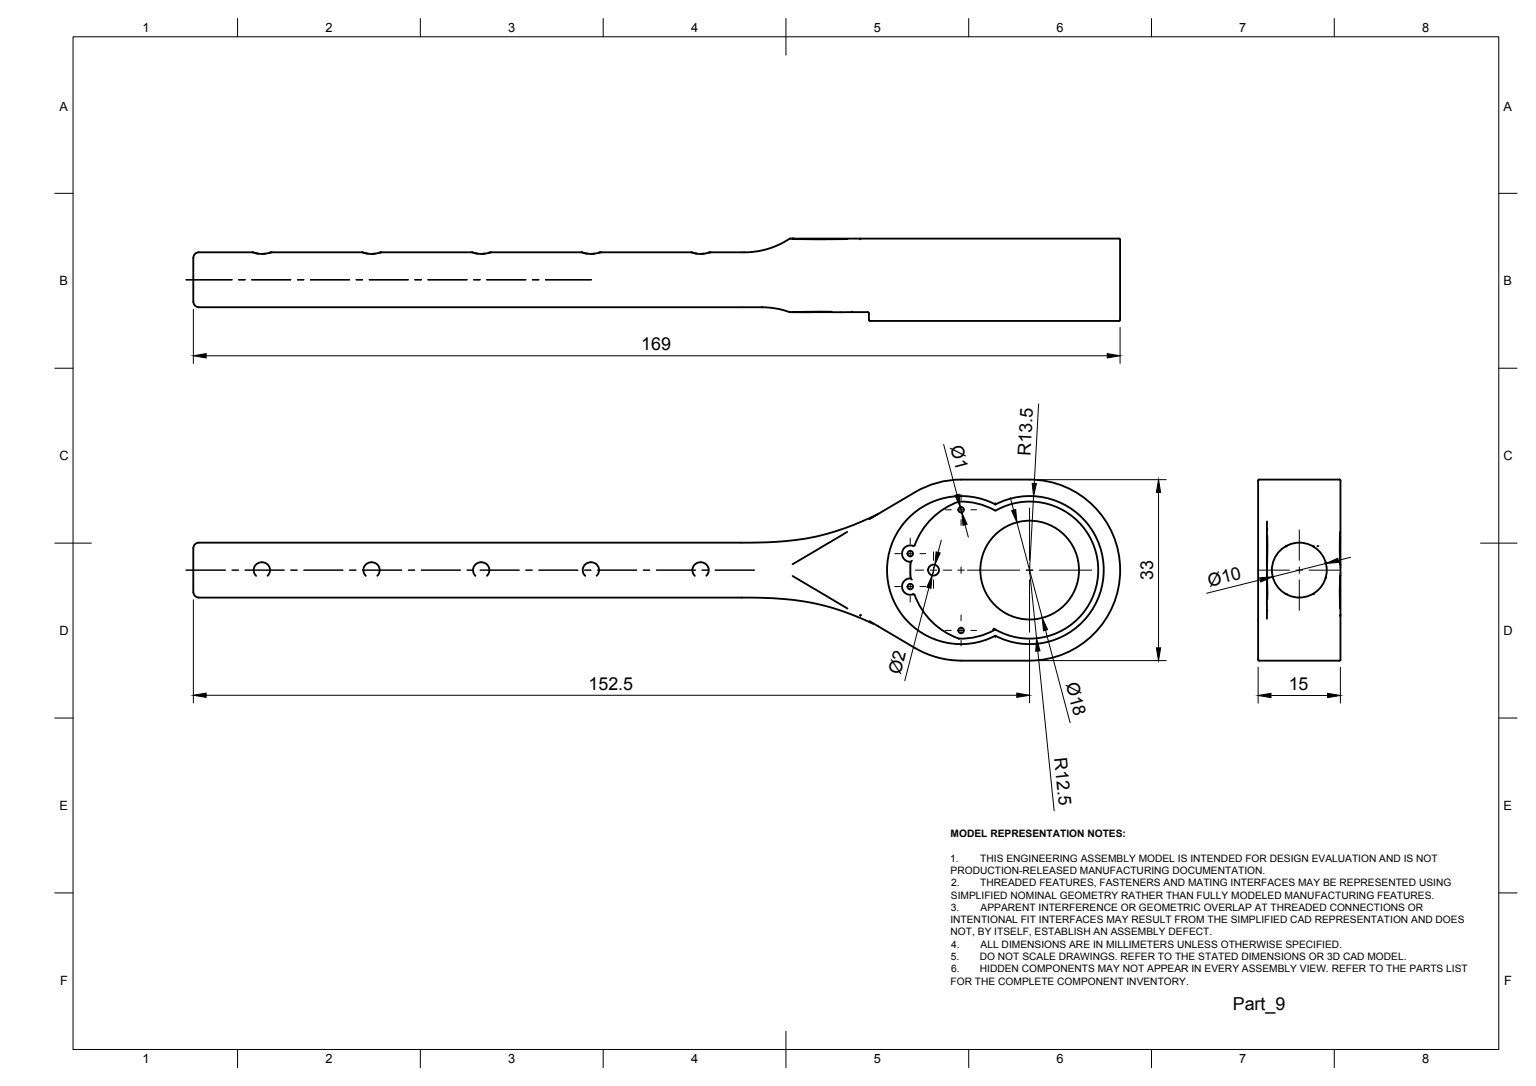
ISO-10303-21;
HEADER;
/* Generated by software containing ST-Developer
 * from STEP Tools, Inc. (www.steptools.com) 
 */

FILE_DESCRIPTION(
/* description */ ('STEP AP242 Edition 2'),
/* implementation_level */ '2;1');

FILE_NAME(
/* name */ 'Part_9.step',
/* time_stamp */ '2026-10-06T10:11:12-07:00',
/* author */ (''),
/* organization */ (''),
/* preprocessor_version */ 'ST-DEVELOPER v20.2',
/* originating_system */ 'Autodesk Translation Framework v15.15.0.0',
/* authorisation */ '');

FILE_SCHEMA (('AUTOMOTIVE_DESIGN { 1 0 10303 214 3 1 1 }'));
ENDSEC;

DATA;
#10=MECHANICAL_DESIGN_GEOMETRIC_PRESENTATION_REPRESENTATION('',(#1799),#54580);
#124=ELLIPSE('',#19386,0.00047049920898836,0.0004);
#125=ELLIPSE('',#19388,0.00047049920898836,0.0004);
#126=ELLIPSE('',#19445,0.000286242347628646,0.000206247332886668);
#127=ELLIPSE('',#19470,0.000318385781181688,0.0002);
#128=ELLIPSE('',#19492,0.000318385781181688,0.0002);
#129=ELLIPSE('',#19548,0.00200013961276074,0.00200000211919392);
#130=ELLIPSE('',#19569,0.00200131676890062,0.00200065811979615);
#160=SPHERICAL_SURFACE('',#19391,0.0015);
#161=SPHERICAL_SURFACE('',#19392,0.0015);
#162=SPHERICAL_SURFACE('',#19393,0.0015);
#163=SPHERICAL_SURFACE('',#19394,0.0015);
#164=SPHERICAL_SURFACE('',#19395,0.0015);
#165=SPHERICAL_SURFACE('',#19475,0.0002);
#166=SPHERICAL_SURFACE('',#19500,0.0002);
#167=SPHERICAL_SURFACE('',#19532,0.0002);
#168=SPHERICAL_SURFACE('',#19537,0.0002);
#169=SPHERICAL_SURFACE('',#19539,0.0002);
#283=TOROIDAL_SURFACE('',#19417,0.0723798046062635,0.0693846505577955);
#284=TOROIDAL_SURFACE('',#19418,0.0725493479148083,0.0695588361081736);
#285=TOROIDAL_SURFACE('',#19419,0.0729629625245639,0.0699799856940105);
#286=TOROIDAL_SURFACE('',#19420,0.0719744531392773,0.0689794249020661);
#287=TOROIDAL_SURFACE('',#19421,0.0127,0.0002);
#288=TOROIDAL_SURFACE('',#19424,0.0004,0.0002);
#289=TOROIDAL_SURFACE('',#19429,0.0134323601801219,0.0002);
#290=TOROIDAL_SURFACE('',#19430,0.0130323601801219,0.0002);
#291=TOROIDAL_SURFACE('',#19435,0.0004,0.0002);
#292=TOROIDAL_SURFACE('',#19437,0.0013,0.0002);
#293=TOROIDAL_SURFACE('',#19438,0.0130323601801219,0.0002);
#294=TOROIDAL_SURFACE('',#19439,0.0013,0.0002);
#295=TOROIDAL_SURFACE('',#19441,0.0004,0.0002);
#296=TOROIDAL_SURFACE('',#19444,0.0130323601801219,0.0002);
#297=TOROIDAL_SURFACE('',#19449,0.0134323601801219,0.0002);
#298=TOROIDAL_SURFACE('',#19451,0.0004,0.0002);
#299=TOROIDAL_SURFACE('',#19453,0.0127,0.0002);
#300=TOROIDAL_SURFACE('',#19456,0.0163,0.0002);
#301=TOROIDAL_SURFACE('',#19461,1.2311209928723,1.23094461923187);
#302=TOROIDAL_SURFACE('',#19471,0.00114036081014246,0.000200479570708582);
#303=TOROIDAL_SURFACE('',#19473,0.0163,0.0002);
#304=TOROIDAL_SURFACE('',#19479,1.19654575499128,1.19636811754444);
#305=TOROIDAL_SURFACE('',#19485,0.0023,0.0002);
#306=TOROIDAL_SURFACE('',#19487,0.0163,0.0002);
#307=TOROIDAL_SURFACE('',#19489,0.0027,0.0002);
#308=TOROIDAL_SURFACE('',#19503,0.0123,0.0002);
#309=TOROIDAL_SURFACE('',#19506,0.0092,0.0002);
#310=TOROIDAL_SURFACE('',#19512,0.0163,0.0002);
#311=TOROIDAL_SURFACE('',#19514,0.00109148741098655,0.000200226016163471);
#312=TOROIDAL_SURFACE('',#19519,0.0163,0.0002);
#313=TOROIDAL_SURFACE('',#19525,0.0163,0.0002);
#314=TOROIDAL_SURFACE('',#19526,0.0137,0.0002);
#315=TOROIDAL_SURFACE('',#19527,0.0137,0.0002);
#316=TOROIDAL_SURFACE('',#19528,0.0092,0.0002);
#317=TOROIDAL_SURFACE('',#19530,0.0012,0.0002);
#318=TOROIDAL_SURFACE('',#19534,0.0127,0.0002);
#319=TOROIDAL_SURFACE('',#19543,0.0123,0.0002);
#320=TOROIDAL_SURFACE('',#19546,0.0127,0.0002);
#321=TOROIDAL_SURFACE('',#19547,0.0021940391762114,0.00199286501744214);
#322=TOROIDAL_SURFACE('',#19575,0.004,0.001);
#337=B_SPLINE_SURFACE_WITH_KNOTS('',3,3,((#50042,#50043,#50044,#50045),
(#50046,#50047,#50048,#50049),(#50050,#50051,#50052,#50053),(#50054,#50055,
#50056,#50057),(#50058,#50059,#50060,#50061),(#50062,#50063,#50064,#50065),
(#50066,#50067,#50068,#50069)),.UNSPECIFIED.,.F.,.F.,.F.,(4,1,1,1,4),(4,
4),(0.581678330580955,0.66570223965942,0.749726148737884,0.833750057816349,
0.917773966894813),(0.,0.272096154167828),.UNSPECIFIED.);
#338=B_SPLINE_SURFACE_WITH_KNOTS('',3,3,((#50328,#50329,#50330,#50331),
(#50332,#50333,#50334,#50335),(#50336,#50337,#50338,#50339),(#50340,#50341,
#50342,#50343),(#50344,#50345,#50346,#50347),(#50348,#50349,#50350,#50351),
(#50352,#50353,#50354,#50355)),.UNSPECIFIED.,.F.,.F.,.F.,(4,1,1,1,4),(4,
4),(0.082398587787618,0.16607539724211,0.249752206696602,0.333429016151093,
0.417105825605585),(0.,0.340678729399104),.UNSPECIFIED.);
#339=B_SPLINE_SURFACE_WITH_KNOTS('',3,3,((#50620,#50621,#50622,#50623),
(#50624,#50625,#50626,#50627),(#50628,#50629,#50630,#50631),(#50632,#50633,
#50634,#50635),(#50636,#50637,#50638,#50639),(#50640,#50641,#50642,#50643),
(#50644,#50645,#50646,#50647),(#50648,#50649,#50650,#50651),(#50652,#50653,
#50654,#50655),(#50656,#50657,#50658,#50659)),.UNSPECIFIED.,.F.,.F.,.F.,
(4,3,1,1,1,4),(4,4),(0.88386669972742,0.917773966894813,0.93833047517111,
0.958886983447406,0.979443491723703,1.),(0.,1.),.UNSPECIFIED.);
#340=B_SPLINE_SURFACE_WITH_KNOTS('',3,3,((#50859,#50860,#50861,#50862),
(#50863,#50864,#50865,#50866),(#50867,#50868,#50869,#50870),(#50871,#50872,
#50873,#50874),(#50875,#50876,#50877,#50878),(#50879,#50880,#50881,#50882),
(#50883,#50884,#50885,#50886),(#50887,#50888,#50889,#50890),(#50891,#50892,
#50893,#50894),(#50895,#50896,#50897,#50898),(#50899,#50900,#50901,#50902),
(#50903,#50904,#50905,#50906),(#50907,#50908,#50909,#50910),(#50911,#50912,
#50913,#50914),(#50915,#50916,#50917,#50918),(#50919,#50920,#50921,#50922),
(#50923,#50924,#50925,#50926),(#50927,#50928,#50929,#50930)),
 .UNSPECIFIED.,.F.,.F.,.F.,(4,3,1,1,1,2,1,1,1,3,4),(4,4),(0.414454525410024,
0.417105825605585,0.437698866011632,0.45829190641768,0.478884946823728,
0.499477987229775,0.52002807306757,0.540578158905365,0.56112824474316,0.581678330580955,
0.616449456714453),(0.,1.),.UNSPECIFIED.);
#341=B_SPLINE_SURFACE_WITH_KNOTS('',3,3,((#51085,#51086,#51087,#51088),
(#51089,#51090,#51091,#51092),(#51093,#51094,#51095,#51096),(#51097,#51098,
#51099,#51100),(#51101,#51102,#51103,#51104),(#51105,#51106,#51107,#51108),
(#51109,#51110,#51111,#51112),(#51113,#51114,#51115,#51116),(#51117,#51118,
#51119,#51120),(#51121,#51122,#51123,#51124)),.UNSPECIFIED.,.F.,.F.,.F.,
(4,1,1,1,3,4),(4,4),(0.,0.0205996469469045,0.041199293893809,0.0617989408407135,
0.082398587787618,0.082892979314345),(0.,1.),.UNSPECIFIED.);
#342=B_SPLINE_SURFACE_WITH_KNOTS('',3,3,((#53343,#53344,#53345,#53346),
(#53347,#53348,#53349,#53350),(#53351,#53352,#53353,#53354),(#53355,#53356,
#53357,#53358),(#53359,#53360,#53361,#53362),(#53363,#53364,#53365,#53366),
(#53367,#53368,#53369,#53370),(#53371,#53372,#53373,#53374),(#53375,#53376,
#53377,#53378),(#53379,#53380,#53381,#53382),(#53383,#53384,#53385,#53386)),
 .UNSPECIFIED.,.F.,.F.,.F.,(4,1,1,1,1,1,1,1,4),(4,4),(-0.00100716856165045,
0.00254911418953192,0.00509822837906388,0.00764734256859584,0.0101964567581278,
0.0127455709476598,0.0152946851371917,0.0178437993267237,0.0213314374719094),
(0.,1.00749523383058),.UNSPECIFIED.);
#1362=B_SPLINE_CURVE_WITH_KNOTS('',3,(#49171,#49172,#49173,#49174,#49175,
#49176,#49177,#49178,#49179,#49180,#49181),.UNSPECIFIED.,.F.,.F.,(4,1,1,
1,1,1,1,1,4),(2.16840434497101E-19,0.00133638350122092,0.00267276700244183,
0.00400915050366275,0.00534553400488367,0.00668191750610458,0.0080183010073255,
0.00935468450854642,0.0106661079505718),.UNSPECIFIED.);
#1363=B_SPLINE_CURVE_WITH_KNOTS('',3,(#49187,#49188,#49189,#49190),
 .UNSPECIFIED.,.F.,.F.,(4,4),(0.0082109079468729,0.00936873648796082),
 .UNSPECIFIED.);
#1364=B_SPLINE_CURVE_WITH_KNOTS('',3,(#49192,#49193,#49194,#49195,#49196),
 .UNSPECIFIED.,.F.,.F.,(4,1,4),(0.00704598836791066,0.00819764442696572,
0.0082109079468729),.UNSPECIFIED.);
#1365=B_SPLINE_CURVE_WITH_KNOTS('',3,(#49198,#49199,#49200,#49201,#49202),
 .UNSPECIFIED.,.F.,.F.,(4,1,4),(0.00585546030497552,0.00702655236597062,
0.00704598836791066),.UNSPECIFIED.);
#1366=B_SPLINE_CURVE_WITH_KNOTS('',3,(#49204,#49205,#49206,#49207,#49208),
 .UNSPECIFIED.,.F.,.F.,(4,1,4),(0.00352617550117164,0.00468436824398041,
0.00585546030497552),.UNSPECIFIED.);
#1367=B_SPLINE_CURVE_WITH_KNOTS('',3,(#49210,#49211,#49212,#49213,#49214),
 .UNSPECIFIED.,.F.,.F.,(4,1,4),(0.00236041305988056,0.00351327618298531,
0.00352617550117164),.UNSPECIFIED.);
#1368=B_SPLINE_CURVE_WITH_KNOTS('',3,(#49216,#49217,#49218,#49219,#49220),
 .UNSPECIFIED.,.F.,.F.,(4,1,4),(0.0011710920609951,0.00234218412199021,
0.00236041305988056),.UNSPECIFIED.);
#1369=B_SPLINE_CURVE_WITH_KNOTS('',3,(#49221,#49222,#49223,#49224),
 .UNSPECIFIED.,.F.,.F.,(4,4),(2.22095063237474E-5,0.0011710920609951),
 .UNSPECIFIED.);
#1370=B_SPLINE_CURVE_WITH_KNOTS('',3,(#49264,#49265,#49266,#49267,#49268,
#49269,#49270,#49271,#49272,#49273,#49274),.UNSPECIFIED.,.F.,.F.,(4,1,1,
1,1,1,1,1,4),(2.16840434497101E-19,0.00133638350122092,0.00267276700244184,
0.00400915050366276,0.00534553400488369,0.00668191750610461,0.00801830100732553,
0.00935468450854645,0.0106661079505719),.UNSPECIFIED.);
#1371=B_SPLINE_CURVE_WITH_KNOTS('',3,(#49280,#49281,#49282,#49283),
 .UNSPECIFIED.,.F.,.F.,(4,4),(0.00821090794687196,0.00936873648796082),
 .UNSPECIFIED.);
#1372=B_SPLINE_CURVE_WITH_KNOTS('',3,(#49285,#49286,#49287,#49288,#49289),
 .UNSPECIFIED.,.F.,.F.,(4,1,4),(0.00704598836790975,0.00819764442696572,
0.00821090794687196),.UNSPECIFIED.);
#1373=B_SPLINE_CURVE_WITH_KNOTS('',3,(#49291,#49292,#49293,#49294,#49295),
 .UNSPECIFIED.,.F.,.F.,(4,1,4),(0.00585546030497551,0.00702655236597062,
0.00704598836790975),.UNSPECIFIED.);
#1374=B_SPLINE_CURVE_WITH_KNOTS('',3,(#49297,#49298,#49299,#49300,#49301),
 .UNSPECIFIED.,.F.,.F.,(4,1,4),(0.00352617550117226,0.00468436824398041,
0.00585546030497551),.UNSPECIFIED.);
#1375=B_SPLINE_CURVE_WITH_KNOTS('',3,(#49303,#49304,#49305,#49306,#49307),
 .UNSPECIFIED.,.F.,.F.,(4,1,4),(0.00236041305988015,0.00351327618298531,
0.00352617550117226),.UNSPECIFIED.);
#1376=B_SPLINE_CURVE_WITH_KNOTS('',3,(#49309,#49310,#49311,#49312,#49313),
 .UNSPECIFIED.,.F.,.F.,(4,1,4),(0.0011710920609951,0.00234218412199021,
0.00236041305988015),.UNSPECIFIED.);
#1377=B_SPLINE_CURVE_WITH_KNOTS('',3,(#49314,#49315,#49316,#49317),
 .UNSPECIFIED.,.F.,.F.,(4,4),(2.22095063236846E-5,0.0011710920609951),
 .UNSPECIFIED.);
#1378=B_SPLINE_CURVE_WITH_KNOTS('',3,(#49357,#49358,#49359,#49360,#49361,
#49362,#49363,#49364,#49365,#49366,#49367),.UNSPECIFIED.,.F.,.F.,(4,1,1,
1,1,1,1,1,4),(2.16840434497101E-19,0.00133638350122092,0.00267276700244184,
0.00400915050366277,0.00534553400488369,0.00668191750610461,0.00801830100732553,
0.00935468450854646,0.0106661079505718),.UNSPECIFIED.);
#1379=B_SPLINE_CURVE_WITH_KNOTS('',3,(#49373,#49374,#49375,#49376),
 .UNSPECIFIED.,.F.,.F.,(4,4),(0.00821090794687294,0.00936873648796081),
 .UNSPECIFIED.);
#1380=B_SPLINE_CURVE_WITH_KNOTS('',3,(#49378,#49379,#49380,#49381,#49382),
 .UNSPECIFIED.,.F.,.F.,(4,1,4),(0.00704598836791145,0.00819764442696571,
0.00821090794687294),.UNSPECIFIED.);
#1381=B_SPLINE_CURVE_WITH_KNOTS('',3,(#49384,#49385,#49386,#49387,#49388),
 .UNSPECIFIED.,.F.,.F.,(4,1,4),(0.00585546030497551,0.00702655236597061,
0.00704598836791145),.UNSPECIFIED.);
#1382=B_SPLINE_CURVE_WITH_KNOTS('',3,(#49390,#49391,#49392,#49393,#49394),
 .UNSPECIFIED.,.F.,.F.,(4,1,4),(0.00352617550117169,0.00468436824398041,
0.00585546030497551),.UNSPECIFIED.);
#1383=B_SPLINE_CURVE_WITH_KNOTS('',3,(#49396,#49397,#49398,#49399,#49400),
 .UNSPECIFIED.,.F.,.F.,(4,1,4),(0.00236041305987884,0.00351327618298531,
0.00352617550117169),.UNSPECIFIED.);
#1384=B_SPLINE_CURVE_WITH_KNOTS('',3,(#49402,#49403,#49404,#49405,#49406),
 .UNSPECIFIED.,.F.,.F.,(4,1,4),(0.0011710920609951,0.0023421841219902,0.00236041305987884),
 .UNSPECIFIED.);
#1385=B_SPLINE_CURVE_WITH_KNOTS('',3,(#49407,#49408,#49409,#49410),
 .UNSPECIFIED.,.F.,.F.,(4,4),(2.2209506323702E-5,0.0011710920609951),
 .UNSPECIFIED.);
#1386=B_SPLINE_CURVE_WITH_KNOTS('',3,(#49450,#49451,#49452,#49453,#49454,
#49455,#49456,#49457,#49458,#49459,#49460),.UNSPECIFIED.,.F.,.F.,(4,1,1,
1,1,1,1,1,4),(2.16840434497101E-19,0.00133638350122092,0.00267276700244185,
0.00400915050366277,0.0053455340048837,0.00668191750610462,0.00801830100732555,
0.00935468450854647,0.0106661079505723),.UNSPECIFIED.);
#1387=B_SPLINE_CURVE_WITH_KNOTS('',3,(#49466,#49467,#49468,#49469),
 .UNSPECIFIED.,.F.,.F.,(4,4),(0.00821090794688191,0.00936873648796083),
 .UNSPECIFIED.);
#1388=B_SPLINE_CURVE_WITH_KNOTS('',3,(#49471,#49472,#49473,#49474,#49475),
 .UNSPECIFIED.,.F.,.F.,(4,1,4),(0.00704598836790659,0.00819764442696573,
0.00821090794688191),.UNSPECIFIED.);
#1389=B_SPLINE_CURVE_WITH_KNOTS('',3,(#49477,#49478,#49479,#49480,#49481),
 .UNSPECIFIED.,.F.,.F.,(4,1,4),(0.00585546030497552,0.00702655236597062,
0.00704598836790659),.UNSPECIFIED.);
#1390=B_SPLINE_CURVE_WITH_KNOTS('',3,(#49483,#49484,#49485,#49486,#49487),
 .UNSPECIFIED.,.F.,.F.,(4,1,4),(0.00352617550117701,0.00468436824398042,
0.00585546030497552),.UNSPECIFIED.);
#1391=B_SPLINE_CURVE_WITH_KNOTS('',3,(#49489,#49490,#49491,#49492,#49493),
 .UNSPECIFIED.,.F.,.F.,(4,1,4),(0.00236041305988171,0.00351327618298531,
0.00352617550117701),.UNSPECIFIED.);
#1392=B_SPLINE_CURVE_WITH_KNOTS('',3,(#49495,#49496,#49497,#49498,#49499),
 .UNSPECIFIED.,.F.,.F.,(4,1,4),(0.0011710920609951,0.00234218412199021,
0.00236041305988171),.UNSPECIFIED.);
#1393=B_SPLINE_CURVE_WITH_KNOTS('',3,(#49500,#49501,#49502,#49503),
 .UNSPECIFIED.,.F.,.F.,(4,4),(2.22095063237639E-5,0.0011710920609951),
 .UNSPECIFIED.);
#1394=B_SPLINE_CURVE_WITH_KNOTS('',3,(#49543,#49544,#49545,#49546,#49547,
#49548,#49549,#49550,#49551,#49552,#49553),.UNSPECIFIED.,.F.,.F.,(4,1,1,
1,1,1,1,1,4),(2.16840434497101E-19,0.00133638350122091,0.00267276700244182,
0.00400915050366274,0.00534553400488365,0.00668191750610456,0.00801830100732547,
0.00935468450854638,0.0106661079505722),.UNSPECIFIED.);
#1395=B_SPLINE_CURVE_WITH_KNOTS('',3,(#49559,#49560,#49561,#49562),
 .UNSPECIFIED.,.F.,.F.,(4,4),(0.00821090794688314,0.00936873648796083),
 .UNSPECIFIED.);
#1396=B_SPLINE_CURVE_WITH_KNOTS('',3,(#49564,#49565,#49566,#49567,#49568),
 .UNSPECIFIED.,.F.,.F.,(4,1,4),(0.00704598836790498,0.00819764442696573,
0.00821090794688314),.UNSPECIFIED.);
#1397=B_SPLINE_CURVE_WITH_KNOTS('',3,(#49570,#49571,#49572,#49573,#49574),
 .UNSPECIFIED.,.F.,.F.,(4,1,4),(0.00585546030497552,0.00702655236597062,
0.00704598836790498),.UNSPECIFIED.);
#1398=B_SPLINE_CURVE_WITH_KNOTS('',3,(#49576,#49577,#49578,#49579,#49580),
 .UNSPECIFIED.,.F.,.F.,(4,1,4),(0.0035261755011782,0.00468436824398041,
0.00585546030497552),.UNSPECIFIED.);
#1399=B_SPLINE_CURVE_WITH_KNOTS('',3,(#49582,#49583,#49584,#49585,#49586),
 .UNSPECIFIED.,.F.,.F.,(4,1,4),(0.00236041305988064,0.00351327618298531,
0.0035261755011782),.UNSPECIFIED.);
#1400=B_SPLINE_CURVE_WITH_KNOTS('',3,(#49588,#49589,#49590,#49591,#49592),
 .UNSPECIFIED.,.F.,.F.,(4,1,4),(0.0011710920609951,0.00234218412199021,
0.00236041305988064),.UNSPECIFIED.);
#1401=B_SPLINE_CURVE_WITH_KNOTS('',3,(#49593,#49594,#49595,#49596),
 .UNSPECIFIED.,.F.,.F.,(4,4),(2.2209506323727E-5,0.0011710920609951),
 .UNSPECIFIED.);
#1402=B_SPLINE_CURVE_WITH_KNOTS('',3,(#49600,#49601,#49602,#49603),
 .UNSPECIFIED.,.F.,.F.,(4,4),(0.,0.000682262674512534),.UNSPECIFIED.);
#1403=B_SPLINE_CURVE_WITH_KNOTS('',3,(#49668,#49669,#49670,#49671,#49672,
#49673),.UNSPECIFIED.,.F.,.F.,(4,2,4),(-0.101895978906481,-0.0984710269726971,
-0.0896897186466305),.UNSPECIFIED.);
#1404=B_SPLINE_CURVE_WITH_KNOTS('',3,(#49680,#49681,#49682,#49683,#49684,
#49685,#49686,#49687,#49688,#49689),.UNSPECIFIED.,.F.,.F.,(4,2,2,2,4),(0.00701311257563557,
0.010982820742087,0.0253526872842843,0.0698643291505208,0.0772205186033042),
 .UNSPECIFIED.);
#1405=B_SPLINE_CURVE_WITH_KNOTS('',3,(#49702,#49703,#49704,#49705,#49706,
#49707,#49708,#49709,#49710,#49711,#49712,#49713,#49714),.UNSPECIFIED.,
 .F.,.F.,(4,3,3,3,4),(0.0824582419012307,0.166224116038678,0.249986773069777,
0.333749430179514,0.417515304238324),.UNSPECIFIED.);
#1406=B_SPLINE_CURVE_WITH_KNOTS('',3,(#49720,#49721,#49722,#49723,#49724,
#49725,#49726,#49727,#49728,#49729,#49730,#49731,#49732),.UNSPECIFIED.,
 .F.,.F.,(4,3,3,3,4),(0.582140268332509,0.666078166051184,0.750012831472539,
0.833947496910044,0.91788539461257),.UNSPECIFIED.);
#1407=B_SPLINE_CURVE_WITH_KNOTS('',3,(#49741,#49742,#49743,#49744),
 .UNSPECIFIED.,.F.,.F.,(4,4),(0.0106661079505722,0.0106910680097673),
 .UNSPECIFIED.);
#1408=B_SPLINE_CURVE_WITH_KNOTS('',3,(#49745,#49746,#49747,#49748),
 .UNSPECIFIED.,.F.,.F.,(4,4),(0.0106661079505723,0.0106910680097674),
 .UNSPECIFIED.);
#1409=B_SPLINE_CURVE_WITH_KNOTS('',3,(#49749,#49750,#49751,#49752),
 .UNSPECIFIED.,.F.,.F.,(4,4),(0.0106661079505718,0.0106910680097674),
 .UNSPECIFIED.);
#1410=B_SPLINE_CURVE_WITH_KNOTS('',3,(#49753,#49754,#49755,#49756),
 .UNSPECIFIED.,.F.,.F.,(4,4),(0.0106661079505719,0.0106910680097674),
 .UNSPECIFIED.);
#1411=B_SPLINE_CURVE_WITH_KNOTS('',3,(#49757,#49758,#49759,#49760),
 .UNSPECIFIED.,.F.,.F.,(4,4),(0.0106661079505718,0.0106910680097673),
 .UNSPECIFIED.);
#1412=B_SPLINE_CURVE_WITH_KNOTS('',3,(#49824,#49825,#49826,#49827,#49828,
#49829,#49830),.UNSPECIFIED.,.F.,.F.,(4,3,4),(2.16840434497101E-19,0.00581319522920539,
0.0116263904584108),.UNSPECIFIED.);
#1413=B_SPLINE_CURVE_WITH_KNOTS('',3,(#49832,#49833,#49834,#49835),
 .UNSPECIFIED.,.F.,.F.,(4,4),(2.79715755706988E-17,0.00267897349074099),
 .UNSPECIFIED.);
#1414=B_SPLINE_CURVE_WITH_KNOTS('',3,(#49851,#49852,#49853,#49854),
 .UNSPECIFIED.,.F.,.F.,(4,4),(3.43963882861591E-14,0.0026798705859963),
 .UNSPECIFIED.);
#1415=B_SPLINE_CURVE_WITH_KNOTS('',3,(#49856,#49857,#49858,#49859,#49860,
#49861,#49862),.UNSPECIFIED.,.F.,.F.,(4,3,4),(0.0153783179950603,0.0211672261179413,
0.0269561342408223),.UNSPECIFIED.);
#1416=B_SPLINE_CURVE_WITH_KNOTS('',3,(#49863,#49864,#49865,#49866,#49867,
#49868,#49869,#49870,#49871,#49872,#49873,#49874,#49875),.UNSPECIFIED.,
 .F.,.F.,(4,3,3,3,4),(1.62471150819444E-9,0.371962494639839,0.5,0.868119627457051,
0.999999997610495),.UNSPECIFIED.);
#1417=B_SPLINE_CURVE_WITH_KNOTS('',3,(#49934,#49935,#49936,#49937,#49938,
#49939,#49940,#49941,#49942,#49943,#49944,#49945,#49946,#49947,#49948,#49949),
 .UNSPECIFIED.,.F.,.F.,(4,3,3,3,3,4),(1.63653485417008E-17,0.000871734875690096,
0.00174346975138018,0.00261520462707026,0.0030510720649153,0.00348693950276033),
 .UNSPECIFIED.);
#1418=B_SPLINE_CURVE_WITH_KNOTS('',3,(#49951,#49952,#49953,#49954,#49955,
#49956,#49957,#49958,#49959,#49960,#49961,#49962,#49963,#49964,#49965,#49966),
 .UNSPECIFIED.,.F.,.F.,(4,3,3,3,3,4),(0.,0.25,0.375,0.5,0.75,1.),
 .UNSPECIFIED.);
#1419=B_SPLINE_CURVE_WITH_KNOTS('',3,(#49970,#49971,#49972,#49973,#49974,
#49975,#49976,#49977,#49978,#49979,#49980,#49981,#49982),.UNSPECIFIED.,
 .F.,.F.,(4,3,3,3,4),(3.26962013452912E-17,0.000593256852872857,0.00118651370574568,
0.00177977055861851,0.00237302741149133),.UNSPECIFIED.);
#1420=B_SPLINE_CURVE_WITH_KNOTS('',3,(#49993,#49994,#49995,#49996,#49997,
#49998,#49999,#50000,#50001,#50002,#50003,#50004,#50005),.UNSPECIFIED.,
 .F.,.F.,(4,3,3,3,4),(1.56949960400744E-16,0.000586676321783765,0.00117335264356737,
0.00176002896535098,0.00234670528713459),.UNSPECIFIED.);
#1421=B_SPLINE_CURVE_WITH_KNOTS('',3,(#50009,#50010,#50011,#50012),
 .UNSPECIFIED.,.F.,.F.,(4,4),(0.,1.),.UNSPECIFIED.);
#1422=B_SPLINE_CURVE_WITH_KNOTS('',3,(#50014,#50015,#50016,#50017),
 .UNSPECIFIED.,.F.,.F.,(4,4),(0.,1.),.UNSPECIFIED.);
#1423=B_SPLINE_CURVE_WITH_KNOTS('',3,(#50019,#50020,#50021,#50022,#50023,
#50024,#50025,#50026,#50027,#50028,#50029,#50030,#50031,#50032,#50033,#50034),
 .UNSPECIFIED.,.F.,.F.,(4,3,3,3,3,4),(1.23884035470014E-17,0.000436227682635904,
0.000872455365271796,0.00174491073054358,0.00261736609581536,0.00348982146108715),
 .UNSPECIFIED.);
#1424=B_SPLINE_CURVE_WITH_KNOTS('',3,(#50071,#50072,#50073,#50074,#50075,
#50076,#50077,#50078,#50079,#50080),.UNSPECIFIED.,.F.,.F.,(4,3,3,4),(0.,
0.250198742533901,0.484142189377901,0.72625720196945),.UNSPECIFIED.);
#1425=B_SPLINE_CURVE_WITH_KNOTS('',3,(#50082,#50083,#50084,#50085,#50086,
#50087,#50088,#50089,#50090,#50091,#50092,#50093,#50094,#50095,#50096,#50097,
#50098,#50099,#50100,#50101,#50102,#50103,#50104,#50105,#50106,#50107,#50108,
#50109,#50110,#50111,#50112,#50113,#50114,#50115,#50116,#50117,#50118,#50119,
#50120,#50121,#50122,#50123,#50124,#50125,#50126,#50127,#50128,#50129,#50130,
#50131,#50132,#50133,#50134,#50135,#50136),.UNSPECIFIED.,.F.,.F.,(4,3,3,
3,3,3,3,3,3,3,3,3,3,3,3,3,3,3,4),(2.6220077343514E-7,0.0203152518413343,
0.134046967430369,0.239869415550571,0.25,0.339303542480863,0.375,0.5,0.523390970218302,
0.625,0.6875,0.69519800169401,0.71875,0.75,0.78125,0.8125,0.875,0.884458267348107,
1.),.UNSPECIFIED.);
#1426=B_SPLINE_CURVE_WITH_KNOTS('',3,(#50138,#50139,#50140,#50141,#50142,
#50143,#50144,#50145,#50146,#50147,#50148,#50149,#50150,#50151,#50152,#50153,
#50154,#50155,#50156,#50157,#50158,#50159,#50160,#50161,#50162,#50163,#50164,
#50165,#50166,#50167,#50168,#50169,#50170,#50171,#50172,#50173,#50174,#50175,
#50176,#50177,#50178,#50179,#50180,#50181,#50182,#50183,#50184,#50185,#50186,
#50187,#50188,#50189,#50190,#50191,#50192,#50193,#50194,#50195,#50196,#50197,
#50198,#50199,#50200,#50201,#50202,#50203,#50204),.UNSPECIFIED.,.F.,.F.,
(4,3,3,3,3,3,3,3,3,3,3,3,3,3,3,3,3,3,3,3,3,3,4),(0.,0.0625,0.125,0.182156208275604,
0.1875,0.25,0.31138954419103,0.3125,0.375,0.41421262630946,0.4375,0.5,0.5625,
0.586017101931546,0.625,0.6875,0.688684714649581,0.75,0.8125,0.81792114283053,
0.875,0.9375,1.),.UNSPECIFIED.);
#1427=B_SPLINE_CURVE_WITH_KNOTS('',3,(#50206,#50207,#50208,#50209,#50210,
#50211,#50212,#50213,#50214,#50215,#50216,#50217,#50218,#50219,#50220,#50221,
#50222,#50223,#50224,#50225,#50226,#50227,#50228,#50229,#50230,#50231,#50232,
#50233,#50234,#50235,#50236,#50237,#50238,#50239,#50240,#50241,#50242,#50243,
#50244,#50245,#50246,#50247,#50248,#50249,#50250,#50251,#50252,#50253,#50254,
#50255,#50256,#50257),.UNSPECIFIED.,.F.,.F.,(4,3,3,3,3,3,3,3,3,3,3,3,3,
3,3,3,3,4),(0.,0.113955744298881,0.125,0.1875,0.21875,0.25,0.28125,0.30198702723121,
0.3125,0.375,0.471780754133228,0.5,0.625,0.654220290439613,0.75,0.856955738520236,
0.969024551611296,0.999999731075503),.UNSPECIFIED.);
#1428=B_SPLINE_CURVE_WITH_KNOTS('',3,(#50258,#50259,#50260,#50261,#50262,
#50263,#50264,#50265,#50266,#50267,#50268,#50269,#50270,#50271,#50272,#50273,
#50274,#50275,#50276,#50277,#50278,#50279,#50280,#50281,#50282,#50283,#50284,
#50285,#50286,#50287,#50288,#50289,#50290,#50291,#50292,#50293,#50294,#50295,
#50296,#50297,#50298,#50299,#50300,#50301,#50302,#50303,#50304,#50305,#50306,
#50307,#50308,#50309,#50310,#50311,#50312,#50313,#50314,#50315,#50316,#50317,
#50318,#50319,#50320,#50321,#50322,#50323,#50324,#50325,#50326,#50327),
 .UNSPECIFIED.,.F.,.F.,(4,3,3,3,3,3,3,3,3,3,3,3,3,3,3,3,3,3,3,3,3,3,3,4),
(0.,0.0625,0.09375,0.109375,0.1171875,0.125,0.140625,0.15625,0.1875,0.25,
0.3125,0.375,0.4375,0.5,0.5625,0.625,0.65625,0.6875,0.703125,0.71875,0.75,
0.8125,0.875,1.),.UNSPECIFIED.);
#1429=B_SPLINE_CURVE_WITH_KNOTS('',3,(#50358,#50359,#50360,#50361,#50362,
#50363,#50364,#50365,#50366,#50367,#50368,#50369,#50370,#50371,#50372,#50373,
#50374,#50375,#50376,#50377,#50378,#50379,#50380,#50381,#50382,#50383,#50384,
#50385,#50386,#50387,#50388,#50389,#50390,#50391,#50392,#50393,#50394,#50395,
#50396,#50397,#50398,#50399,#50400,#50401,#50402,#50403,#50404,#50405,#50406,
#50407,#50408,#50409,#50410,#50411,#50412,#50413,#50414,#50415,#50416,#50417,
#50418),.UNSPECIFIED.,.F.,.F.,(4,3,3,3,3,3,3,3,3,3,3,3,3,3,3,3,3,3,3,3,
4),(0.,0.125,0.18211780806116,0.21875,0.232943528841739,0.25,0.28125,0.3125,
0.32477251801541,0.375,0.4375,0.451086136346817,0.5,0.5625,0.589820371942222,
0.625,0.740436596594459,0.75,0.823581534574207,0.912738301505326,0.999999265653549),
 .UNSPECIFIED.);
#1430=B_SPLINE_CURVE_WITH_KNOTS('',3,(#50419,#50420,#50421,#50422,#50423,
#50424,#50425,#50426,#50427,#50428,#50429,#50430,#50431,#50432,#50433,#50434,
#50435,#50436,#50437,#50438,#50439,#50440,#50441,#50442,#50443,#50444,#50445,
#50446,#50447,#50448,#50449,#50450,#50451,#50452,#50453,#50454,#50455,#50456,
#50457,#50458,#50459,#50460,#50461,#50462,#50463,#50464,#50465,#50466,#50467,
#50468,#50469,#50470),.UNSPECIFIED.,.F.,.F.,(4,3,3,3,3,3,3,3,3,3,3,3,3,
3,3,3,3,4),(1.08343486081908E-7,0.125,0.1875,0.25,0.375,0.4375,0.46875,
0.5,0.53125,0.5625,0.625,0.6875,0.75,0.8125,0.875,0.90625,0.9375,1.),
 .UNSPECIFIED.);
#1431=B_SPLINE_CURVE_WITH_KNOTS('',3,(#50472,#50473,#50474,#50475,#50476,
#50477,#50478,#50479,#50480,#50481,#50482,#50483,#50484,#50485,#50486,#50487,
#50488,#50489,#50490,#50491,#50492,#50493,#50494,#50495,#50496,#50497,#50498,
#50499,#50500,#50501,#50502,#50503,#50504,#50505,#50506,#50507,#50508),
 .UNSPECIFIED.,.F.,.F.,(4,3,3,3,3,3,3,3,3,3,3,3,4),(0.,0.0625,0.125,0.1875,
0.25,0.375,0.5,0.625,0.75,0.78125,0.8125,0.875,0.999999860772477),
 .UNSPECIFIED.);
#1432=B_SPLINE_CURVE_WITH_KNOTS('',3,(#50510,#50511,#50512,#50513,#50514,
#50515,#50516,#50517,#50518,#50519,#50520,#50521,#50522,#50523,#50524,#50525,
#50526,#50527,#50528,#50529,#50530,#50531,#50532,#50533,#50534,#50535,#50536,
#50537,#50538,#50539,#50540,#50541,#50542,#50543,#50544,#50545,#50546,#50547,
#50548,#50549,#50550,#50551,#50552,#50553,#50554,#50555,#50556,#50557,#50558,
#50559,#50560,#50561,#50562,#50563,#50564,#50565,#50566,#50567,#50568,#50569,
#50570),.UNSPECIFIED.,.F.,.F.,(4,3,3,3,3,3,3,3,3,3,3,3,3,3,3,3,3,3,3,3,
4),(7.54076708606675E-7,0.0890838043400427,0.177519647918873,0.25,0.260152278755688,
0.375,0.410146430846909,0.4375,0.5,0.548806008922445,0.5625,0.625,0.675295564779425,
0.6875,0.71875,0.75,0.768236511403328,0.78125,0.829706236970379,0.875,1.),
 .UNSPECIFIED.);
#1433=B_SPLINE_CURVE_WITH_KNOTS('',3,(#50571,#50572,#50573,#50574,#50575,
#50576,#50577,#50578,#50579,#50580,#50581,#50582,#50583,#50584,#50585,#50586,
#50587,#50588,#50589,#50590,#50591,#50592,#50593,#50594,#50595,#50596,#50597,
#50598,#50599,#50600,#50601,#50602,#50603,#50604,#50605,#50606,#50607,#50608,
#50609,#50610,#50611,#50612,#50613,#50614,#50615,#50616,#50617,#50618,#50619),
 .UNSPECIFIED.,.F.,.F.,(4,3,3,3,3,3,3,3,3,3,3,3,3,3,3,3,4),(0.,0.125,0.1875,
0.25,0.299171599130771,0.3125,0.375,0.405133032227414,0.5,0.597278855307766,
0.625,0.6875,0.702732497560042,0.75,0.8125,0.875,1.),.UNSPECIFIED.);
#1434=B_SPLINE_CURVE_WITH_KNOTS('',3,(#50662,#50663,#50664,#50665),
 .UNSPECIFIED.,.F.,.F.,(4,4),(4.48352082164622E-10,0.999999999778094),
 .UNSPECIFIED.);
#1435=B_SPLINE_CURVE_WITH_KNOTS('',3,(#50669,#50670,#50671,#50672,#50673,
#50674,#50675,#50676,#50677,#50678,#50679,#50680,#50681,#50682,#50683,#50684,
#50685,#50686,#50687,#50688,#50689,#50690,#50691,#50692,#50693,#50694,#50695,
#50696,#50697,#50698,#50699,#50700,#50701,#50702,#50703,#50704,#50705,#50706,
#50707,#50708,#50709,#50710,#50711,#50712,#50713,#50714,#50715,#50716,#50717,
#50718,#50719,#50720,#50721,#50722,#50723,#50724,#50725,#50726,#50727,#50728,
#50729,#50730,#50731,#50732,#50733,#50734,#50735,#50736,#50737,#50738,#50739,
#50740,#50741,#50742,#50743,#50744,#50745,#50746,#50747,#50748,#50749,#50750,
#50751,#50752,#50753,#50754,#50755,#50756,#50757,#50758,#50759,#50760,#50761,
#50762,#50763,#50764,#50765,#50766,#50767,#50768,#50769,#50770,#50771,#50772,
#50773,#50774,#50775,#50776,#50777,#50778,#50779,#50780,#50781,#50782,#50783,
#50784,#50785,#50786,#50787,#50788,#50789,#50790,#50791,#50792,#50793,#50794,
#50795),.UNSPECIFIED.,.F.,.F.,(4,3,3,3,3,3,3,3,3,3,3,3,3,3,3,3,3,3,3,3,
3,3,3,3,3,3,3,3,3,3,3,3,3,3,3,3,3,3,3,3,3,3,4),(0.,0.0458053754614711,0.0750691510926553,
0.10248161995056,0.135574456705558,0.183221501845885,0.215541126384413,
0.235200596896411,0.25121949529829,0.270280464799092,0.297803561834966,
0.3125,0.34375,0.375,0.389701511535224,0.40625,0.445507570744879,0.477590011279423,
0.506318202949039,0.54013120645178,0.5625,0.585957017411357,0.625,0.6875,
0.703125,0.71875,0.75,0.780133441203814,0.78125,0.796875,0.813355261544154,
0.831836748639714,0.84375,0.873025477612267,0.875,0.890625,0.912254662027643,
0.926757684009806,0.940434508371303,0.953125,0.964809427833706,0.96875,
0.999999999954988),.UNSPECIFIED.);
#1436=B_SPLINE_CURVE_WITH_KNOTS('',3,(#50797,#50798,#50799,#50800,#50801,
#50802,#50803,#50804,#50805,#50806,#50807,#50808),.UNSPECIFIED.,.F.,.F.,
(4,1,1,1,1,1,1,1,1,4),(0.,0.125,0.25,0.375,0.5,0.5625,0.625,0.75,0.875,
1.),.UNSPECIFIED.);
#1437=B_SPLINE_CURVE_WITH_KNOTS('',3,(#50809,#50810,#50811,#50812,#50813,
#50814,#50815,#50816,#50817,#50818,#50819,#50820,#50821,#50822,#50823,#50824,
#50825,#50826,#50827,#50828,#50829,#50830,#50831,#50832,#50833,#50834,#50835,
#50836,#50837,#50838,#50839,#50840,#50841,#50842,#50843,#50844,#50845,#50846,
#50847,#50848,#50849,#50850,#50851,#50852,#50853,#50854),.UNSPECIFIED.,
 .F.,.F.,(4,3,3,3,3,3,3,3,3,3,3,3,3,3,3,4),(0.,0.0625,0.125,0.15625,0.1875,
0.25,0.375,0.4375,0.5,0.5625,0.625,0.6875,0.75,0.875,0.977913764805899,
1.),.UNSPECIFIED.);
#1438=B_SPLINE_CURVE_WITH_KNOTS('',3,(#50855,#50856,#50857,#50858),
 .UNSPECIFIED.,.F.,.F.,(4,4),(0.,0.997240928837636),.UNSPECIFIED.);
#1439=B_SPLINE_CURVE_WITH_KNOTS('',3,(#50935,#50936,#50937,#50938,#50939,
#50940,#50941,#50942,#50943,#50944,#50945,#50946,#50947,#50948,#50949,#50950,
#50951,#50952,#50953,#50954,#50955,#50956,#50957,#50958,#50959),
 .UNSPECIFIED.,.F.,.F.,(4,3,3,3,3,3,3,3,4),(2.03487242492536E-9,0.0258251891945382,
0.164170751422891,0.302802438327866,0.441718638276399,0.580627042706572,
0.719815414030138,0.859281996108356,1.),.UNSPECIFIED.);
#1440=B_SPLINE_CURVE_WITH_KNOTS('',3,(#50961,#50962,#50963,#50964,#50965,
#50966,#50967,#50968,#50969),.UNSPECIFIED.,.F.,.F.,(4,1,1,1,1,1,4),(7.70326878569046E-5,
0.00437432926208278,0.008671626066204,0.0108202744682646,0.0129689228703252,
0.0151175712723858,0.0172662196744464),.UNSPECIFIED.);
#1441=B_SPLINE_CURVE_WITH_KNOTS('',3,(#50970,#50971,#50972,#50973,#50974,
#50975,#50976,#50977,#50978,#50979,#50980,#50981,#50982,#50983,#50984,#50985,
#50986,#50987,#50988,#50989,#50990,#50991,#50992,#50993,#50994,#50995,#50996,
#50997,#50998,#50999,#51000,#51001,#51002,#51003,#51004,#51005,#51006,#51007,
#51008,#51009,#51010,#51011,#51012,#51013,#51014,#51015,#51016,#51017,#51018,
#51019,#51020,#51021,#51022,#51023,#51024,#51025,#51026,#51027,#51028,#51029,
#51030,#51031,#51032,#51033,#51034,#51035,#51036),.UNSPECIFIED.,.F.,.F.,
(4,3,3,3,3,3,3,3,3,3,3,3,3,3,3,3,3,3,3,3,3,3,4),(1.42349606405191E-7,0.125,
0.1875,0.25,0.3125,0.375,0.4375,0.46875,0.484375,0.5,0.515625,0.53125,0.5625,
0.625,0.6875,0.75,0.8125,0.832640388956925,0.84375,0.875,0.90625,0.9375,
1.),.UNSPECIFIED.);
#1442=B_SPLINE_CURVE_WITH_KNOTS('',3,(#51038,#51039,#51040,#51041,#51042,
#51043,#51044,#51045,#51046,#51047,#51048,#51049,#51050,#51051,#51052,#51053,
#51054,#51055,#51056,#51057,#51058,#51059,#51060,#51061,#51062),
 .UNSPECIFIED.,.F.,.F.,(4,3,3,3,3,3,3,3,4),(0.,0.0171992441380122,0.25,
0.5,0.625,0.75,0.8125,0.875,1.),.UNSPECIFIED.);
#1443=B_SPLINE_CURVE_WITH_KNOTS('',3,(#51064,#51065,#51066,#51067,#51068,
#51069,#51070,#51071,#51072,#51073,#51074,#51075,#51076),.UNSPECIFIED.,
 .F.,.F.,(4,3,3,3,4),(0.,0.500000000000001,0.548723791104437,0.75,1.),
 .UNSPECIFIED.);
#1444=B_SPLINE_CURVE_WITH_KNOTS('',3,(#51077,#51078,#51079,#51080,#51081,
#51082,#51083,#51084),.UNSPECIFIED.,.F.,.F.,(4,1,1,1,1,4),(-5.99999999944752E-8,
0.00312786895657466,0.00469183343486199,0.00625579791314932,0.00938372686972398,
0.0125116558262986),.UNSPECIFIED.);
#1445=B_SPLINE_CURVE_WITH_KNOTS('',3,(#51127,#51128,#51129,#51130,#51131,
#51132,#51133,#51134,#51135,#51136,#51137,#51138,#51139,#51140,#51141,#51142,
#51143,#51144,#51145,#51146,#51147,#51148,#51149,#51150,#51151,#51152,#51153,
#51154,#51155,#51156,#51157,#51158,#51159,#51160,#51161,#51162,#51163,#51164,
#51165,#51166,#51167,#51168,#51169,#51170,#51171,#51172,#51173,#51174,#51175,
#51176,#51177,#51178,#51179,#51180,#51181,#51182,#51183,#51184,#51185,#51186,
#51187,#51188,#51189,#51190,#51191,#51192,#51193,#51194,#51195,#51196,#51197,
#51198,#51199,#51200,#51201,#51202,#51203,#51204,#51205,#51206,#51207,#51208,
#51209,#51210,#51211,#51212,#51213,#51214,#51215,#51216,#51217,#51218,#51219,
#51220,#51221,#51222,#51223,#51224,#51225,#51226,#51227,#51228,#51229,#51230,
#51231,#51232,#51233,#51234,#51235,#51236,#51237,#51238,#51239,#51240,#51241,
#51242,#51243,#51244,#51245,#51246,#51247,#51248,#51249,#51250,#51251,#51252,
#51253,#51254,#51255,#51256,#51257,#51258,#51259,#51260,#51261,#51262,#51263,
#51264,#51265,#51266,#51267,#51268,#51269,#51270,#51271,#51272,#51273,#51274),
 .UNSPECIFIED.,.F.,.F.,(4,3,3,3,3,3,3,3,3,3,3,3,3,3,3,3,3,3,3,3,3,3,3,3,
3,3,3,3,3,3,3,3,3,3,3,3,3,3,3,3,3,3,3,3,3,3,3,3,3,4),(0.,0.0625,0.09375,
0.124731584851994,0.125,0.15625,0.185898086488356,0.1875,0.21875,0.246713282675617,
0.25,0.28125,0.308162129481387,0.328945253391501,0.346341543597235,0.359375,
0.370641832386322,0.375,0.3828125,0.390625,0.3984375,0.40625,0.4140625,
0.421875,0.430538691367311,0.4375,0.46875,0.492575847998397,0.5,0.53125,
0.5625,0.59375,0.609375,0.618852153197554,0.625,0.644295096358991,0.671432424588419,
0.706945894626813,0.730283133511903,0.734375,0.74707850512236,0.75,0.765625,
0.78125,0.84375,0.875,0.876135893436369,0.9375,0.939588219697389,1.),
 .UNSPECIFIED.);
#1446=B_SPLINE_CURVE_WITH_KNOTS('',3,(#51275,#51276,#51277,#51278,#51279,
#51280,#51281,#51282,#51283,#51284,#51285,#51286,#51287),.UNSPECIFIED.,
 .F.,.F.,(4,3,3,3,4),(2.79419382013459E-10,0.290816211170589,0.60141503799362,
0.93668173505155,0.999999998265381),.UNSPECIFIED.);
#1447=B_SPLINE_CURVE_WITH_KNOTS('',3,(#51288,#51289,#51290,#51291,#51292,
#51293,#51294,#51295,#51296,#51297,#51298,#51299,#51300,#51301,#51302,#51303,
#51304,#51305,#51306,#51307,#51308,#51309,#51310,#51311,#51312,#51313,#51314,
#51315,#51316,#51317,#51318,#51319,#51320,#51321,#51322,#51323,#51324,#51325,
#51326,#51327,#51328,#51329,#51330,#51331,#51332,#51333,#51334,#51335,#51336,
#51337,#51338,#51339,#51340,#51341,#51342,#51343,#51344,#51345,#51346,#51347,
#51348),.UNSPECIFIED.,.F.,.F.,(4,3,3,3,3,3,3,3,3,3,3,3,3,3,3,3,3,3,3,3,
4),(0.,0.0625,0.078125,0.09375,0.125,0.15625,0.160643478189123,0.1875,0.25,
0.3125,0.375,0.4375,0.5,0.53125,0.546875,0.5625,0.59375,0.625,0.6875,0.75,
0.999999873926191),.UNSPECIFIED.);
#1448=B_SPLINE_CURVE_WITH_KNOTS('',3,(#51353,#51354,#51355,#51356),
 .UNSPECIFIED.,.F.,.F.,(4,4),(0.,2.22095063237474E-5),.UNSPECIFIED.);
#1449=B_SPLINE_CURVE_WITH_KNOTS('',3,(#51358,#51359,#51360,#51361),
 .UNSPECIFIED.,.F.,.F.,(4,4),(0.,2.22095063236846E-5),.UNSPECIFIED.);
#1450=B_SPLINE_CURVE_WITH_KNOTS('',3,(#51363,#51364,#51365,#51366),
 .UNSPECIFIED.,.F.,.F.,(4,4),(0.,2.2209506323702E-5),.UNSPECIFIED.);
#1451=B_SPLINE_CURVE_WITH_KNOTS('',3,(#51368,#51369,#51370,#51371),
 .UNSPECIFIED.,.F.,.F.,(4,4),(0.,2.22095063237639E-5),.UNSPECIFIED.);
#1452=B_SPLINE_CURVE_WITH_KNOTS('',3,(#51373,#51374,#51375,#51376),
 .UNSPECIFIED.,.F.,.F.,(4,4),(0.,2.2209506323727E-5),.UNSPECIFIED.);
#1453=B_SPLINE_CURVE_WITH_KNOTS('',3,(#51397,#51398,#51399,#51400,#51401,
#51402,#51403),.UNSPECIFIED.,.F.,.F.,(4,3,4),(0.,0.125,0.25),
 .UNSPECIFIED.);
#1454=B_SPLINE_CURVE_WITH_KNOTS('',3,(#51405,#51406,#51407,#51408,#51409,
#51410,#51411,#51412,#51413,#51414,#51415,#51416,#51417,#51418,#51419,#51420,
#51421,#51422,#51423,#51424,#51425,#51426,#51427,#51428,#51429,#51430,#51431,
#51432,#51433,#51434,#51435,#51436,#51437,#51438,#51439,#51440,#51441,#51442,
#51443,#51444,#51445,#51446,#51447,#51448,#51449,#51450),.UNSPECIFIED.,
 .F.,.F.,(4,3,3,3,3,3,3,3,3,3,3,3,3,3,3,4),(0.25,0.3125,0.375,0.4375,0.46875,
0.4765625,0.484375,0.5,0.515625,0.53125,0.5625,0.625,0.6875,0.75,0.875,
1.),.UNSPECIFIED.);
#1455=B_SPLINE_CURVE_WITH_KNOTS('',3,(#51452,#51453,#51454,#51455,#51456,
#51457,#51458,#51459,#51460,#51461,#51462,#51463,#51464),.UNSPECIFIED.,
 .F.,.F.,(4,3,3,3,4),(3.36788025480501E-14,0.351091870377537,0.5,0.845889958604177,
0.999999999999961),.UNSPECIFIED.);
#1456=B_SPLINE_CURVE_WITH_KNOTS('',3,(#51466,#51467,#51468,#51469,#51470,
#51471,#51472,#51473,#51474,#51475,#51476,#51477,#51478,#51479,#51480,#51481,
#51482,#51483,#51484,#51485,#51486,#51487,#51488,#51489,#51490,#51491,#51492,
#51493,#51494,#51495,#51496,#51497,#51498,#51499,#51500,#51501,#51502,#51503,
#51504,#51505,#51506,#51507,#51508,#51509,#51510,#51511,#51512,#51513,#51514),
 .UNSPECIFIED.,.F.,.F.,(4,3,3,3,3,3,3,3,3,3,3,3,3,3,3,3,4),(1.91266793240995E-6,
0.125,0.25,0.3125,0.375,0.4375,0.46875,0.484375,0.5,0.515625,0.53125,0.53515625,
0.53857421875,0.5625,0.625,0.6875,0.75),.UNSPECIFIED.);
#1457=B_SPLINE_CURVE_WITH_KNOTS('',3,(#51516,#51517,#51518,#51519,#51520,
#51521,#51522),.UNSPECIFIED.,.F.,.F.,(4,3,4),(0.75,0.875,1.),
 .UNSPECIFIED.);
#1458=B_SPLINE_CURVE_WITH_KNOTS('',3,(#51524,#51525,#51526,#51527),
 .UNSPECIFIED.,.F.,.F.,(4,4),(7.33287537516016E-16,0.00234848012465154),
 .UNSPECIFIED.);
#1459=B_SPLINE_CURVE_WITH_KNOTS('',3,(#51538,#51539,#51540,#51541),
 .UNSPECIFIED.,.F.,.F.,(4,4),(1.73200015566965E-14,0.00232242609217698),
 .UNSPECIFIED.);
#1460=B_SPLINE_CURVE_WITH_KNOTS('',3,(#51725,#51726,#51727,#51728,#51729,
#51730,#51731,#51732,#51733,#51734,#51735,#51736,#51737,#51738,#51739,#51740,
#51741,#51742,#51743,#51744,#51745,#51746,#51747,#51748,#51749,#51750,#51751,
#51752,#51753,#51754,#51755,#51756,#51757,#51758,#51759,#51760,#51761,#51762,
#51763,#51764,#51765,#51766,#51767,#51768,#51769,#51770,#51771,#51772,#51773,
#51774,#51775,#51776,#51777,#51778,#51779,#51780,#51781,#51782,#51783,#51784,
#51785,#51786,#51787,#51788,#51789,#51790,#51791,#51792,#51793,#51794),
 .UNSPECIFIED.,.F.,.F.,(4,3,3,3,3,3,3,3,3,3,3,3,3,3,3,3,3,3,3,3,3,3,3,4),
(3.70547010534069E-18,0.000685488878875431,0.00136362733180547,0.00203809428842422,
0.00233379670455984,0.00271195014349479,0.00304962754454054,0.00338935778381529,
0.0037325111035576,0.00408059769401021,0.00425701959752223,0.00443534472717101,
0.00461584026680862,0.0047069932936327,0.00479880275422561,0.00489131137324147,
0.0049845646172225,0.00502420741213766,0.00507856216536076,0.0051258809722966,
0.00517358713695751,0.00519763445194167,0.00521516460782795,0.00522531763086377),
 .UNSPECIFIED.);
#1461=B_SPLINE_CURVE_WITH_KNOTS('',3,(#51796,#51797,#51798,#51799,#51800,
#51801,#51802,#51803,#51804,#51805,#51806,#51807,#51808,#51809,#51810,#51811,
#51812,#51813,#51814,#51815,#51816,#51817,#51818,#51819,#51820,#51821,#51822,
#51823,#51824,#51825,#51826,#51827,#51828,#51829,#51830,#51831,#51832,#51833,
#51834,#51835,#51836,#51837,#51838,#51839,#51840,#51841,#51842,#51843,#51844,
#51845,#51846,#51847,#51848,#51849,#51850,#51851,#51852,#51853,#51854,#51855,
#51856,#51857,#51858,#51859,#51860,#51861,#51862,#51863,#51864,#51865,#51866,
#51867,#51868,#51869,#51870,#51871,#51872,#51873,#51874,#51875,#51876,#51877),
 .UNSPECIFIED.,.F.,.F.,(4,3,3,3,3,3,3,3,3,3,3,3,3,3,3,3,3,3,3,3,3,3,3,3,
3,3,3,4),(0.00522531763086377,0.00522824582386111,0.00524825807115921,0.00527773686304108,
0.005310921500641,0.00534817438862756,0.00538918146335247,0.00543238248536955,
0.00547514739040225,0.0055150805388988,0.00557528016196572,0.00564345584262177,
0.00570170125821141,0.00578803619489881,0.00581440066319727,0.00592499322569639,
0.00614208305587578,0.00635423289316619,0.00656198496558043,0.00676580497685607,
0.00696609711170371,0.00735747320605897,0.00773849369111559,0.00811107456944985,
0.00883702717746603,0.00954554528659402,0.010244744341838,0.0115760723897976),
 .UNSPECIFIED.);
#1462=B_SPLINE_CURVE_WITH_KNOTS('',3,(#51878,#51879,#51880,#51881,#51882,
#51883,#51884,#51885,#51886,#51887,#51888,#51889,#51890,#51891,#51892,#51893,
#51894,#51895,#51896,#51897,#51898,#51899,#51900,#51901,#51902,#51903,#51904,
#51905,#51906,#51907,#51908,#51909,#51910,#51911,#51912,#51913,#51914,#51915,
#51916,#51917,#51918,#51919,#51920,#51921,#51922,#51923),.UNSPECIFIED.,
 .F.,.F.,(4,3,3,3,3,3,3,3,3,3,3,3,3,3,3,4),(0.000332625453320718,0.00115607112755972,
0.00186065645282291,0.00239123963891823,0.00362640815027674,0.0045803311999874,
0.00527329949875475,0.00568502233587425,0.00692019084723276,0.00693751245226992,
0.00856708219571078,0.00911007271031551,0.0102139735441888,0.0106256963813083,
0.0112717507118465,0.0135077562411448),.UNSPECIFIED.);
#1463=B_SPLINE_CURVE_WITH_KNOTS('',3,(#51959,#51960,#51961,#51962,#51963,
#51964,#51965,#51966,#51967,#51968,#51969,#51970,#51971,#51972,#51973,#51974,
#51975,#51976,#51977,#51978,#51979,#51980,#51981,#51982,#51983,#51984,#51985,
#51986,#51987,#51988,#51989,#51990,#51991,#51992,#51993,#51994,#51995,#51996,
#51997,#51998,#51999,#52000,#52001),.UNSPECIFIED.,.F.,.F.,(4,3,3,3,3,3,
3,3,3,3,3,3,3,3,4),(0.,0.0803788659656621,0.125,0.199206661927729,0.25,
0.345037361920189,0.375,0.5,0.625,0.654605288102519,0.75,0.800518552305932,
0.875,0.91969786384336,1.),.UNSPECIFIED.);
#1464=B_SPLINE_CURVE_WITH_KNOTS('',3,(#52156,#52157,#52158,#52159,#52160,
#52161,#52162),.UNSPECIFIED.,.F.,.F.,(4,1,1,1,4),(0.,0.00328982736702057,
0.00657965473404115,0.00986948210106172,0.0131593094680823),
 .UNSPECIFIED.);
#1465=B_SPLINE_CURVE_WITH_KNOTS('',3,(#52164,#52165,#52166,#52167,#52168,
#52169,#52170,#52171,#52172,#52173,#52174,#52175,#52176,#52177,#52178,#52179,
#52180,#52181,#52182,#52183,#52184,#52185,#52186,#52187,#52188,#52189,#52190,
#52191,#52192,#52193,#52194,#52195,#52196,#52197,#52198,#52199,#52200,#52201,
#52202,#52203,#52204,#52205,#52206,#52207,#52208,#52209,#52210,#52211,#52212,
#52213,#52214,#52215,#52216,#52217,#52218,#52219,#52220,#52221,#52222,#52223,
#52224,#52225,#52226,#52227,#52228,#52229,#52230,#52231,#52232,#52233,#52234,
#52235,#52236,#52237,#52238,#52239,#52240,#52241,#52242,#52243,#52244,#52245,
#52246,#52247,#52248,#52249,#52250,#52251,#52252,#52253,#52254,#52255,#52256,
#52257,#52258,#52259,#52260,#52261,#52262,#52263),.UNSPECIFIED.,.F.,.F.,
(4,3,3,3,3,3,3,3,3,3,3,3,3,3,3,3,3,3,3,3,3,3,3,3,3,3,3,3,3,3,3,3,3,4),(1.79045146764256E-15,
0.00133239898080196,0.00203135800119964,0.0027393221849017,0.00346457247643882,
0.00383680540508471,0.00421752044955265,0.00460867485617364,0.00480890442754651,
0.00501270574910554,0.00522049417185399,0.00543274922784831,0.00554072296176422,
0.00565003054244384,0.00576075791804394,0.00581233006619133,0.00587405491108055,
0.00593349990772224,0.00599474288809984,0.00605737935932001,0.00612089251884205,
0.00618468694311985,0.00621649466230807,0.00624814061748105,0.00631066365578348,
0.00632608721374795,0.00634141346716181,0.00635663602067303,0.00637174896766624,
0.00640162488731466,0.00643100383429519,0.00648815925212972,0.00654306111029986,
0.00659565065852666),.UNSPECIFIED.);
#1466=B_SPLINE_CURVE_WITH_KNOTS('',3,(#52264,#52265,#52266,#52267,#52268,
#52269,#52270,#52271,#52272,#52273,#52274,#52275,#52276,#52277,#52278,#52279,
#52280,#52281,#52282,#52283,#52284,#52285,#52286,#52287,#52288,#52289,#52290,
#52291,#52292,#52293,#52294,#52295,#52296,#52297,#52298,#52299,#52300,#52301,
#52302,#52303,#52304,#52305,#52306,#52307,#52308,#52309),.UNSPECIFIED.,
 .F.,.F.,(4,3,3,3,3,3,3,3,3,3,3,3,3,3,3,4),(0.00659565065852666,0.00669380080030737,
0.00678763860389039,0.00688067717343409,0.0069731418250513,0.00715645851125297,
0.00733779444607574,0.007517337530045,0.00787172263135117,0.00822084899494823,
0.00856579604438765,0.0089075288715255,0.00958482516796702,0.0102592404404008,
0.0109370028829842,0.0116246601323809),.UNSPECIFIED.);
#1467=B_SPLINE_CURVE_WITH_KNOTS('',3,(#52458,#52459,#52460,#52461,#52462,
#52463,#52464,#52465),.UNSPECIFIED.,.F.,.F.,(4,1,1,1,1,4),(1.77756260508886E-17,
0.00247652675053282,0.00371479012579921,0.00495305350106561,0.00742958025159841,
0.00990610420568183),.UNSPECIFIED.);
#1468=B_SPLINE_CURVE_WITH_KNOTS('',3,(#52467,#52468,#52469,#52470,#52471,
#52472,#52473),.UNSPECIFIED.,.F.,.F.,(4,3,4),(0.890529645287399,0.941951608103805,
1.),.UNSPECIFIED.);
#1469=B_SPLINE_CURVE_WITH_KNOTS('',3,(#52475,#52476,#52477,#52478,#52479,
#52480,#52481,#52482,#52483,#52484,#52485,#52486,#52487,#52488,#52489,#52490,
#52491,#52492,#52493,#52494,#52495,#52496,#52497,#52498,#52499,#52500,#52501,
#52502,#52503,#52504,#52505,#52506,#52507,#52508,#52509,#52510,#52511,#52512,
#52513,#52514,#52515,#52516,#52517,#52518,#52519,#52520,#52521,#52522,#52523,
#52524,#52525,#52526,#52527,#52528,#52529,#52530,#52531,#52532,#52533,#52534,
#52535,#52536,#52537,#52538,#52539,#52540,#52541,#52542,#52543,#52544,#52545,
#52546,#52547,#52548,#52549,#52550,#52551,#52552,#52553,#52554,#52555,#52556,
#52557,#52558,#52559,#52560,#52561,#52562,#52563,#52564,#52565,#52566,#52567,
#52568,#52569,#52570,#52571,#52572,#52573,#52574,#52575,#52576,#52577,#52578,
#52579,#52580,#52581,#52582,#52583,#52584,#52585,#52586,#52587,#52588,#52589,
#52590,#52591,#52592,#52593,#52594,#52595,#52596,#52597,#52598,#52599,#52600,
#52601),.UNSPECIFIED.,.F.,.F.,(4,3,3,3,3,3,3,3,3,3,3,3,3,3,3,3,3,3,3,3,
3,3,3,3,3,3,3,3,3,3,3,3,3,3,3,3,3,3,3,3,3,3,4),(0.4375,0.447953139951671,
0.46875,0.484375,0.5,0.50261698921794,0.515625,0.522734388082496,0.53125,
0.533337365500028,0.543622114252509,0.553625463971614,0.5625,0.568643278230123,
0.574064030279117,0.579758768591498,0.585692930148249,0.588732265688585,
0.590265995396032,0.591807342322294,0.593354897555682,0.594907192948267,
0.598019914889625,0.601133101571348,0.604234327992868,0.610353982579369,
0.616296060704126,0.622000466234711,0.625,0.63268403637845,0.642706690214556,
0.65223168774306,0.670184521519534,0.6875,0.71875,0.746273631098841,0.75,
0.779126048854605,0.78125,0.8125,0.875,0.877403592710768,0.890529645287399),
 .UNSPECIFIED.);
#1470=B_SPLINE_CURVE_WITH_KNOTS('',3,(#52603,#52604,#52605,#52606,#52607,
#52608,#52609,#52610,#52611,#52612,#52613,#52614,#52615,#52616,#52617,#52618,
#52619,#52620,#52621,#52622,#52623,#52624,#52625,#52626,#52627,#52628,#52629,
#52630,#52631,#52632,#52633,#52634,#52635,#52636,#52637,#52638,#52639,#52640,
#52641,#52642,#52643,#52644,#52645,#52646,#52647,#52648),.UNSPECIFIED.,
 .F.,.F.,(4,3,3,3,3,3,3,3,3,3,3,3,3,3,3,4),(0.,0.0680280639044606,0.104883098894702,
0.125,0.144558395882076,0.188305153814917,0.238207334935121,0.25,0.266693333173773,
0.298717535411549,0.3125,0.335981288472857,0.375,0.381870329444042,0.410570188685067,
0.4375),.UNSPECIFIED.);
#1471=B_SPLINE_CURVE_WITH_KNOTS('',3,(#52678,#52679,#52680,#52681,#52682,
#52683,#52684,#52685,#52686,#52687,#52688,#52689,#52690),.UNSPECIFIED.,
 .F.,.F.,(4,3,3,3,4),(0.,0.385769213597709,0.5,0.8882470488323,0.99999999999998),
 .UNSPECIFIED.);
#1472=B_SPLINE_CURVE_WITH_KNOTS('',3,(#52858,#52859,#52860,#52861,#52862,
#52863,#52864,#52865,#52866,#52867,#52868,#52869,#52870,#52871,#52872,#52873,
#52874,#52875,#52876,#52877,#52878,#52879),.UNSPECIFIED.,.F.,.F.,(4,3,3,
3,3,3,3,4),(0.75,0.762630349837623,0.812707493406033,0.856396526178607,
0.875,0.895847435088822,0.932392098898145,1.),.UNSPECIFIED.);
#1473=B_SPLINE_CURVE_WITH_KNOTS('',3,(#52881,#52882,#52883,#52884,#52885,
#52886,#52887,#52888,#52889,#52890,#52891,#52892,#52893,#52894,#52895,#52896,
#52897,#52898,#52899,#52900,#52901,#52902,#52903,#52904,#52905,#52906,#52907,
#52908,#52909,#52910,#52911,#52912,#52913,#52914,#52915,#52916,#52917,#52918,
#52919,#52920,#52921,#52922,#52923,#52924,#52925,#52926,#52927,#52928,#52929,
#52930,#52931,#52932,#52933,#52934,#52935,#52936,#52937,#52938,#52939,#52940,
#52941,#52942,#52943,#52944,#52945,#52946,#52947,#52948,#52949,#52950,#52951,
#52952,#52953,#52954,#52955,#52956,#52957,#52958,#52959,#52960,#52961,#52962,
#52963,#52964,#52965,#52966,#52967,#52968,#52969,#52970,#52971,#52972,#52973,
#52974,#52975,#52976,#52977,#52978,#52979,#52980,#52981,#52982,#52983,#52984,
#52985,#52986,#52987,#52988,#52989,#52990,#52991,#52992,#52993,#52994,#52995,
#52996,#52997,#52998,#52999,#53000,#53001,#53002,#53003,#53004,#53005,#53006,
#53007,#53008,#53009,#53010,#53011,#53012,#53013,#53014,#53015,#53016,#53017,
#53018,#53019,#53020,#53021,#53022,#53023,#53024,#53025,#53026,#53027,#53028,
#53029,#53030,#53031,#53032,#53033,#53034,#53035,#53036,#53037,#53038,#53039,
#53040,#53041,#53042,#53043,#53044,#53045,#53046,#53047,#53048,#53049,#53050,
#53051,#53052,#53053,#53054,#53055,#53056,#53057,#53058,#53059,#53060,#53061,
#53062,#53063,#53064,#53065,#53066,#53067,#53068,#53069,#53070),
 .UNSPECIFIED.,.F.,.F.,(4,3,3,3,3,3,3,3,3,3,3,3,3,3,3,3,3,3,3,3,3,3,3,3,
3,3,3,3,3,3,3,3,3,3,3,3,3,3,3,3,3,3,3,3,3,3,3,3,3,3,3,3,3,3,3,3,3,3,3,3,
3,3,3,4),(0.183933550895872,0.1875,0.21875,0.25,0.25098239560007,0.279533235815916,
0.28125,0.295006732441368,0.31232060369789,0.331303612740551,0.34139109420047,
0.34375,0.351986115795895,0.359375,0.364637802978179,0.375,0.376321507864968,
0.38451085849127,0.388462648085802,0.390625,0.392740169656706,0.397601835508714,
0.400288993494641,0.403160543694781,0.406217079719029,0.40958258006508,
0.411447390674892,0.413444325260174,0.415574852471787,0.417830243347339,
0.418954779483583,0.419628043089068,0.42005515725583,0.421336499756114,
0.42371844902768,0.42676266038335,0.428586931024468,0.430291954434473,0.433433718802995,
0.436311041923835,0.438987607354032,0.443872262911617,0.452821357758043,
0.46160958182739,0.46875,0.478223111052318,0.484375,0.4921875,0.493727913835873,
0.5,0.5078125,0.515625,0.53125,0.542156621633365,0.5625,0.584268222136265,
0.59375,0.615486063512961,0.625,0.66344091850867,0.6875,0.701499573604137,
0.733921780432045,0.75),.UNSPECIFIED.);
#1474=B_SPLINE_CURVE_WITH_KNOTS('',3,(#53072,#53073,#53074,#53075,#53076,
#53077,#53078,#53079,#53080,#53081,#53082,#53083,#53084),.UNSPECIFIED.,
 .F.,.F.,(4,3,3,3,4),(0.,0.0559678243043705,0.11909959188631,0.125,0.183933550895872),
 .UNSPECIFIED.);
#1475=B_SPLINE_CURVE_WITH_KNOTS('',3,(#53085,#53086,#53087,#53088,#53089,
#53090,#53091,#53092,#53093,#53094,#53095,#53096,#53097,#53098,#53099,#53100,
#53101,#53102,#53103,#53104,#53105,#53106,#53107,#53108,#53109,#53110,#53111,
#53112,#53113,#53114,#53115,#53116,#53117,#53118,#53119,#53120,#53121,#53122,
#53123,#53124,#53125,#53126,#53127,#53128,#53129,#53130,#53131,#53132,#53133),
 .UNSPECIFIED.,.F.,.F.,(4,3,3,3,3,3,3,3,3,3,3,3,3,3,3,3,4),(0.000238545193572011,
0.000851590334526773,0.00177115804595892,0.00202346165952711,0.00223094190167499,
0.00269072575739106,0.00319418747363505,0.00391681603930059,0.00425872230842761,
0.00514290632121012,0.00616921820595708,0.00636899660311964,0.00652225788835833,
0.00712664416160244,0.00759508688502917,0.00809898762340667,0.0100472674488482),
 .UNSPECIFIED.);
#1476=B_SPLINE_CURVE_WITH_KNOTS('',3,(#53177,#53178,#53179,#53180,#53181,
#53182,#53183),.UNSPECIFIED.,.F.,.F.,(4,3,4),(1.64794717479639E-14,0.000692615597163757,
0.0022638573967611),.UNSPECIFIED.);
#1477=B_SPLINE_CURVE_WITH_KNOTS('',3,(#53185,#53186,#53187,#53188,#53189,
#53190,#53191,#53192,#53193,#53194),.UNSPECIFIED.,.F.,.F.,(4,1,1,1,1,1,
1,4),(0.,0.000164336190648263,0.000328672381296526,0.000657344762593053,
0.000986017143889579,0.00131468952518611,0.00197203428777916,0.00262937905037221),
 .UNSPECIFIED.);
#1478=B_SPLINE_CURVE_WITH_KNOTS('',3,(#53195,#53196,#53197,#53198,#53199,
#53200,#53201,#53202,#53203,#53204,#53205,#53206,#53207,#53208,#53209,#53210,
#53211,#53212,#53213,#53214,#53215,#53216,#53217,#53218,#53219,#53220,#53221,
#53222),.UNSPECIFIED.,.F.,.F.,(4,3,3,3,3,3,3,3,3,4),(1.58990032769613E-17,
0.000791485231628063,0.000826267123390952,0.00158297046325611,0.00197871307907013,
0.00199274490496515,0.00237445569488416,0.00277019831069818,0.00296806961860519,
0.0031659409265122),.UNSPECIFIED.);
#1479=B_SPLINE_CURVE_WITH_KNOTS('',3,(#53223,#53224,#53225,#53226,#53227,
#53228,#53229),.UNSPECIFIED.,.F.,.F.,(4,3,4),(0.,0.864714126347195,0.999999253323372),
 .UNSPECIFIED.);
#1480=B_SPLINE_CURVE_WITH_KNOTS('',3,(#53280,#53281,#53282,#53283,#53284,
#53285,#53286,#53287,#53288,#53289,#53290,#53291,#53292,#53293,#53294,#53295,
#53296,#53297,#53298),.UNSPECIFIED.,.F.,.F.,(4,3,3,3,3,3,4),(3.84625751079355E-15,
0.000265106688219907,0.000530213376435968,0.000795320064652029,0.00106042675286809,
0.00159064012930021,0.00212085350573233),.UNSPECIFIED.);
#1481=B_SPLINE_CURVE_WITH_KNOTS('',3,(#53300,#53301,#53302,#53303,#53304,
#53305,#53306,#53307,#53308,#53309,#53310,#53311,#53312,#53313,#53314,#53315,
#53316,#53317,#53318,#53319,#53320,#53321,#53322,#53323,#53324,#53325,#53326,
#53327,#53328,#53329,#53330,#53331,#53332,#53333),.UNSPECIFIED.,.F.,.F.,
(4,3,3,3,3,3,3,3,3,3,3,4),(3.93312924486614E-18,0.000498106772859835,0.000538560220293626,
0.000996213545719667,0.00106388037241615,0.00124526693214958,0.0014943203185795,
0.00156579269657072,0.00174337370500941,0.00180010855767657,0.00186790039822437,
0.00199242709143933),.UNSPECIFIED.);
#1482=B_SPLINE_CURVE_WITH_KNOTS('',3,(#53334,#53335,#53336,#53337),
 .UNSPECIFIED.,.F.,.F.,(4,4),(-0.000356991008063635,0.00227547242484036),
 .UNSPECIFIED.);
#1483=B_SPLINE_CURVE_WITH_KNOTS('',3,(#53338,#53339,#53340,#53341),
 .UNSPECIFIED.,.F.,.F.,(4,4),(6.75947242081653E-8,1.),.UNSPECIFIED.);
#1484=B_SPLINE_CURVE_WITH_KNOTS('',3,(#53388,#53389,#53390,#53391),
 .UNSPECIFIED.,.F.,.F.,(4,4),(5.26912590866588E-9,0.00263380354365925),
 .UNSPECIFIED.);
#1485=B_SPLINE_CURVE_WITH_KNOTS('',3,(#53393,#53394,#53395,#53396,#53397,
#53398,#53399,#53400,#53401,#53402,#53403,#53404,#53405,#53406,#53407,#53408,
#53409,#53410,#53411,#53412,#53413,#53414,#53415,#53416,#53417,#53418,#53419,
#53420,#53421,#53422,#53423,#53424,#53425,#53426),.UNSPECIFIED.,.F.,.F.,
(4,3,3,3,3,3,3,3,3,3,3,4),(0.,0.000124653703275801,0.000184227434801142,
0.000249307406551601,0.00041766537279728,0.000498614813103202,0.000747922219654804,
0.000922322810580849,0.000997229626206405,0.00145222768964327,0.00149584443930961,
0.00199445925241281),.UNSPECIFIED.);
#1486=B_SPLINE_CURVE_WITH_KNOTS('',3,(#53427,#53428,#53429,#53430,#53431,
#53432,#53433,#53434,#53435,#53436,#53437,#53438,#53439,#53440,#53441,#53442,
#53443,#53444,#53445),.UNSPECIFIED.,.F.,.F.,(4,3,3,3,3,3,4),(3.90312782094781E-18,
0.000530467727866949,0.00106093545573389,0.00132616931966737,0.00159140318360084,
0.00185663704753431,0.00212187091146779),.UNSPECIFIED.);
#1487=B_SPLINE_CURVE_WITH_KNOTS('',3,(#53446,#53447,#53448,#53449),
 .UNSPECIFIED.,.F.,.F.,(4,4),(0.,1.),.UNSPECIFIED.);
#1488=B_SPLINE_CURVE_WITH_KNOTS('',3,(#53452,#53453,#53454,#53455,#53456,
#53457,#53458),.UNSPECIFIED.,.F.,.F.,(4,3,4),(7.59701845949959E-7,0.86537068925697,
1.),.UNSPECIFIED.);
#1489=B_SPLINE_CURVE_WITH_KNOTS('',3,(#53505,#53506,#53507,#53508,#53509,
#53510,#53511,#53512,#53513,#53514,#53515,#53516,#53517,#53518,#53519,#53520,
#53521,#53522,#53523,#53524,#53525,#53526,#53527,#53528,#53529,#53530,#53531,
#53532),.UNSPECIFIED.,.F.,.F.,(4,3,3,3,3,3,3,3,3,4),(5.70737205233477E-16,
0.000202064457052415,0.000404128914104259,0.000808257828207947,0.00119619719877999,
0.00121238674231163,0.00161651565641532,0.00237726972942536,0.0024247734846227,
0.00323303131283008),.UNSPECIFIED.);
#1490=B_SPLINE_CURVE_WITH_KNOTS('',3,(#53534,#53535,#53536,#53537,#53538,
#53539,#53540,#53541,#53542,#53543,#53544,#53545,#53546,#53547,#53548,#53549,
#53550,#53551,#53552,#53553,#53554,#53555,#53556,#53557,#53558,#53559,#53560,
#53561,#53562,#53563,#53564,#53565,#53566,#53567),.UNSPECIFIED.,.F.,.F.,
(4,3,3,3,3,3,3,3,3,3,3,4),(7.94950163848063E-18,0.000640690988150711,0.000699211931287781,
0.00128138197630141,0.00137633837260762,0.00160172747037677,0.00192207296445212,
0.00201766788276466,0.00224241845852747,0.00231776125826869,0.00240259120556514,
0.00256276376725831),.UNSPECIFIED.);
#1491=B_SPLINE_CURVE_WITH_KNOTS('',3,(#53568,#53569,#53570,#53571,#53572,
#53573,#53574),.UNSPECIFIED.,.F.,.F.,(4,3,4),(-0.000461466528563571,0.00111744893139882,
0.00182907629052203),.UNSPECIFIED.);
#1492=B_SPLINE_CURVE_WITH_KNOTS('',3,(#53584,#53585,#53586,#53587,#53588,
#53589,#53590,#53591,#53592,#53593,#53594,#53595),.UNSPECIFIED.,.F.,.F.,
(4,2,2,2,2,4),(-0.0429082490477899,-0.0358623622035485,-0.0270225822664231,
-0.0151674140885932,0.,0.000281753242151189),.UNSPECIFIED.);
#1493=B_SPLINE_CURVE_WITH_KNOTS('',3,(#53604,#53605,#53606,#53607,#53608,
#53609,#53610,#53611,#53612,#53613,#53614,#53615,#53616,#53617),
 .UNSPECIFIED.,.F.,.F.,(4,2,2,2,2,2,4),(-0.0423657771798303,-0.0371697057665082,
-0.0311389710525321,-0.022717188634609,-0.0120263902095206,-3.97598620693884E-15,
0.00034806785588522),.UNSPECIFIED.);
#1494=B_SPLINE_CURVE_WITH_KNOTS('',3,(#53619,#53620,#53621,#53622,#53623,
#53624,#53625,#53626,#53627,#53628,#53629,#53630,#53631,#53632),
 .UNSPECIFIED.,.F.,.F.,(4,2,2,2,2,2,4),(-0.0423574776745687,-0.0371604407800644,
-0.0311227690155774,-0.022675758099277,-0.0120468921834928,-2.5882074261574E-15,
0.000356146845347506),.UNSPECIFIED.);
#1495=B_SPLINE_CURVE_WITH_KNOTS('',3,(#53641,#53642,#53643,#53644,#53645,
#53646,#53647,#53648,#53649,#53650,#53651,#53652),.UNSPECIFIED.,.F.,.F.,
(4,2,2,2,2,4),(0.0382003500357908,0.043948148696183,0.0511593452998606,
0.060830394704669,0.0732034634623376,0.0734333083269417),.UNSPECIFIED.);
#1496=B_SPLINE_CURVE_WITH_KNOTS('',3,(#53673,#53674,#53675,#53676,#53677,
#53678,#53679),.UNSPECIFIED.,.F.,.F.,(4,3,4),(0.,0.726667315922346,1.),
 .UNSPECIFIED.);
#1497=B_SPLINE_CURVE_WITH_KNOTS('',3,(#53686,#53687,#53688,#53689,#53690,
#53691,#53692),.UNSPECIFIED.,.F.,.F.,(4,3,4),(1.07390946806767E-6,0.86016968037695,
0.999942871118562),.UNSPECIFIED.);
#1498=B_SPLINE_CURVE_WITH_KNOTS('',3,(#53693,#53694,#53695,#53696,#53697,
#53698,#53699,#53700,#53701,#53702,#53703,#53704,#53705,#53706,#53707,#53708,
#53709,#53710,#53711,#53712,#53713,#53714,#53715,#53716,#53717,#53718,#53719,
#53720,#53721,#53722,#53723),.UNSPECIFIED.,.F.,.F.,(4,3,3,3,3,3,3,3,3,3,
4),(1.34228257431211E-16,3.87540787402395E-5,7.75081574803447E-5,0.000155016314960555,
0.000310032629920976,0.000465048944881397,0.000620065259841818,0.00093009788976266,
0.0012401305196835,0.00186019577952519,0.00248026103936687),
 .UNSPECIFIED.);
#1499=B_SPLINE_CURVE_WITH_KNOTS('',3,(#53778,#53779,#53780,#53781,#53782,
#53783,#53784),.UNSPECIFIED.,.F.,.F.,(4,3,4),(0.,0.816373731602943,1.),
 .UNSPECIFIED.);
#1500=B_SPLINE_CURVE_WITH_KNOTS('',3,(#53793,#53794,#53795,#53796,#53797,
#53798,#53799,#53800,#53801,#53802,#53803,#53804,#53805,#53806,#53807,#53808,
#53809,#53810,#53811,#53812,#53813,#53814,#53815,#53816,#53817,#53818,#53819,
#53820,#53821,#53822,#53823),.UNSPECIFIED.,.F.,.F.,(4,3,3,3,3,3,3,3,3,3,
4),(4.26082128994329E-16,0.000617840564227267,0.00123568112845411,0.00154460141056753,
0.00185352169268095,0.00200798183373766,0.00216244197479437,0.00231690211585108,
0.00239413218637943,0.00243274722164361,0.00247136225690779),
 .UNSPECIFIED.);
#1501=B_SPLINE_CURVE_WITH_KNOTS('',3,(#53824,#53825,#53826,#53827,#53828,
#53829,#53830),.UNSPECIFIED.,.F.,.F.,(4,3,4),(3.15157433218311E-5,0.776531405694898,
0.999998921742255),.UNSPECIFIED.);
#1502=B_SPLINE_CURVE_WITH_KNOTS('',3,(#53872,#53873,#53874,#53875,#53876,
#53877,#53878),.UNSPECIFIED.,.F.,.F.,(4,3,4),(0.,0.5,1.),.UNSPECIFIED.);
#1503=B_SPLINE_CURVE_WITH_KNOTS('',3,(#53882,#53883,#53884,#53885,#53886,
#53887,#53888,#53889,#53890,#53891,#53892,#53893,#53894,#53895,#53896,#53897,
#53898,#53899,#53900,#53901,#53902,#53903,#53904,#53905,#53906,#53907,#53908,
#53909,#53910,#53911,#53912,#53913,#53914,#53915,#53916,#53917,#53918,#53919,
#53920,#53921),.UNSPECIFIED.,.F.,.F.,(4,3,3,3,3,3,3,3,3,3,3,3,3,4),(3.87981183129397E-18,
0.000476315485915268,0.00053559406864673,0.000952630971830532,0.0010598222626488,
0.00119078871478816,0.0014289464577458,0.00154802532922461,0.00155886726192386,
0.00166710420070343,0.00177886290992897,0.00184572250792165,0.00188774403954471,
0.00190526194366106),.UNSPECIFIED.);
#1504=B_SPLINE_CURVE_WITH_KNOTS('',3,(#53922,#53923,#53924,#53925,#53926,
#53927,#53928),.UNSPECIFIED.,.F.,.F.,(4,3,4),(9.15977827778901E-6,0.5,0.999998963616504),
 .UNSPECIFIED.);
#1505=B_SPLINE_CURVE_WITH_KNOTS('',3,(#53982,#53983,#53984,#53985,#53986,
#53987,#53988),.UNSPECIFIED.,.F.,.F.,(4,3,4),(0.,0.661687537605397,0.999999849194684),
 .UNSPECIFIED.);
#1506=B_SPLINE_CURVE_WITH_KNOTS('',3,(#53993,#53994,#53995,#53996,#53997,
#53998,#53999),.UNSPECIFIED.,.F.,.F.,(4,3,4),(1.05656453661477E-6,0.769344479228148,
0.999985988157446),.UNSPECIFIED.);
#1507=B_SPLINE_CURVE_WITH_KNOTS('',3,(#54000,#54001,#54002,#54003,#54004,
#54005,#54006,#54007,#54008,#54009,#54010,#54011,#54012,#54013,#54014,#54015,
#54016,#54017,#54018,#54019,#54020,#54021,#54022,#54023,#54024,#54025,#54026,
#54027,#54028,#54029,#54030),.UNSPECIFIED.,.F.,.F.,(4,3,3,3,3,3,3,3,3,3,
4),(7.59605884606955E-17,3.00957540793479E-5,6.01915081586198E-5,0.000120383016317164,
0.000240766032634251,0.000361149048951339,0.000481532065268427,0.000722298097902602,
0.000963064130536778,0.00144459619580513,0.00192612826107348),
 .UNSPECIFIED.);
#1508=B_SPLINE_CURVE_WITH_KNOTS('',3,(#54034,#54035,#54036,#54037,#54038,
#54039,#54040,#54041,#54042,#54043,#54044,#54045,#54046,#54047,#54048,#54049),
 .UNSPECIFIED.,.F.,.F.,(4,2,2,2,2,2,2,4),(-0.0333293903198794,-0.0329576040327539,
-0.0259519923232747,-0.0185023367726281,-0.0101196043509111,-0.00508448543974312,
-4.19109191795997E-15,0.00022476035086433),.UNSPECIFIED.);
#1509=B_SPLINE_CURVE_WITH_KNOTS('',3,(#54050,#54051,#54052,#54053,#54054,
#54055,#54056,#54057,#54058,#54059,#54060,#54061),.UNSPECIFIED.,.F.,.F.,
(4,2,2,2,2,4),(0.0333293903199977,0.0401691226088174,0.0479843704625406,
0.0568871869476023,0.0666660435803344,0.066890541210896),.UNSPECIFIED.);
#1510=B_SPLINE_CURVE_WITH_KNOTS('',3,(#54079,#54080,#54081,#54082,#54083,
#54084,#54085,#54086,#54087,#54088,#54089,#54090,#54091,#54092,#54093,#54094,
#54095,#54096,#54097,#54098,#54099,#54100,#54101,#54102,#54103,#54104,#54105,
#54106,#54107,#54108,#54109),.UNSPECIFIED.,.F.,.F.,(4,3,3,3,3,3,3,3,3,3,
4),(0.,1.25074494335884E-5,5.94103848095448E-5,0.000200119190937414,0.000212626640371002,
0.000224352374214991,0.00031229537804491,0.000356266879959869,0.000378252630917348,
0.000389245506396088,0.000400238381874828),.UNSPECIFIED.);
#1511=B_SPLINE_CURVE_WITH_KNOTS('',3,(#54111,#54112,#54113,#54114,#54115,
#54116,#54117,#54118,#54119,#54120),.UNSPECIFIED.,.F.,.F.,(4,2,2,2,4),(0.0495097784252302,
0.0511592393817984,0.0608272218939915,0.0732022980075359,0.0734320722136546),
 .UNSPECIFIED.);
#1520=(
BOUNDED_CURVE()
B_SPLINE_CURVE(2,(#49167,#49168,#49169),.UNSPECIFIED.,.F.,.F.)
B_SPLINE_CURVE_WITH_KNOTS((3,3),(-0.999979498354126,-3.91220184957483E-5),
 .UNSPECIFIED.)
CURVE()
GEOMETRIC_REPRESENTATION_ITEM()
RATIONAL_B_SPLINE_CURVE((0.999987153020195,0.686696441488091,0.999975485362207))
REPRESENTATION_ITEM('')
);
#1521=(
BOUNDED_CURVE()
B_SPLINE_CURVE(2,(#49183,#49184,#49185),.UNSPECIFIED.,.F.,.F.)
B_SPLINE_CURVE_WITH_KNOTS((3,3),(-1.00003164257888,4.00451552356698E-5),
 .UNSPECIFIED.)
CURVE()
GEOMETRIC_REPRESENTATION_ITEM()
RATIONAL_B_SPLINE_CURVE((1.00001982986642,0.686645949278685,1.00002509582908))
REPRESENTATION_ITEM('')
);
#1522=(
BOUNDED_CURVE()
B_SPLINE_CURVE(2,(#49260,#49261,#49262),.UNSPECIFIED.,.F.,.F.)
B_SPLINE_CURVE_WITH_KNOTS((3,3),(-0.999979498354114,-3.91220185005021E-5),
 .UNSPECIFIED.)
CURVE()
GEOMETRIC_REPRESENTATION_ITEM()
RATIONAL_B_SPLINE_CURVE((0.999987153020188,0.686696441488096,0.999975485362204))
REPRESENTATION_ITEM('')
);
#1523=(
BOUNDED_CURVE()
B_SPLINE_CURVE(2,(#49276,#49277,#49278),.UNSPECIFIED.,.F.,.F.)
B_SPLINE_CURVE_WITH_KNOTS((3,3),(-1.00003164257888,4.00451552399089E-5),
 .UNSPECIFIED.)
CURVE()
GEOMETRIC_REPRESENTATION_ITEM()
RATIONAL_B_SPLINE_CURVE((1.00001982986642,0.686645949278685,1.00002509582908))
REPRESENTATION_ITEM('')
);
#1524=(
BOUNDED_CURVE()
B_SPLINE_CURVE(2,(#49353,#49354,#49355),.UNSPECIFIED.,.F.,.F.)
B_SPLINE_CURVE_WITH_KNOTS((3,3),(-0.999979498354106,-3.9122018497479E-5),
 .UNSPECIFIED.)
CURVE()
GEOMETRIC_REPRESENTATION_ITEM()
RATIONAL_B_SPLINE_CURVE((0.999987153020183,0.686696441488098,0.999975485362207))
REPRESENTATION_ITEM('')
);
#1525=(
BOUNDED_CURVE()
B_SPLINE_CURVE(2,(#49369,#49370,#49371),.UNSPECIFIED.,.F.,.F.)
B_SPLINE_CURVE_WITH_KNOTS((3,3),(-1.00003164257888,4.00451552363315E-5),
 .UNSPECIFIED.)
CURVE()
GEOMETRIC_REPRESENTATION_ITEM()
RATIONAL_B_SPLINE_CURVE((1.00001982986642,0.686645949278687,1.00002509582908))
REPRESENTATION_ITEM('')
);
#1526=(
BOUNDED_CURVE()
B_SPLINE_CURVE(2,(#49446,#49447,#49448),.UNSPECIFIED.,.F.,.F.)
B_SPLINE_CURVE_WITH_KNOTS((3,3),(-0.999979498354116,-3.91220185320975E-5),
 .UNSPECIFIED.)
CURVE()
GEOMETRIC_REPRESENTATION_ITEM()
RATIONAL_B_SPLINE_CURVE((0.999987153020189,0.686696441488106,0.999975485362184))
REPRESENTATION_ITEM('')
);
#1527=(
BOUNDED_CURVE()
B_SPLINE_CURVE(2,(#49462,#49463,#49464),.UNSPECIFIED.,.F.,.F.)
B_SPLINE_CURVE_WITH_KNOTS((3,3),(-1.00003164257888,4.0045155211594E-5),
 .UNSPECIFIED.)
CURVE()
GEOMETRIC_REPRESENTATION_ITEM()
RATIONAL_B_SPLINE_CURVE((1.00001982986642,0.686645949278692,1.00002509582907))
REPRESENTATION_ITEM('')
);
#1528=(
BOUNDED_CURVE()
B_SPLINE_CURVE(2,(#49539,#49540,#49541),.UNSPECIFIED.,.F.,.F.)
B_SPLINE_CURVE_WITH_KNOTS((3,3),(-0.999979498354118,-3.91220184959991E-5),
 .UNSPECIFIED.)
CURVE()
GEOMETRIC_REPRESENTATION_ITEM()
RATIONAL_B_SPLINE_CURVE((0.99998715302019,0.686696441488094,0.999975485362207))
REPRESENTATION_ITEM('')
);
#1529=(
BOUNDED_CURVE()
B_SPLINE_CURVE(2,(#49555,#49556,#49557),.UNSPECIFIED.,.F.,.F.)
B_SPLINE_CURVE_WITH_KNOTS((3,3),(-1.00003164257889,4.00451552394756E-5),
 .UNSPECIFIED.)
CURVE()
GEOMETRIC_REPRESENTATION_ITEM()
RATIONAL_B_SPLINE_CURVE((1.00001982986643,0.686645949278681,1.00002509582908))
REPRESENTATION_ITEM('')
);
#1707=(
BOUNDED_SURFACE()
B_SPLINE_SURFACE(3,2,((#49132,#49133,#49134),(#49135,#49136,#49137),(#49138,
#49139,#49140),(#49141,#49142,#49143),(#49144,#49145,#49146),(#49147,#49148,
#49149),(#49150,#49151,#49152),(#49153,#49154,#49155),(#49156,#49157,#49158),
(#49159,#49160,#49161),(#49162,#49163,#49164)),.UNSPECIFIED.,.T.,.F.,.F.)
B_SPLINE_SURFACE_WITH_KNOTS((4,1,1,1,1,1,1,1,4),(3,3),(-0.010465367918601,
-0.00915719692877588,-0.00784902593895075,-0.00654085494912563,-0.00523268395930051,
-0.00392451296947538,-0.00261634197965026,-0.00130817098982514,0.),(-9.28189933853903E-5,
1.00709936745582),.UNSPECIFIED.)
GEOMETRIC_REPRESENTATION_ITEM()
RATIONAL_B_SPLINE_SURFACE(((1.00005816990851,0.684423875674772,1.00448036293941),
(1.0000582548459,0.683963083961899,1.00448690498728),(1.00005264871468,
0.714376767023455,1.00405510952515),(1.00004410969851,0.760701571366749,
1.00339741738511),(1.00005214672296,0.717100109865145,1.00401644511616),
(1.000061052267,0.66878686428705,1.00470236796737),(1.00005266324573,0.714297935018859,
1.00405622873527),(1.00004410774396,0.760712174947014,1.00339726684175),
(1.00005213909035,0.717141517300695,1.00401585723791),(1.00005808497112,
0.684884667387646,1.00447382089153),(1.00005816990851,0.684423875674772,
1.00448036293941)))
REPRESENTATION_ITEM('')
SURFACE()
);
#1708=(
BOUNDED_SURFACE()
B_SPLINE_SURFACE(3,2,((#49225,#49226,#49227),(#49228,#49229,#49230),(#49231,
#49232,#49233),(#49234,#49235,#49236),(#49237,#49238,#49239),(#49240,#49241,
#49242),(#49243,#49244,#49245),(#49246,#49247,#49248),(#49249,#49250,#49251),
(#49252,#49253,#49254),(#49255,#49256,#49257)),.UNSPECIFIED.,.T.,.F.,.F.)
B_SPLINE_SURFACE_WITH_KNOTS((4,1,1,1,1,1,1,1,4),(3,3),(-0.010465367918601,
-0.00915719692877587,-0.00784902593895075,-0.00654085494912562,-0.00523268395930049,
-0.00392451296947537,-0.00261634197965024,-0.00130817098982511,0.),(-9.28189933903628E-5,
1.0070993674559),.UNSPECIFIED.)
GEOMETRIC_REPRESENTATION_ITEM()
RATIONAL_B_SPLINE_SURFACE(((1.00005816990851,0.684423875674746,1.00448036293946),
(1.0000582548459,0.683963083961873,1.00448690498733),(1.00005264871469,
0.714376767023432,1.0040551095252),(1.00004410969851,0.760701571366722,
1.00339741738514),(1.00005214672296,0.717100109865137,1.00401644511621),
(1.000061052267,0.668786864287018,1.00470236796742),(1.00005266324573,0.714297935018832,
1.00405622873532),(1.00004410774396,0.760712174947011,1.00339726684179),
(1.00005213909036,0.717141517300666,1.00401585723796),(1.00005808497112,
0.684884667387618,1.00447382089158),(1.00005816990851,0.684423875674746,
1.00448036293946)))
REPRESENTATION_ITEM('')
SURFACE()
);
#1709=(
BOUNDED_SURFACE()
B_SPLINE_SURFACE(3,2,((#49318,#49319,#49320),(#49321,#49322,#49323),(#49324,
#49325,#49326),(#49327,#49328,#49329),(#49330,#49331,#49332),(#49333,#49334,
#49335),(#49336,#49337,#49338),(#49339,#49340,#49341),(#49342,#49343,#49344),
(#49345,#49346,#49347),(#49348,#49349,#49350)),.UNSPECIFIED.,.T.,.F.,.F.)
B_SPLINE_SURFACE_WITH_KNOTS((4,1,1,1,1,1,1,1,4),(3,3),(-0.010465367918601,
-0.00915719692877587,-0.00784902593895075,-0.00654085494912562,-0.00523268395930049,
-0.00392451296947537,-0.00261634197965024,-0.00130817098982511,0.),(-9.28189933861358E-5,
1.00709936745573),.UNSPECIFIED.)
GEOMETRIC_REPRESENTATION_ITEM()
RATIONAL_B_SPLINE_SURFACE(((1.00005816990851,0.6844238756748,1.00448036293935),
(1.0000582548459,0.683963083961927,1.00448690498722),(1.00005264871468,
0.714376767023479,1.0040551095251),(1.00004410969851,0.760701571366764,
1.00339741738506),(1.00005214672296,0.717100109865185,1.00401644511611),
(1.000061052267,0.668786864287076,1.00470236796731),(1.00005266324573,0.714297935018881,
1.00405622873522),(1.00004410774396,0.760712174947052,1.00339726684171),
(1.00005213909035,0.717141517300717,1.00401585723786),(1.00005808497112,
0.684884667387673,1.00447382089148),(1.00005816990851,0.6844238756748,1.00448036293935)))
REPRESENTATION_ITEM('')
SURFACE()
);
#1710=(
BOUNDED_SURFACE()
B_SPLINE_SURFACE(3,2,((#49411,#49412,#49413),(#49414,#49415,#49416),(#49417,
#49418,#49419),(#49420,#49421,#49422),(#49423,#49424,#49425),(#49426,#49427,
#49428),(#49429,#49430,#49431),(#49432,#49433,#49434),(#49435,#49436,#49437),
(#49438,#49439,#49440),(#49441,#49442,#49443)),.UNSPECIFIED.,.T.,.F.,.F.)
B_SPLINE_SURFACE_WITH_KNOTS((4,1,1,1,1,1,1,1,4),(3,3),(-0.0104653679186011,
-0.00915719692877597,-0.00784902593895083,-0.0065408549491257,-0.00523268395930056,
-0.00392451296947543,-0.0026163419796503,-0.00130817098982516,0.),(-9.28189933908896E-5,
1.00709936745538),.UNSPECIFIED.)
GEOMETRIC_REPRESENTATION_ITEM()
RATIONAL_B_SPLINE_SURFACE(((1.00005816990851,0.684423875674909,1.00448036293913),
(1.0000582548459,0.683963083962039,1.004486904987),(1.00005264871469,0.714376767023586,
1.0040551095249),(1.00004410969851,0.760701571366847,1.00339741738489),
(1.00005214672296,0.717100109865272,1.00401644511591),(1.000061052267,0.668786864287198,
1.00470236796707),(1.00005266324573,0.714297935018957,1.00405622873502),
(1.00004410774396,0.760712174947142,1.00339726684154),(1.00005213909036,
0.717141517300806,1.00401585723766),(1.00005808497112,0.68488466738778,
1.00447382089125),(1.00005816990851,0.684423875674909,1.00448036293913)))
REPRESENTATION_ITEM('')
SURFACE()
);
#1711=(
BOUNDED_SURFACE()
B_SPLINE_SURFACE(3,2,((#49504,#49505,#49506),(#49507,#49508,#49509),(#49510,
#49511,#49512),(#49513,#49514,#49515),(#49516,#49517,#49518),(#49519,#49520,
#49521),(#49522,#49523,#49524),(#49525,#49526,#49527),(#49528,#49529,#49530),
(#49531,#49532,#49533),(#49534,#49535,#49536)),.UNSPECIFIED.,.T.,.F.,.F.)
B_SPLINE_SURFACE_WITH_KNOTS((4,1,1,1,1,1,1,1,4),(3,3),(-0.010465367918601,
-0.00915719692877588,-0.00784902593895076,-0.00654085494912564,-0.00523268395930052,
-0.0039245129694754,-0.00261634197965027,-0.00130817098982515,0.),(-9.28189933859035E-5,
1.00709936745473),.UNSPECIFIED.)
GEOMETRIC_REPRESENTATION_ITEM()
RATIONAL_B_SPLINE_SURFACE(((1.00005816990851,0.684423875675114,1.00448036293871),
(1.0000582548459,0.683963083962243,1.00448690498659),(1.00005264871468,
0.71437676702377,1.00405510952452),(1.00004410969851,0.760701571367001,
1.00339741738458),(1.00005214672296,0.717100109865461,1.00401644511554),
(1.000061052267,0.668786864287407,1.00470236796664),(1.00005266324573,0.714297935019167,
1.00405622873464),(1.00004410774396,0.760712174947296,1.00339726684123),
(1.00005213909035,0.717141517300991,1.00401585723729),(1.00005808497112,
0.684884667387984,1.00447382089084),(1.00005816990851,0.684423875675114,
1.00448036293871)))
REPRESENTATION_ITEM('')
SURFACE()
);
#1712=(
BOUNDED_SURFACE()
B_SPLINE_SURFACE(3,2,((#51569,#51570,#51571),(#51572,#51573,#51574),(#51575,
#51576,#51577),(#51578,#51579,#51580),(#51581,#51582,#51583),(#51584,#51585,
#51586),(#51587,#51588,#51589),(#51590,#51591,#51592),(#51593,#51594,#51595),
(#51596,#51597,#51598),(#51599,#51600,#51601),(#51602,#51603,#51604),(#51605,
#51606,#51607),(#51608,#51609,#51610),(#51611,#51612,#51613),(#51614,#51615,
#51616),(#51617,#51618,#51619),(#51620,#51621,#51622),(#51623,#51624,#51625),
(#51626,#51627,#51628),(#51629,#51630,#51631),(#51632,#51633,#51634),(#51635,
#51636,#51637),(#51638,#51639,#51640),(#51641,#51642,#51643),(#51644,#51645,
#51646),(#51647,#51648,#51649),(#51650,#51651,#51652),(#51653,#51654,#51655),
(#51656,#51657,#51658),(#51659,#51660,#51661),(#51662,#51663,#51664),(#51665,
#51666,#51667),(#51668,#51669,#51670),(#51671,#51672,#51673),(#51674,#51675,
#51676),(#51677,#51678,#51679),(#51680,#51681,#51682),(#51683,#51684,#51685),
(#51686,#51687,#51688),(#51689,#51690,#51691),(#51692,#51693,#51694),(#51695,
#51696,#51697),(#51698,#51699,#51700),(#51701,#51702,#51703),(#51704,#51705,
#51706),(#51707,#51708,#51709),(#51710,#51711,#51712),(#51713,#51714,#51715),
(#51716,#51717,#51718),(#51719,#51720,#51721)),.UNSPECIFIED.,.F.,.F.,.F.)
B_SPLINE_SURFACE_WITH_KNOTS((4,1,1,1,1,1,1,1,1,1,1,1,1,1,1,1,1,1,1,1,1,
1,1,1,1,1,1,1,1,1,1,1,1,1,1,1,1,1,1,1,1,1,1,1,1,1,1,1,4),(3,3),(0.0518556011495693,
0.0527138134588282,0.053572025768087,0.0544302380773458,0.0552884503866047,
0.0557175565412341,0.0561466626958635,0.056575768850493,0.0570048750051224,
0.0572194280824371,0.0574339811597518,0.0576485342370665,0.0577558107757239,
0.0578630873143813,0.0579703638530386,0.058077640391696,0.0581849169303533,
0.058238555199682,0.0582921934690107,0.058319012603675,0.0583324221710072,
0.0583458317383393,0.0583525365220054,0.0583592413056715,0.0583726508730037,
0.058399470007668,0.0584262891423324,0.0584531082769967,0.058479927411661,
0.0585067465463254,0.0585335656809897,0.0585603848156541,0.0586140230849827,
0.0586676613543114,0.0587212996236401,0.0588285761622974,0.0589358527009548,
0.0591504057782695,0.0593649588555842,0.0595795119328989,0.0597940650102137,
0.0600086180875284,0.0604377242421578,0.0608668303967872,0.0612959365514166,
0.0621541488606755,0.0630123611699343,0.0638705734791932,0.0655869980977109),
(0.,0.992792082539057),.UNSPECIFIED.)
GEOMETRIC_REPRESENTATION_ITEM()
RATIONAL_B_SPLINE_SURFACE(((1.,0.972633129448393,0.999605483711799),(1.,
0.972466377099184,0.99960307983746),(1.,0.972148941685609,0.99959850374094),
(1.,0.971773197203986,0.99959308707052),(1.,0.971559616448449,0.999590008125606),
(1.,0.971579911851545,0.999590300700786),(1.,0.971765309373093,0.999592973360852),
(1.,0.972004806824618,0.999596425916577),(1.,0.972363384740146,0.999601595116614),
(1.,0.972780617477487,0.99960760987488),(1.,0.973200212475753,0.999613658687109),
(1.,0.973562382687643,0.999618879673097),(1.,0.973908001496278,0.999623862056788),
(1.,0.974213764697866,0.999628269888628),(1.,0.974458567755711,0.999631798929098),
(1.,0.974719713112157,0.999635563557447),(1.,0.974998257795603,0.999639579011622),
(1.,0.975245417202801,0.999643142020835),(1.,0.975453404959813,0.999646140338006),
(1.,0.975586309882469,0.999648056273432),(1.,0.975684096253627,0.999649465945616),
(1.,0.975736704855896,0.999650224342542),(1.,0.975779062452084,0.999650834962656),
(1.,0.975792003625264,0.999651021520472),(1.,0.975908768836828,0.999652704788487),
(1.,0.976065613949059,0.999654965841733),(1.,0.976313695495099,0.999658542144348),
(1.,0.976550038655931,0.999661949228339),(1.,0.976622806276155,0.99966299823434),
(1.,0.975803080158142,0.999651181197942),(1.,0.974689019040623,0.999635121076779),
(1.,0.973731835785377,0.999621322480981),(1.,0.972580633402563,0.999604726937469),
(1.,0.971352050442573,0.99958701588833),(1.,0.970101157684635,0.999568983224826),
(1.,0.968635702989752,0.999547857471859),(1.,0.96708115063371,0.999525447301717),
(1.,0.964966417199759,0.999494961653629),(1.,0.962813822852091,0.99946393020886),
(1.,0.960726792115487,0.999433843918284),(1.,0.958985775800798,0.999408745714495),
(1.,0.957502218932609,0.999387359003586),(1.,0.955794846906811,0.999362745810312),
(1.,0.954070061596803,0.999337881590007),(1.,0.952465322779582,0.999314747940125),
(1.,0.950801594537222,0.999290763908429),(1.,0.949428667831148,0.999270972023674),
(1.,0.948542326646378,0.99925819467547),(1.,0.948107945986102,0.999251932715578),
(1.,0.948414256938409,0.999256348443701),(1.,0.948789582111737,0.999261759069442)))
REPRESENTATION_ITEM('')
SURFACE()
);
#1713=(
BOUNDED_SURFACE()
B_SPLINE_SURFACE(3,2,((#51924,#51925,#51926),(#51927,#51928,#51929),(#51930,
#51931,#51932),(#51933,#51934,#51935),(#51936,#51937,#51938),(#51939,#51940,
#51941),(#51942,#51943,#51944),(#51945,#51946,#51947),(#51948,#51949,#51950),
(#51951,#51952,#51953),(#51954,#51955,#51956)),.UNSPECIFIED.,.F.,.F.,.F.)
B_SPLINE_SURFACE_WITH_KNOTS((4,1,1,1,1,1,1,1,4),(3,3),(0.0274600167716821,
0.0306293591014511,0.0337987014312201,0.036968043760989,0.040137386090758,
0.043306728420527,0.046476070750296,0.049645413080065,0.0528147554098339),
(0.,0.999158823292938),.UNSPECIFIED.)
GEOMETRIC_REPRESENTATION_ITEM()
RATIONAL_B_SPLINE_SURFACE(((1.,0.972499180711492,0.999953733902779),(1.,
0.969563181973315,0.999948794515278),(1.,0.964404879424878,0.999940116427374),
(1.,0.959820144441259,0.999932403282822),(1.,0.957768745632045,0.999928952105031),
(1.,0.957323191790612,0.999928202526005),(1.,0.957772770292401,0.999928958875932),
(1.,0.959817788845774,0.999932399319878),(1.,0.964400556847234,0.999940109155271),
(1.,0.969511549840245,0.999948707651782),(1.,0.972457626668796,0.999953663994193)))
REPRESENTATION_ITEM('')
SURFACE()
);
#1714=(
BOUNDED_SURFACE()
B_SPLINE_SURFACE(3,2,((#52002,#52003,#52004),(#52005,#52006,#52007),(#52008,
#52009,#52010),(#52011,#52012,#52013),(#52014,#52015,#52016),(#52017,#52018,
#52019),(#52020,#52021,#52022),(#52023,#52024,#52025),(#52026,#52027,#52028),
(#52029,#52030,#52031),(#52032,#52033,#52034),(#52035,#52036,#52037),(#52038,
#52039,#52040),(#52041,#52042,#52043),(#52044,#52045,#52046),(#52047,#52048,
#52049),(#52050,#52051,#52052),(#52053,#52054,#52055),(#52056,#52057,#52058),
(#52059,#52060,#52061),(#52062,#52063,#52064),(#52065,#52066,#52067),(#52068,
#52069,#52070),(#52071,#52072,#52073),(#52074,#52075,#52076),(#52077,#52078,
#52079),(#52080,#52081,#52082),(#52083,#52084,#52085),(#52086,#52087,#52088),
(#52089,#52090,#52091),(#52092,#52093,#52094),(#52095,#52096,#52097),(#52098,
#52099,#52100),(#52101,#52102,#52103),(#52104,#52105,#52106),(#52107,#52108,
#52109),(#52110,#52111,#52112),(#52113,#52114,#52115),(#52116,#52117,#52118),
(#52119,#52120,#52121),(#52122,#52123,#52124),(#52125,#52126,#52127),(#52128,
#52129,#52130),(#52131,#52132,#52133),(#52134,#52135,#52136),(#52137,#52138,
#52139),(#52140,#52141,#52142),(#52143,#52144,#52145),(#52146,#52147,#52148),
(#52149,#52150,#52151),(#52152,#52153,#52154)),.UNSPECIFIED.,.F.,.F.,.F.)
B_SPLINE_SURFACE_WITH_KNOTS((4,1,1,1,1,1,1,1,1,1,1,1,1,1,1,1,1,1,1,1,1,
1,1,1,1,1,1,1,1,1,1,1,1,1,1,1,1,1,1,1,1,1,1,1,1,1,1,1,4),(3,3),(0.0549773880899424,
0.0558467220379677,0.056716055985993,0.0575853899340184,0.0584547238820437,
0.0588893908560563,0.059324057830069,0.0597587248040816,0.0601933917780943,
0.0604107252651006,0.060628058752107,0.0608453922391133,0.0609540589826165,
0.0610627257261196,0.0611713924696228,0.061280059213126,0.0613343925848776,
0.0613887259566291,0.0614430593283807,0.0614702260142565,0.0614973927001323,
0.0615109760430702,0.0615177677145391,0.0615245593860081,0.061538142728946,
0.0615517260718839,0.0616060594436355,0.0616332261295112,0.061660392815387,
0.0617147261871386,0.0617690595588902,0.0618233929306418,0.0618777263023934,
0.061932059674145,0.0620407264176481,0.0621493931611513,0.0622580599046544,
0.0623667266481576,0.0625840601351639,0.0628013936221703,0.0630187271091766,
0.0632360605961829,0.0636707275701956,0.0641053945442083,0.0645400615182209,
0.0654093954662462,0.0662787294142715,0.0671480633622969,0.0688867312583475),
(0.0071934162772836,1.),.UNSPECIFIED.)
GEOMETRIC_REPRESENTATION_ITEM()
RATIONAL_B_SPLINE_SURFACE(((0.999606865695227,0.972674019574369,1.),(0.999604493486164,
0.972509132059776,1.),(0.999599985924059,0.972195820419529,1.),(0.99959469878352,
0.97182832183922,1.),(0.999591787920345,0.971625993553036,1.),(0.999592262320468,
0.971658968158147,1.),(0.999595111580877,0.971857014559129,1.),(0.999598719790412,
0.972107813998253,1.),(0.999604075332896,0.972480067061186,1.),(0.999610278894004,
0.972911264205102,1.),(0.999616504333946,0.973343982103104,1.),(0.999621872051548,
0.973717081434168,1.),(0.999626989683936,0.974072797841428,1.),(0.999631514141331,
0.97438728383948,1.),(0.999635134621242,0.974638936167879,1.),(0.999638995891387,
0.974907325344667,1.),(0.999642423004491,0.975145537132501,1.),(0.999645303509732,
0.975345755299341,1.),(0.999647519951942,0.975499815771031,1.),(0.999649466882302,
0.975635143012321,1.),(0.999650966259817,0.975739361749083,1.),(0.999652131141739,
0.975820330365203,1.),(0.999652527992851,0.975847914693448,1.),(0.999653424322134,
0.975910216751927,1.),(0.99965486617898,0.976010437341898,1.),(0.999656495605389,
0.976123695517568,1.),(0.999660353374776,0.976391841363585,1.),(0.999665654480073,
0.976760310606368,1.),(0.999660382980781,0.97639389921788,1.),(0.999642122172533,
0.975124626903821,1.),(0.999618855766348,0.973507425473537,1.),(0.999597068940179,
0.971993066695347,1.),(0.999578353121333,0.970692167503353,1.),(0.999561988209168,
0.969554675139877,1.),(0.999542407463857,0.968193656636564,1.),(0.999521161635198,
0.966716901514952,1.),(0.99949931886217,0.965198653982345,1.),(0.999480183940009,
0.963868623755846,1.),(0.999457441535243,0.962287844617692,1.),(0.999433158062626,
0.960599948930796,1.),(0.999408652723323,0.958896631733652,1.),(0.999387680310542,
0.957438881203672,1.),(0.99936345490367,0.955755021550734,1.),(0.99933892884738,
0.954050264357146,1.),(0.999316157675712,0.952467485689127,1.),(0.999292552850348,
0.950826761417559,1.),(0.999273004213266,0.949467974693082,1.),(0.999260366937433,
0.948589582886857,1.),(0.999254191533472,0.94816034288997,1.),(0.999258647490592,
0.948470067570712,1.),(0.999264080382697,0.948847697051352,1.)))
REPRESENTATION_ITEM('')
SURFACE()
);
#1715=(
BOUNDED_SURFACE()
B_SPLINE_SURFACE(3,2,((#52310,#52311,#52312),(#52313,#52314,#52315),(#52316,
#52317,#52318),(#52319,#52320,#52321),(#52322,#52323,#52324),(#52325,#52326,
#52327),(#52328,#52329,#52330),(#52331,#52332,#52333),(#52334,#52335,#52336),
(#52337,#52338,#52339),(#52340,#52341,#52342),(#52343,#52344,#52345),(#52346,
#52347,#52348),(#52349,#52350,#52351),(#52352,#52353,#52354),(#52355,#52356,
#52357),(#52358,#52359,#52360),(#52361,#52362,#52363),(#52364,#52365,#52366),
(#52367,#52368,#52369),(#52370,#52371,#52372),(#52373,#52374,#52375),(#52376,
#52377,#52378),(#52379,#52380,#52381),(#52382,#52383,#52384),(#52385,#52386,
#52387),(#52388,#52389,#52390),(#52391,#52392,#52393),(#52394,#52395,#52396),
(#52397,#52398,#52399),(#52400,#52401,#52402),(#52403,#52404,#52405),(#52406,
#52407,#52408),(#52409,#52410,#52411),(#52412,#52413,#52414),(#52415,#52416,
#52417),(#52418,#52419,#52420),(#52421,#52422,#52423),(#52424,#52425,#52426),
(#52427,#52428,#52429),(#52430,#52431,#52432),(#52433,#52434,#52435),(#52436,
#52437,#52438),(#52439,#52440,#52441),(#52442,#52443,#52444),(#52445,#52446,
#52447),(#52448,#52449,#52450),(#52451,#52452,#52453),(#52454,#52455,#52456)),
 .UNSPECIFIED.,.F.,.F.,.F.)
B_SPLINE_SURFACE_WITH_KNOTS((4,1,1,1,1,1,1,1,1,1,1,1,1,1,1,1,1,1,1,1,1,
1,1,1,1,1,1,1,1,1,1,1,1,1,1,1,1,1,1,1,1,1,1,1,1,1,4),(3,3),(0.0264470415813064,
0.0280904658576036,0.0289121779957522,0.0297338901339008,0.0305556022720494,
0.031377314410198,0.0317881704792723,0.0321990265483466,0.0326098826174209,
0.0330207386864952,0.0332261667210323,0.0334315947555695,0.0336370227901066,
0.0338424508246438,0.0339451648419123,0.0340478788591809,0.0341505928764495,
0.0342533068937181,0.0343046639023524,0.0343560209109866,0.0344073779196209,
0.0344587349282552,0.0344844134325724,0.0344908330586516,0.0344972526847309,
0.0345036723108102,0.0345100919368895,0.0345229311890481,0.0345357704412066,
0.0345614489455238,0.0345871274498409,0.0346128059541581,0.0346641629627924,
0.0347155199714267,0.034766876980061,0.0348695909973295,0.0349723050145981,
0.0350750190318667,0.0352804470664038,0.035485875100941,0.0358967311700153,
0.0363075872390896,0.0367184433081639,0.0371292993772382,0.0379510115153868,
0.0387727236535354,0.039594435791684),(0.0092590728241763,1.00003353933066),
 .UNSPECIFIED.)
GEOMETRIC_REPRESENTATION_ITEM()
RATIONAL_B_SPLINE_SURFACE(((0.99978961747398,0.988638737368156,1.0000007692208),
(0.999781382332911,0.988194016020487,1.00000079933091),(0.999768697684378,
0.987509008448325,1.00000084570974),(0.999753627458576,0.986695172829483,
1.00000090081095),(0.999744161654649,0.986183992141261,1.00000093542073),
(0.999737468268737,0.985822530014733,1.00000095989373),(0.99973519309943,
0.985699664316171,1.00000096821242),(0.99973614054353,0.985750829027678,
1.00000096474829),(0.999738491598624,0.985877792777406,1.00000095615213),
(0.999742772930425,0.986108997031503,1.00000094049832),(0.999748231548623,
0.986403778143447,1.00000092053999),(0.999753939590464,0.986712028850878,
1.0000008996697),(0.999758950041984,0.986982607670794,1.00000088135001),
(0.999764751091548,0.987295881063196,1.00000086013965),(0.999770296259429,
0.98759533610742,1.00000083986488),(0.999775187421617,0.98785947295972,
1.00000082198134),(0.999779088017462,0.988070116375048,1.00000080771961),
(0.999783226816312,0.988293623439104,1.00000079258693),(0.999786866208497,
0.988490161104194,1.00000077928024),(0.999789885779805,0.988653226655847,
1.00000076823979),(0.999792201848896,0.988778301060619,1.00000075977156),
(0.999794571142586,0.988906249747113,1.00000075110872),(0.999796573339135,
0.989014374130155,1.0000007437881),(0.999797909962534,0.989086555645273,
1.00000073890101),(0.999798507874639,0.989118844621846,1.00000073671486),
(0.999798847443193,0.989137182302254,1.0000007354733),(0.999799031432296,
0.989147118243971,1.00000073480058),(0.999802525289213,0.989335796585208,
1.000000722026),(0.999804716867525,0.989454148129176,1.00000071401295),
(0.99980662464054,0.989557173369326,1.00000070703756),(0.999804818702909,
0.989459647533336,1.00000071364061),(0.99979931983484,0.989162692812403,
1.00000073374609),(0.999790180893756,0.988669163659588,1.00000076716077),
(0.999777974706557,0.98800999437815,1.0000008117902),(0.99976387234001,
0.987248425947972,1.00000086335263),(0.999746122600327,0.986289888858417,
1.00000092825093),(0.999726420849751,0.985225937555842,1.00000100028637),
(0.999705699374946,0.9841069182065,1.00000107605021),(0.99968115178329,
0.982781277522072,1.00000116580347),(0.999655015039571,0.98136981804707,
1.00000126136715),(0.999620253220177,0.979492579632052,1.00000138846665),
(0.999586859443545,0.977689219468202,1.00000151056418),(0.999556749601363,
0.976063201227523,1.00000162065468),(0.999533861409886,0.974827172934429,
1.00000170434069),(0.9995106558406,0.973574005325064,1.00000178918712),
(0.999492456288907,0.97259117709081,1.00000185573007),(0.999482414904449,
0.972048913395374,1.00000189244434),(0.999481440401765,0.971996287442349,
1.00000189600741),(0.999482031626613,0.972028215287785,1.00000189384572)))
REPRESENTATION_ITEM('')
SURFACE()
);
#1716=(
BOUNDED_SURFACE()
B_SPLINE_SURFACE(3,2,((#52650,#52651,#52652),(#52653,#52654,#52655),(#52656,
#52657,#52658),(#52659,#52660,#52661),(#52662,#52663,#52664),(#52665,#52666,
#52667),(#52668,#52669,#52670),(#52671,#52672,#52673),(#52674,#52675,#52676)),
 .UNSPECIFIED.,.F.,.F.,.F.)
B_SPLINE_SURFACE_WITH_KNOTS((4,1,1,1,1,1,4),(3,3),(0.0199977630484638,0.0246245671030636,
0.026855473567606,0.0290863800321484,0.0313172864966908,0.0335481929612332,
0.0381749960364376),(0.,0.999290254333488),.UNSPECIFIED.)
GEOMETRIC_REPRESENTATION_ITEM()
RATIONAL_B_SPLINE_SURFACE(((1.,0.988770559028899,0.999984059905866),(1.,
0.986589245178597,0.999980963549762),(1.,0.984866673614857,0.999978518374356),
(1.,0.98480091247204,0.999978425026984),(1.,0.984960622739239,0.999978651734324),
(1.,0.984785723305408,0.999978403466094),(1.,0.984833323646006,0.999978471034365),
(1.,0.986526872930274,0.999980875012895),(1.,0.988716343491653,0.999983982947382)))
REPRESENTATION_ITEM('')
SURFACE()
);
#1717=(
BOUNDED_SURFACE()
B_SPLINE_SURFACE(3,2,((#52692,#52693,#52694),(#52695,#52696,#52697),(#52698,
#52699,#52700),(#52701,#52702,#52703),(#52704,#52705,#52706),(#52707,#52708,
#52709),(#52710,#52711,#52712),(#52713,#52714,#52715),(#52716,#52717,#52718),
(#52719,#52720,#52721),(#52722,#52723,#52724),(#52725,#52726,#52727),(#52728,
#52729,#52730),(#52731,#52732,#52733),(#52734,#52735,#52736),(#52737,#52738,
#52739),(#52740,#52741,#52742),(#52743,#52744,#52745),(#52746,#52747,#52748),
(#52749,#52750,#52751),(#52752,#52753,#52754),(#52755,#52756,#52757),(#52758,
#52759,#52760),(#52761,#52762,#52763),(#52764,#52765,#52766),(#52767,#52768,
#52769),(#52770,#52771,#52772),(#52773,#52774,#52775),(#52776,#52777,#52778),
(#52779,#52780,#52781),(#52782,#52783,#52784),(#52785,#52786,#52787),(#52788,
#52789,#52790),(#52791,#52792,#52793),(#52794,#52795,#52796),(#52797,#52798,
#52799),(#52800,#52801,#52802),(#52803,#52804,#52805),(#52806,#52807,#52808),
(#52809,#52810,#52811),(#52812,#52813,#52814),(#52815,#52816,#52817),(#52818,
#52819,#52820),(#52821,#52822,#52823),(#52824,#52825,#52826),(#52827,#52828,
#52829),(#52830,#52831,#52832),(#52833,#52834,#52835),(#52836,#52837,#52838),
(#52839,#52840,#52841),(#52842,#52843,#52844),(#52845,#52846,#52847),(#52848,
#52849,#52850),(#52851,#52852,#52853),(#52854,#52855,#52856)),
 .UNSPECIFIED.,.F.,.F.,.F.)
B_SPLINE_SURFACE_WITH_KNOTS((4,1,1,1,1,1,1,1,1,1,1,1,1,1,1,1,1,1,1,1,1,
1,1,1,1,1,1,1,1,1,1,1,1,1,1,1,1,1,1,1,1,1,1,1,1,1,1,1,1,1,1,1,4),(3,3),
(0.0486184959373272,0.0502403308116338,0.051051248248787,0.0518621656859403,
0.0526730831230936,0.0534840005602469,0.0538894592788235,0.0542949179974001,
0.0547003767159768,0.0551058354345534,0.0553085647938417,0.0555112941531301,
0.0557140235124184,0.0559167528717067,0.056119482230995,0.0562208469106392,
0.0563222115902833,0.0564869291947051,0.0564932644871829,0.0564995997796606,
0.0565059350721384,0.0565091027183773,0.0565122703646161,0.0565138541877356,
0.056515438010855,0.0565170218339745,0.0565186056570939,0.0565217733033328,
0.0565249409495717,0.0565376115345272,0.0565502821194827,0.0565629527044382,
0.0565756232893937,0.0566009644593048,0.0566263056292158,0.0566516467991268,
0.0566769879690379,0.05672767030886,0.0567783526486821,0.0568290349885041,
0.0569303996681483,0.0570317643477925,0.0571331290274366,0.0572344937070808,
0.0573358583867249,0.0575385877460133,0.0577413171053016,0.0579440464645899,
0.0583495051831665,0.0591604226203198,0.0599713400574731,0.0607822574946264,
0.0615931749317796),(0.,0.991165909752447),.UNSPECIFIED.)
GEOMETRIC_REPRESENTATION_ITEM()
RATIONAL_B_SPLINE_SURFACE(((1.,0.988579705956782,0.999798224183537),(1.,
0.988129226965691,0.999790265039413),(1.,0.987439893836455,0.999778085777264),
(1.,0.986625048090304,0.999763688935546),(1.,0.986111622194986,0.999754617634157),
(1.,0.9857486338806,0.999748204291101),(1.,0.985627260338365,0.999746059841449),
(1.,0.985683472003575,0.999747052999296),(1.,0.985816599097477,0.999749405112821),
(1.,0.986057632374737,0.999753663732267),(1.,0.98636574427647,0.99975910750896),
(1.,0.986689926424631,0.999764835217667),(1.,0.986975306492696,0.999769877364219),
(1.,0.987306481284958,0.999775728620225),(1.,0.987687389316159,0.999782458572072),
(1.,0.988049270371101,0.999788852351869),(1.,0.988366516495903,0.999794457513663),
(1.,0.988670704507122,0.99979983196235),(1.,0.988911877377787,0.999804093048157),
(1.,0.989074395964705,0.999806964455887),(1.,0.98909185437314,0.999807272914197),
(1.,0.989106320171297,0.99980752849853),(1.,0.989117495068773,0.999807725938636),
(1.,0.989127192857273,0.999807897280914),(1.,0.989121479139524,0.999807796329917),
(1.,0.989175325491616,0.999808747696985),(1.,0.989270871665965,0.999810435824039),
(1.,0.989370384575404,0.999812194036085),(1.,0.989462621663806,0.999813823697611),
(1.,0.989543515522181,0.999815252944901),(1.,0.989328957337217,0.999811462092163),
(1.,0.989016983430099,0.999805950080862),(1.,0.988696686701124,0.999800291020443),
(1.,0.988288392274654,0.999793077200821),(1.,0.987809951865198,0.99978462402931),
(1.,0.987281787718638,0.999775292329838),(1.,0.986791762419011,0.999766634474397),
(1.,0.986187018253921,0.999755949745335),(1.,0.985502666806469,0.999743858500439),
(1.,0.984765419501987,0.999730832681994),(1.,0.983869626093595,0.999715005642368),
(1.,0.982881120683453,0.999697540550362),(1.,0.981843977689429,0.999679216120743),
(1.,0.980929669268354,0.999663061954532),(1.,0.980110711771224,0.999648592465655),
(1.,0.979123821893318,0.999631155917163),(1.,0.978054517766649,0.999612263258849),
(1.,0.97696770723055,0.999593061294133),(1.,0.975726567304752,0.999571132609905),
(1.,0.973998108141452,0.999540593881429),(1.,0.972431575764954,0.99951291610465),
(1.,0.971422011780473,0.99949507894595),(1.,0.971014932146137,0.999487886589495),
(1.,0.971036354184058,0.999488265077928),(1.,0.971102653860526,0.999489436472578)))
REPRESENTATION_ITEM('')
SURFACE()
);
#1718=(
BOUNDED_SURFACE()
B_SPLINE_SURFACE(3,2,((#53134,#53135,#53136),(#53137,#53138,#53139),(#53140,
#53141,#53142),(#53143,#53144,#53145),(#53146,#53147,#53148),(#53149,#53150,
#53151),(#53152,#53153,#53154),(#53155,#53156,#53157),(#53158,#53159,#53160),
(#53161,#53162,#53163),(#53164,#53165,#53166),(#53167,#53168,#53169),(#53170,
#53171,#53172),(#53173,#53174,#53175)),.UNSPECIFIED.,.F.,.F.,.F.)
B_SPLINE_SURFACE_WITH_KNOTS((4,1,1,1,1,1,1,1,1,1,1,4),(3,3),(2.60208521396521E-18,
0.00224502843470091,0.00336754265205136,0.00449005686940182,0.00673508530410272,
0.00785759952145318,0.00898011373880363,0.0112251421735045,0.0134701706082054,
0.0157151990429064,0.0168377132602568,0.0179602274776073),(0.,1.),
 .UNSPECIFIED.)
GEOMETRIC_REPRESENTATION_ITEM()
RATIONAL_B_SPLINE_SURFACE(((1.,0.946871694682909,1.),(1.,0.946299968542447,
1.),(1.,0.946816109299184,1.),(1.,0.948892577451966,1.),(1.,0.949020476847393,
1.),(1.,0.94867679597236,1.),(1.,0.950073546741643,1.),(1.,0.9463002894051,
1.),(1.,0.930830476264166,1.),(1.,0.904147532449761,1.),(1.,0.881006864817563,
1.),(1.,0.861569290206786,1.),(1.,0.850439810109567,1.),(1.,0.84434427061595,
1.)))
REPRESENTATION_ITEM('')
SURFACE()
);
#1719=(
BOUNDED_SURFACE()
B_SPLINE_SURFACE(3,2,((#53231,#53232,#53233),(#53234,#53235,#53236),(#53237,
#53238,#53239),(#53240,#53241,#53242),(#53243,#53244,#53245),(#53246,#53247,
#53248),(#53249,#53250,#53251),(#53252,#53253,#53254),(#53255,#53256,#53257),
(#53258,#53259,#53260),(#53261,#53262,#53263),(#53264,#53265,#53266),(#53267,
#53268,#53269),(#53270,#53271,#53272),(#53273,#53274,#53275),(#53276,#53277,
#53278)),.UNSPECIFIED.,.F.,.F.,.F.)
B_SPLINE_SURFACE_WITH_KNOTS((4,1,1,1,1,1,1,1,1,1,1,1,1,4),(3,3),(-0.00203692429636695,
0.00254615537045871,0.00318269421307338,0.00381923305568806,0.00509231074091741,
0.00636538842614676,0.00700192726876144,0.00763846611137611,0.00891154379660546,
0.0101846214818348,0.0127307768522935,0.0152769322227522,0.0178230875932109,
0.0203692429636696),(-0.00168930119361338,1.00677133507503),
 .UNSPECIFIED.)
GEOMETRIC_REPRESENTATION_ITEM()
RATIONAL_B_SPLINE_SURFACE(((1.00008496330189,0.974681960965966,1.00034229172858),
(1.00010212847963,0.969566945066644,1.00041144509514),(1.00010690360001,
0.968144016797988,1.00043068262677),(1.00009873080779,0.970579410288973,
1.00039775689162),(1.00010107133118,0.969881962553438,1.00040718616024),
(1.00009941607801,0.970375208030169,1.00040051764035),(1.00009727006519,
0.971014693961847,1.00039187199664),(1.00009252792433,0.972427794734359,
1.00037276732959),(1.00009494037177,0.971708914498314,1.00038248635871),
(1.00009557216839,0.971520646726924,1.0003850316783),(1.00009294321431,
0.972304043329874,1.00037444040869),(1.00010749982106,0.96796635011755,
1.00043308462303),(1.00016473057531,0.950912275737492,1.00066365021269),
(1.0002312640321,0.931086108219379,1.00093169360822),(1.000274044616,0.918338010288713,
1.00110404378395),(1.00029567557767,0.911892244649696,1.00119118845814)))
REPRESENTATION_ITEM('')
SURFACE()
);
#1720=(
BOUNDED_SURFACE()
B_SPLINE_SURFACE(3,2,((#53459,#53460,#53461),(#53462,#53463,#53464),(#53465,
#53466,#53467),(#53468,#53469,#53470),(#53471,#53472,#53473),(#53474,#53475,
#53476),(#53477,#53478,#53479),(#53480,#53481,#53482),(#53483,#53484,#53485),
(#53486,#53487,#53488),(#53489,#53490,#53491),(#53492,#53493,#53494),(#53495,
#53496,#53497),(#53498,#53499,#53500),(#53501,#53502,#53503)),
 .UNSPECIFIED.,.F.,.F.,.F.)
B_SPLINE_SURFACE_WITH_KNOTS((4,1,1,1,1,1,1,1,1,1,1,1,4),(3,3),(-0.00112697568940802,
0.00227630595534438,0.00341445893301658,0.00398353542185268,0.00455261191068878,
0.00682891786603319,0.00796707084370539,0.00910522382137759,0.011381529776722,
0.0136578357320664,0.0159341416874108,0.017072294665083,0.0192306646931621),
(-0.0052660988655586,1.00285157929027),.UNSPECIFIED.)
GEOMETRIC_REPRESENTATION_ITEM()
RATIONAL_B_SPLINE_SURFACE(((1.00054177139849,0.948413008428147,1.00029266321785),
(1.00057240532917,0.945496072745762,1.00030921157155),(1.00056048610494,
0.946631010695459,1.00030277284384),(1.00054277515829,0.948317431311034,
1.00029320544576),(1.00052730480877,0.949790504257771,1.00028484841125),
(1.00054259713588,0.948334382447352,1.00029310927861),(1.00053010590215,
0.949523786632503,1.00028636155315),(1.00051694701969,0.950776763737995,
1.00027925316593),(1.00055340254948,0.947305500557184,1.0002989463293),
(1.00071450524393,0.931965445020424,1.00038597350182),(1.00099633115592,
0.905130231890504,1.0005382149795),(1.00124584768938,0.881371489098238,
1.0006730030318),(1.00149815795622,0.857346729494382,1.00080930025014),
(1.00167734639862,0.840284565094988,1.00090609728723),(1.00181930116002,
0.826767758744447,1.0009827808061)))
REPRESENTATION_ITEM('')
SURFACE()
);
#1721=(
BOUNDED_SURFACE()
B_SPLINE_SURFACE(3,2,((#53661,#53662,#53663),(#53664,#53665,#53666),(#53667,
#53668,#53669),(#53670,#53671,#53672)),.UNSPECIFIED.,.F.,.F.,.F.)
B_SPLINE_SURFACE_WITH_KNOTS((4,4),(3,3),(-2.25514051876985E-17,0.00236214428547912),
(-0.00620223654517092,1.),.UNSPECIFIED.)
GEOMETRIC_REPRESENTATION_ITEM()
RATIONAL_B_SPLINE_SURFACE(((1.00099729942381,0.919601629465039,1.),(1.00115637496513,
0.906777582835632,1.),(1.00126632012954,0.89791423462212,1.),(1.00133134190946,
0.892672433583815,1.)))
REPRESENTATION_ITEM('')
SURFACE()
);
#1722=(
BOUNDED_SURFACE()
B_SPLINE_SURFACE(3,2,((#53734,#53735,#53736),(#53737,#53738,#53739),(#53740,
#53741,#53742),(#53743,#53744,#53745),(#53746,#53747,#53748)),
 .UNSPECIFIED.,.F.,.F.,.F.)
B_SPLINE_SURFACE_WITH_KNOTS((4,1,4),(3,3),(3.14159265358979,3.92699081698724,
4.71238898038469),(0.,1.),.UNSPECIFIED.)
GEOMETRIC_REPRESENTATION_ITEM()
RATIONAL_B_SPLINE_SURFACE(((1.,0.48655776526455,1.),(1.,0.486557766002833,
1.),(1.,0.547974422145333,1.),(1.,0.658371714258051,1.),(1.,0.707106781186546,
1.)))
REPRESENTATION_ITEM('')
SURFACE()
);
#1723=(
BOUNDED_SURFACE()
B_SPLINE_SURFACE(3,2,((#53766,#53767,#53768),(#53769,#53770,#53771),(#53772,
#53773,#53774),(#53775,#53776,#53777)),.UNSPECIFIED.,.F.,.F.,.F.)
B_SPLINE_SURFACE_WITH_KNOTS((4,4),(3,3),(4.33680868994202E-19,0.0023350688542472),
(0.,1.00547355602571),.UNSPECIFIED.)
GEOMETRIC_REPRESENTATION_ITEM()
RATIONAL_B_SPLINE_SURFACE(((1.,0.921781046509973,1.0008562716484),(1.,0.909146339862613,
1.00099458519781),(1.,0.900351741222426,1.00109086065457),(1.,0.895068725056835,
1.0011486944245)))
REPRESENTATION_ITEM('')
SURFACE()
);
#1724=(
BOUNDED_SURFACE()
B_SPLINE_SURFACE(3,2,((#53836,#53837,#53838),(#53839,#53840,#53841),(#53842,
#53843,#53844),(#53845,#53846,#53847),(#53848,#53849,#53850)),
 .UNSPECIFIED.,.F.,.F.,.F.)
B_SPLINE_SURFACE_WITH_KNOTS((4,1,4),(3,3),(4.71238898038469,5.49778714378214,
6.28318530717959),(0.,1.),.UNSPECIFIED.)
GEOMETRIC_REPRESENTATION_ITEM()
RATIONAL_B_SPLINE_SURFACE(((1.,0.707106781186548,1.),(1.,0.658371714258676,
1.),(1.,0.547974422145018,1.),(1.,0.486557766002833,1.),(1.,0.48655776526455,
1.)))
REPRESENTATION_ITEM('')
SURFACE()
);
#1725=(
BOUNDED_SURFACE()
B_SPLINE_SURFACE(3,2,((#53860,#53861,#53862),(#53863,#53864,#53865),(#53866,
#53867,#53868),(#53869,#53870,#53871)),.UNSPECIFIED.,.F.,.F.,.F.)
B_SPLINE_SURFACE_WITH_KNOTS((4,4),(3,3),(2.5804011705155E-17,0.00269592513607839),
(0.,1.),.UNSPECIFIED.)
GEOMETRIC_REPRESENTATION_ITEM()
RATIONAL_B_SPLINE_SURFACE(((1.,0.887940178746615,1.),(1.,0.872219487795338,
1.),(1.,0.861659279393505,1.),(1.,0.854938173458171,1.)))
REPRESENTATION_ITEM('')
SURFACE()
);
#1726=(
BOUNDED_SURFACE()
B_SPLINE_SURFACE(3,2,((#53930,#53931,#53932),(#53933,#53934,#53935),(#53936,
#53937,#53938),(#53939,#53940,#53941),(#53942,#53943,#53944)),
 .UNSPECIFIED.,.F.,.F.,.F.)
B_SPLINE_SURFACE_WITH_KNOTS((4,1,4),(3,3),(-0.000302909321607987,0.00578886195052519,
0.0118806332226584),(0.,1.03312425876202),.UNSPECIFIED.)
GEOMETRIC_REPRESENTATION_ITEM()
RATIONAL_B_SPLINE_SURFACE(((1.,0.894876494760464,1.00696427637905),(1.,
0.874392201020365,1.00832133047186),(1.,0.77515446292856,1.01489568350288),
(1.,0.867433891531754,1.00878230815995),(0.999999999999999,0.887390355972598,
1.00746022197573)))
REPRESENTATION_ITEM('')
SURFACE()
);
#1727=(
BOUNDED_SURFACE()
B_SPLINE_SURFACE(3,2,((#53952,#53953,#53954),(#53955,#53956,#53957),(#53958,
#53959,#53960),(#53961,#53962,#53963),(#53964,#53965,#53966)),
 .UNSPECIFIED.,.F.,.F.,.F.)
B_SPLINE_SURFACE_WITH_KNOTS((4,1,4),(3,3),(-0.00116263837286272,0.0058131918643132,
0.0127890221014908),(-0.020297547916368,1.),.UNSPECIFIED.)
GEOMETRIC_REPRESENTATION_ITEM()
RATIONAL_B_SPLINE_SURFACE(((1.0039429407102,0.902871501364518,0.999999999999999),
(1.00444247717786,0.890566161090803,1.),(1.00958527090562,0.763881062256417,
1.),(1.00474383084143,0.883142760372419,1.),(1.00423046655648,0.89578872842398,
0.999999999999999)))
REPRESENTATION_ITEM('')
SURFACE()
);
#1728=(
BOUNDED_SURFACE()
B_SPLINE_SURFACE(3,2,((#53970,#53971,#53972),(#53973,#53974,#53975),(#53976,
#53977,#53978),(#53979,#53980,#53981)),.UNSPECIFIED.,.F.,.F.,.F.)
B_SPLINE_SURFACE_WITH_KNOTS((4,4),(3,3),(-1.68094704822153E-15,0.00269464124111705),
(0.,1.),.UNSPECIFIED.)
GEOMETRIC_REPRESENTATION_ITEM()
RATIONAL_B_SPLINE_SURFACE(((1.,0.888319363951509,1.),(1.,0.87265918860752,
1.),(1.,0.862124260711793,1.),(1.,0.855384875699737,1.)))
REPRESENTATION_ITEM('')
SURFACE()
);
#1729=(
BOUNDED_SURFACE()
B_SPLINE_SURFACE(3,2,((#54121,#54122,#54123),(#54124,#54125,#54126),(#54127,
#54128,#54129),(#54130,#54131,#54132)),.UNSPECIFIED.,.F.,.F.,.F.)
B_SPLINE_SURFACE_WITH_KNOTS((4,4),(3,3),(0.000203890603018781,0.000876640979146271),
(0.,1.00234872771707),.UNSPECIFIED.)
GEOMETRIC_REPRESENTATION_ITEM()
RATIONAL_B_SPLINE_SURFACE(((1.,0.706418854765374,1.00137908434605),(1.,
0.794166685486793,1.00096689282179),(1.,0.870219940196321,1.00060963604717),
(1.,0.870219885219157,1.00060963630542)))
REPRESENTATION_ITEM('')
SURFACE()
);
#1730=(
BOUNDED_SURFACE()
B_SPLINE_SURFACE(3,2,((#54135,#54136,#54137),(#54138,#54139,#54140),(#54141,
#54142,#54143),(#54144,#54145,#54146),(#54147,#54148,#54149),(#54150,#54151,
#54152),(#54153,#54154,#54155),(#54156,#54157,#54158),(#54159,#54160,#54161),
(#54162,#54163,#54164),(#54165,#54166,#54167)),.UNSPECIFIED.,.T.,.F.,.F.)
B_SPLINE_SURFACE_WITH_KNOTS((4,1,1,1,1,1,1,1,4),(3,3),(0.,0.00130817098982512,
0.00261634197965024,0.00392451296947536,0.00523268395930048,0.0065408549491256,
0.00784902593895073,0.00915719692877585,0.010465367918601),(-9.28189933859035E-5,
1.00709936745473),.UNSPECIFIED.)
GEOMETRIC_REPRESENTATION_ITEM()
RATIONAL_B_SPLINE_SURFACE(((1.00005816990851,0.684423875675114,1.00448036293871),
(1.0000582548459,0.683963083962243,1.00448690498659),(1.00005264871468,
0.71437676702377,1.00405510952452),(1.00004410969851,0.760701571367001,
1.00339741738458),(1.00005214672296,0.717100109865461,1.00401644511554),
(1.000061052267,0.668786864287407,1.00470236796664),(1.00005266324573,0.714297935019167,
1.00405622873464),(1.00004410774396,0.760712174947296,1.00339726684123),
(1.00005213909035,0.717141517300991,1.00401585723729),(1.00005808497112,
0.684884667387984,1.00447382089084),(1.00005816990851,0.684423875675114,
1.00448036293871)))
REPRESENTATION_ITEM('')
SURFACE()
);
#1731=(
BOUNDED_SURFACE()
B_SPLINE_SURFACE(3,2,((#54168,#54169,#54170),(#54171,#54172,#54173),(#54174,
#54175,#54176),(#54177,#54178,#54179),(#54180,#54181,#54182),(#54183,#54184,
#54185),(#54186,#54187,#54188),(#54189,#54190,#54191),(#54192,#54193,#54194),
(#54195,#54196,#54197),(#54198,#54199,#54200)),.UNSPECIFIED.,.T.,.F.,.F.)
B_SPLINE_SURFACE_WITH_KNOTS((4,1,1,1,1,1,1,1,4),(3,3),(0.,0.00130817098982513,
0.00261634197965027,0.0039245129694754,0.00523268395930054,0.00654085494912567,
0.0078490259389508,0.00915719692877594,0.0104653679186011),(-9.28189933908896E-5,
1.00709936745538),.UNSPECIFIED.)
GEOMETRIC_REPRESENTATION_ITEM()
RATIONAL_B_SPLINE_SURFACE(((1.00005816990851,0.684423875674909,1.00448036293913),
(1.0000582548459,0.683963083962039,1.004486904987),(1.00005264871469,0.714376767023586,
1.0040551095249),(1.00004410969851,0.760701571366847,1.00339741738489),
(1.00005214672296,0.717100109865272,1.00401644511591),(1.000061052267,0.668786864287198,
1.00470236796707),(1.00005266324573,0.714297935018957,1.00405622873502),
(1.00004410774396,0.760712174947142,1.00339726684154),(1.00005213909036,
0.717141517300806,1.00401585723766),(1.00005808497112,0.68488466738778,
1.00447382089125),(1.00005816990851,0.684423875674909,1.00448036293913)))
REPRESENTATION_ITEM('')
SURFACE()
);
#1732=(
BOUNDED_SURFACE()
B_SPLINE_SURFACE(3,2,((#54201,#54202,#54203),(#54204,#54205,#54206),(#54207,
#54208,#54209),(#54210,#54211,#54212),(#54213,#54214,#54215),(#54216,#54217,
#54218),(#54219,#54220,#54221),(#54222,#54223,#54224),(#54225,#54226,#54227),
(#54228,#54229,#54230),(#54231,#54232,#54233)),.UNSPECIFIED.,.T.,.F.,.F.)
B_SPLINE_SURFACE_WITH_KNOTS((4,1,1,1,1,1,1,1,4),(3,3),(0.,0.00130817098982513,
0.00261634197965025,0.00392451296947538,0.00523268395930051,0.00654085494912563,
0.00784902593895076,0.00915719692877589,0.010465367918601),(-9.28189933861358E-5,
1.00709936745573),.UNSPECIFIED.)
GEOMETRIC_REPRESENTATION_ITEM()
RATIONAL_B_SPLINE_SURFACE(((1.00005816990851,0.6844238756748,1.00448036293935),
(1.0000582548459,0.683963083961927,1.00448690498722),(1.00005264871468,
0.714376767023479,1.0040551095251),(1.00004410969851,0.760701571366764,
1.00339741738506),(1.00005214672296,0.717100109865185,1.00401644511611),
(1.000061052267,0.668786864287076,1.00470236796731),(1.00005266324573,0.714297935018881,
1.00405622873522),(1.00004410774396,0.760712174947052,1.00339726684171),
(1.00005213909035,0.717141517300717,1.00401585723786),(1.00005808497112,
0.684884667387673,1.00447382089148),(1.00005816990851,0.6844238756748,1.00448036293935)))
REPRESENTATION_ITEM('')
SURFACE()
);
#1733=(
BOUNDED_SURFACE()
B_SPLINE_SURFACE(3,2,((#54234,#54235,#54236),(#54237,#54238,#54239),(#54240,
#54241,#54242),(#54243,#54244,#54245),(#54246,#54247,#54248),(#54249,#54250,
#54251),(#54252,#54253,#54254),(#54255,#54256,#54257),(#54258,#54259,#54260),
(#54261,#54262,#54263),(#54264,#54265,#54266)),.UNSPECIFIED.,.T.,.F.,.F.)
B_SPLINE_SURFACE_WITH_KNOTS((4,1,1,1,1,1,1,1,4),(3,3),(0.,0.00130817098982513,
0.00261634197965025,0.00392451296947538,0.00523268395930051,0.00654085494912563,
0.00784902593895076,0.00915719692877589,0.010465367918601),(-9.28189933903628E-5,
1.0070993674559),.UNSPECIFIED.)
GEOMETRIC_REPRESENTATION_ITEM()
RATIONAL_B_SPLINE_SURFACE(((1.00005816990851,0.684423875674746,1.00448036293946),
(1.0000582548459,0.683963083961873,1.00448690498733),(1.00005264871469,
0.714376767023432,1.0040551095252),(1.00004410969851,0.760701571366722,
1.00339741738514),(1.00005214672296,0.717100109865137,1.00401644511621),
(1.000061052267,0.668786864287018,1.00470236796742),(1.00005266324573,0.714297935018832,
1.00405622873532),(1.00004410774396,0.760712174947011,1.00339726684179),
(1.00005213909036,0.717141517300666,1.00401585723796),(1.00005808497112,
0.684884667387618,1.00447382089158),(1.00005816990851,0.684423875674746,
1.00448036293946)))
REPRESENTATION_ITEM('')
SURFACE()
);
#1734=(
BOUNDED_SURFACE()
B_SPLINE_SURFACE(3,2,((#54267,#54268,#54269),(#54270,#54271,#54272),(#54273,
#54274,#54275),(#54276,#54277,#54278),(#54279,#54280,#54281),(#54282,#54283,
#54284),(#54285,#54286,#54287),(#54288,#54289,#54290),(#54291,#54292,#54293),
(#54294,#54295,#54296),(#54297,#54298,#54299)),.UNSPECIFIED.,.T.,.F.,.F.)
B_SPLINE_SURFACE_WITH_KNOTS((4,1,1,1,1,1,1,1,4),(3,3),(0.,0.00130817098982512,
0.00261634197965025,0.00392451296947537,0.00523268395930049,0.00654085494912562,
0.00784902593895074,0.00915719692877586,0.010465367918601),(-9.28189933853903E-5,
1.00709936745582),.UNSPECIFIED.)
GEOMETRIC_REPRESENTATION_ITEM()
RATIONAL_B_SPLINE_SURFACE(((1.00005816990851,0.684423875674772,1.00448036293941),
(1.0000582548459,0.683963083961899,1.00448690498728),(1.00005264871468,
0.714376767023455,1.00405510952515),(1.00004410969851,0.760701571366749,
1.00339741738511),(1.00005214672296,0.717100109865145,1.00401644511616),
(1.000061052267,0.66878686428705,1.00470236796737),(1.00005266324573,0.714297935018859,
1.00405622873527),(1.00004410774396,0.760712174947014,1.00339726684175),
(1.00005213909035,0.717141517300695,1.00401585723791),(1.00005808497112,
0.684884667387646,1.00447382089153),(1.00005816990851,0.684423875674772,
1.00448036293941)))
REPRESENTATION_ITEM('')
SURFACE()
);
#1735=(
BOUNDED_SURFACE()
B_SPLINE_SURFACE(3,2,((#54302,#54303,#54304),(#54305,#54306,#54307),(#54308,
#54309,#54310),(#54311,#54312,#54313),(#54314,#54315,#54316),(#54317,#54318,
#54319),(#54320,#54321,#54322),(#54323,#54324,#54325)),.UNSPECIFIED.,.F.,
 .F.,.F.)
B_SPLINE_SURFACE_WITH_KNOTS((4,1,1,1,1,4),(3,3),(-1.90819582357449E-17,
0.000564455951974709,0.00112891190394944,0.00169336785592416,0.00197559583191153,
0.00225782380789889),(0.,1.),.UNSPECIFIED.)
GEOMETRIC_REPRESENTATION_ITEM()
RATIONAL_B_SPLINE_SURFACE(((1.,0.991835613598268,1.),(1.,0.992614005712327,
1.),(1.,0.994141544760846,1.),(1.,0.99631583526732,1.),(1.,0.998003041423521,
1.),(1.,0.999172568373962,1.),(1.,0.999639015745245,1.),(1.,0.999648793303385,
1.)))
REPRESENTATION_ITEM('')
SURFACE()
);
#1736=(
BOUNDED_SURFACE()
B_SPLINE_SURFACE(3,2,((#54327,#54328,#54329),(#54330,#54331,#54332),(#54333,
#54334,#54335),(#54336,#54337,#54338),(#54339,#54340,#54341),(#54342,#54343,
#54344),(#54345,#54346,#54347)),.UNSPECIFIED.,.F.,.F.,.F.)
B_SPLINE_SURFACE_WITH_KNOTS((4,1,1,1,4),(3,3),(-0.000237302740885216,0.000593256852870235,
0.00118651370574085,0.00177977055861147,0.00261032859115487),(0.,1.01493592684462),
 .UNSPECIFIED.)
GEOMETRIC_REPRESENTATION_ITEM()
RATIONAL_B_SPLINE_SURFACE(((1.,0.999079384901643,1.00002750047952),(1.,
0.999827499951708,1.0000051528962),(1.,0.998481551946456,1.00004535885809),
(1.,0.996274060209497,1.00011130072828),(1.,0.993792671277815,1.00018542441539),
(1.,0.99189007799518,1.00024225840356),(1.,0.990734532561305,1.00027677668769)))
REPRESENTATION_ITEM('')
SURFACE()
);
#1737=(
BOUNDED_SURFACE()
B_SPLINE_SURFACE(3,2,((#54353,#54354,#54355),(#54356,#54357,#54358),(#54359,
#54360,#54361),(#54362,#54363,#54364),(#54365,#54366,#54367),(#54368,#54369,
#54370),(#54371,#54372,#54373),(#54374,#54375,#54376)),.UNSPECIFIED.,.F.,
 .F.,.F.)
B_SPLINE_SURFACE_WITH_KNOTS((4,1,1,1,1,4),(3,3),(-0.00022248774067706,0.000871734875690068,
0.00174346975138016,0.00261520462707025,0.0030510720649153,0.00370942724411761),
(0.,1.00163938212957),.UNSPECIFIED.)
GEOMETRIC_REPRESENTATION_ITEM()
RATIONAL_B_SPLINE_SURFACE(((1.,0.984069198332286,1.00005223334313),(1.,
0.986023953875702,1.00004582416052),(1.,0.9893454078424,1.00003493389596),
(1.,0.993616993324213,1.00002092837415),(1.,0.996528307451787,1.00001138286145),
(1.,0.998741040052508,1.00000412783288),(1.,0.999581963593584,1.00000137064283),
(1.,0.999053363005491,1.00000310379954)))
REPRESENTATION_ITEM('')
SURFACE()
);
#1738=(
BOUNDED_SURFACE()
B_SPLINE_SURFACE(3,2,((#54378,#54379,#54380),(#54381,#54382,#54383),(#54384,
#54385,#54386),(#54387,#54388,#54389),(#54390,#54391,#54392),(#54393,#54394,
#54395),(#54396,#54397,#54398),(#54399,#54400,#54401)),.UNSPECIFIED.,.F.,
 .F.,.F.)
B_SPLINE_SURFACE_WITH_KNOTS((4,1,1,1,1,4),(3,3),(-0.000293385255678526,
0.000366731569601773,0.000733463139204117,0.0014669262784088,0.00220038941761349,
0.00322723781250381),(-0.0485261900086986,1.),.UNSPECIFIED.)
GEOMETRIC_REPRESENTATION_ITEM()
RATIONAL_B_SPLINE_SURFACE(((1.00012540024569,0.998707911689922,1.),(0.999997586898636,
1.00002486390713,1.),(1.00010833407507,0.998883756636833,1.),(1.00035522793121,
0.99633983287021,1.),(1.00065835344187,0.993216514198341,1.),(1.00111105184117,
0.988552039208393,1.),(1.00146600902586,0.984894661773356,1.),(1.00168082818161,
0.982681226557189,1.)))
REPRESENTATION_ITEM('')
SURFACE()
);
#1739=(
BOUNDED_SURFACE()
B_SPLINE_SURFACE(3,2,((#54406,#54407,#54408),(#54409,#54410,#54411),(#54412,
#54413,#54414),(#54415,#54416,#54417),(#54418,#54419,#54420),(#54421,#54422,
#54423),(#54424,#54425,#54426),(#54427,#54428,#54429)),.UNSPECIFIED.,.F.,
 .F.,.F.)
B_SPLINE_SURFACE_WITH_KNOTS((4,1,1,1,1,4),(3,3),(-0.000291172064625148,
0.000727930161563534,0.00145586032312702,0.00218379048469051,0.00254775556547226,
0.00320288287705394),(-0.00425992492820294,1.00188056036606),
 .UNSPECIFIED.)
GEOMETRIC_REPRESENTATION_ITEM()
RATIONAL_B_SPLINE_SURFACE(((1.00014547214641,0.982893257690745,1.00006406708988),
(1.00012675132083,0.985094726129536,1.00005582228945),(1.00009615646836,
0.988692516292073,1.00004234807317),(1.00005704155094,0.993292220284361,
1.00002512155255),(1.00003091594257,0.996364451368782,1.00001361562691),
(1.00000928508564,0.99890812384817,1.00000408922554),(0.99999986210703,
1.00001621547194,0.99999993927084),(1.00001068993421,0.998742921209425,
1.00000470793202)))
REPRESENTATION_ITEM('')
SURFACE()
);
#1740=(
BOUNDED_SURFACE()
B_SPLINE_SURFACE(3,2,((#54431,#54432,#54433),(#54434,#54435,#54436),(#54437,
#54438,#54439),(#54440,#54441,#54442),(#54443,#54444,#54445),(#54446,#54447,
#54448),(#54449,#54450,#54451),(#54452,#54453,#54454)),.UNSPECIFIED.,.F.,
 .F.,.F.)
B_SPLINE_SURFACE_WITH_KNOTS((4,1,1,1,1,4),(3,3),(-0.000348982146594615,
0.000436227682637781,0.000872455365275428,0.00174491073055072,0.00261736609582601,
0.00383880360636252),(0.,1.00191159842478),.UNSPECIFIED.)
GEOMETRIC_REPRESENTATION_ITEM()
RATIONAL_B_SPLINE_SURFACE(((1.,0.998610437460761,1.00000531257112),(1.,
0.999703499185041,1.00000113358098),(1.,0.998779073849389,1.00000466784101),
(1.,0.996351424872412,1.00001394922093),(1.,0.993352180114163,1.00002541592404),
(1.,0.988814006533964,1.00004276625498),(1.,0.985173580066159,1.00005668432198),
(1.,0.982918980573743,1.00006530409966)))
REPRESENTATION_ITEM('')
SURFACE()
);
#1741=(
BOUNDED_SURFACE()
B_SPLINE_SURFACE(3,2,((#54462,#54463,#54464),(#54465,#54466,#54467),(#54468,
#54469,#54470),(#54471,#54472,#54473),(#54474,#54475,#54476),(#54477,#54478,
#54479),(#54480,#54481,#54482)),.UNSPECIFIED.,.F.,.F.,.F.)
B_SPLINE_SURFACE_WITH_KNOTS((4,1,1,1,4),(3,3),(-0.000234670538907357,0.000586676321783697,
0.00117335264356738,0.00176002896535107,0.00258134363634634),(0.,1.01053582586227),
 .UNSPECIFIED.)
GEOMETRIC_REPRESENTATION_ITEM()
RATIONAL_B_SPLINE_SURFACE(((1.,0.990705352673112,1.00019585357137),(1.,
0.991867802793339,1.00017135882729),(1.,0.993772696303182,1.00013121957468),
(1.,0.99626757911702,1.00007864827294),(1.,0.998507262784341,1.00003145443872),
(1.,0.999812010880492,1.00000396124125),(1.,0.999030864962552,1.00002042127598)))
REPRESENTATION_ITEM('')
SURFACE()
);
#1742=(
BOUNDED_SURFACE()
B_SPLINE_SURFACE(3,2,((#54484,#54485,#54486),(#54487,#54488,#54489),(#54490,
#54491,#54492),(#54493,#54494,#54495),(#54496,#54497,#54498),(#54499,#54500,
#54501),(#54502,#54503,#54504),(#54505,#54506,#54507)),.UNSPECIFIED.,.F.,
 .F.,.F.)
B_SPLINE_SURFACE_WITH_KNOTS((4,1,1,1,1,4),(3,3),(-0.000226104302166867,
0.000282630377695824,0.000565260755392034,0.00113052151078445,0.00169578226617687,
0.00248714732372626),(-0.0106186671104657,1.),.UNSPECIFIED.)
GEOMETRIC_REPRESENTATION_ITEM()
RATIONAL_B_SPLINE_SURFACE(((1.00001672252316,0.999212588407443,0.999999999999999),
(1.00000032168945,0.999984852644386,1.),(1.00001379719143,0.999350333178205,
1.),(1.00004410049111,0.997923445068481,1.),(1.00008037719364,0.99621528800171,
1.),(1.00013303469651,0.993735810006735,1.),(1.00017300194076,0.991853876811405,
1.),(1.00019675009217,0.990735650241147,1.)))
REPRESENTATION_ITEM('')
SURFACE()
);
#1755=SHAPE_REPRESENTATION_RELATIONSHIP('SRR','None',#54642,#1769);
#1769=ADVANCED_BREP_SHAPE_REPRESENTATION('',(#1813),#54578);
#1799=STYLED_ITEM('',(#54710),#1813);
#1813=MANIFOLD_SOLID_BREP('Body1',#17678);
#2340=LINE('',#49605,#2933);
#2341=LINE('',#49609,#2934);
#2342=LINE('',#49617,#2935);
#2343=LINE('',#49624,#2936);
#2344=LINE('',#49627,#2937);
#2345=LINE('',#49631,#2938);
#2346=LINE('',#49635,#2939);
#2347=LINE('',#49675,#2940);
#2348=LINE('',#49679,#2941);
#2349=LINE('',#49695,#2942);
#2350=LINE('',#49698,#2943);
#2351=LINE('',#49736,#2944);
#2352=LINE('',#49764,#2945);
#2353=LINE('',#49768,#2946);
#2354=LINE('',#49773,#2947);
#2355=LINE('',#49774,#2948);
#2356=LINE('',#49775,#2949);
#2357=LINE('',#49779,#2950);
#2358=LINE('',#49783,#2951);
#2359=LINE('',#49787,#2952);
#2360=LINE('',#49789,#2953);
#2361=LINE('',#49790,#2954);
#2362=LINE('',#49797,#2955);
#2363=LINE('',#49801,#2956);
#2364=LINE('',#49803,#2957);
#2365=LINE('',#49807,#2958);
#2366=LINE('',#49811,#2959);
#2367=LINE('',#49814,#2960);
#2368=LINE('',#49837,#2961);
#2369=LINE('',#49841,#2962);
#2370=LINE('',#49845,#2963);
#2371=LINE('',#49849,#2964);
#2372=LINE('',#49883,#2965);
#2373=LINE('',#49887,#2966);
#2374=LINE('',#49925,#2967);
#2375=LINE('',#49932,#2968);
#2376=LINE('',#49968,#2969);
#2377=LINE('',#49983,#2970);
#2378=LINE('',#49985,#2971);
#2379=LINE('',#49987,#2972);
#2380=LINE('',#49991,#2973);
#2381=LINE('',#50007,#2974);
#2382=LINE('',#50036,#2975);
#2383=LINE('',#50040,#2976);
#2384=LINE('',#50041,#2977);
#2385=LINE('',#50667,#2978);
#2386=LINE('',#50933,#2979);
#2387=LINE('',#51382,#2980);
#2388=LINE('',#51385,#2981);
#2389=LINE('',#51388,#2982);
#2390=LINE('',#51393,#2983);
#2391=LINE('',#51529,#2984);
#2392=LINE('',#51531,#2985);
#2393=LINE('',#51535,#2986);
#2394=LINE('',#51537,#2987);
#2395=LINE('',#51551,#2988);
#2396=LINE('',#51555,#2989);
#2397=LINE('',#51560,#2990);
#2398=LINE('',#51561,#2991);
#2399=LINE('',#51562,#2992);
#2400=LINE('',#51565,#2993);
#2401=LINE('',#51567,#2994);
#2402=LINE('',#51568,#2995);
#2403=LINE('',#54511,#2996);
#2404=LINE('',#54513,#2997);
#2405=LINE('',#54515,#2998);
#2406=LINE('',#54517,#2999);
#2933=VECTOR('',#23046,1.);
#2934=VECTOR('',#23049,1.);
#2935=VECTOR('',#23058,0.001);
#2936=VECTOR('',#23065,1.);
#2937=VECTOR('',#23068,1.);
#2938=VECTOR('',#23071,1.);
#2939=VECTOR('',#23074,1.);
#2940=VECTOR('',#23109,1.);
#2941=VECTOR('',#23112,1.);
#2942=VECTOR('',#23117,1.);
#2943=VECTOR('',#23120,1.);
#2944=VECTOR('',#23129,0.005);
#2945=VECTOR('',#23138,1.);
#2946=VECTOR('',#23141,1.);
#2947=VECTOR('',#23146,1.);
#2948=VECTOR('',#23147,1.);
#2949=VECTOR('',#23148,1.);
#2950=VECTOR('',#23151,1.);
#2951=VECTOR('',#23154,1.);
#2952=VECTOR('',#23159,1.);
#2953=VECTOR('',#23160,1.);
#2954=VECTOR('',#23161,1.);
#2955=VECTOR('',#23170,1.);
#2956=VECTOR('',#23173,1.);
#2957=VECTOR('',#23174,1.);
#2958=VECTOR('',#23177,1.);
#2959=VECTOR('',#23180,1.);
#2960=VECTOR('',#23183,1.);
#2961=VECTOR('',#23192,1.);
#2962=VECTOR('',#23195,1.);
#2963=VECTOR('',#23198,1.);
#2964=VECTOR('',#23201,1.);
#2965=VECTOR('',#23208,1.);
#2966=VECTOR('',#23211,1.);
#2967=VECTOR('',#23256,0.009);
#2968=VECTOR('',#23263,1.);
#2969=VECTOR('',#23264,0.01);
#2970=VECTOR('',#23265,1.);
#2971=VECTOR('',#23266,1.);
#2972=VECTOR('',#23267,1.);
#2973=VECTOR('',#23272,1.);
#2974=VECTOR('',#23273,0.01);
#2975=VECTOR('',#23274,1.);
#2976=VECTOR('',#23277,1.);
#2977=VECTOR('',#23278,1.);
#2978=VECTOR('',#23279,0.01);
#2979=VECTOR('',#23280,0.01);
#2980=VECTOR('',#23299,1.);
#2981=VECTOR('',#23302,1.);
#2982=VECTOR('',#23305,1.);
#2983=VECTOR('',#23312,1.);
#2984=VECTOR('',#23315,1.);
#2985=VECTOR('',#23316,1.);
#2986=VECTOR('',#23319,1.);
#2987=VECTOR('',#23320,1.);
#2988=VECTOR('',#23329,1.);
#2989=VECTOR('',#23332,1.);
#2990=VECTOR('',#23337,1.);
#2991=VECTOR('',#23338,1.);
#2992=VECTOR('',#23339,1.);
#2993=VECTOR('',#23342,1.);
#2994=VECTOR('',#23343,1.);
#2995=VECTOR('',#23344,1.);
#2996=VECTOR('',#23663,0.0005);
#2997=VECTOR('',#23666,0.0005);
#2998=VECTOR('',#23669,0.0005);
#2999=VECTOR('',#23672,0.0005);
#3425=CYLINDRICAL_SURFACE('',#19294,0.0125);
#3426=CYLINDRICAL_SURFACE('',#19298,0.001);
#3427=CYLINDRICAL_SURFACE('',#19301,0.0132323601801219);
#3428=CYLINDRICAL_SURFACE('',#19304,0.0132323601801219);
#3429=CYLINDRICAL_SURFACE('',#19322,0.0125);
#3430=CYLINDRICAL_SURFACE('',#19324,0.0125);
#3431=CYLINDRICAL_SURFACE('',#19327,0.005);
#3432=CYLINDRICAL_SURFACE('',#19334,0.0165);
#3433=CYLINDRICAL_SURFACE('',#19338,0.0165);
#3434=CYLINDRICAL_SURFACE('',#19342,0.0165);
#3435=CYLINDRICAL_SURFACE('',#19359,0.0135);
#3436=CYLINDRICAL_SURFACE('',#19362,0.0135);
#3437=CYLINDRICAL_SURFACE('',#19380,0.009);
#3438=CYLINDRICAL_SURFACE('',#19396,0.0132323601801219);
#3439=CYLINDRICAL_SURFACE('',#19399,0.0015);
#3440=CYLINDRICAL_SURFACE('',#19401,0.0015);
#3441=CYLINDRICAL_SURFACE('',#19408,0.0025);
#3442=CYLINDRICAL_SURFACE('',#19427,0.0002);
#3443=CYLINDRICAL_SURFACE('',#19433,0.0002);
#3444=CYLINDRICAL_SURFACE('',#19446,0.0002);
#3445=CYLINDRICAL_SURFACE('',#19447,0.0002);
#3446=CYLINDRICAL_SURFACE('',#19459,0.0002);
#3447=CYLINDRICAL_SURFACE('',#19463,0.0002);
#3448=CYLINDRICAL_SURFACE('',#19465,0.0002);
#3449=CYLINDRICAL_SURFACE('',#19467,0.0002);
#3450=CYLINDRICAL_SURFACE('',#19477,0.0002);
#3451=CYLINDRICAL_SURFACE('',#19481,0.0002);
#3452=CYLINDRICAL_SURFACE('',#19483,0.0002);
#3453=CYLINDRICAL_SURFACE('',#19491,0.0002);
#3454=CYLINDRICAL_SURFACE('',#19493,0.0002);
#3455=CYLINDRICAL_SURFACE('',#19495,0.0002);
#3456=CYLINDRICAL_SURFACE('',#19497,0.0002);
#3457=CYLINDRICAL_SURFACE('',#19502,0.0002);
#3458=CYLINDRICAL_SURFACE('',#19509,0.0002);
#3459=CYLINDRICAL_SURFACE('',#19516,0.0002);
#3460=CYLINDRICAL_SURFACE('',#19521,0.0002);
#3461=CYLINDRICAL_SURFACE('',#19523,0.0002);
#3462=CYLINDRICAL_SURFACE('',#19541,0.0002);
#3463=CYLINDRICAL_SURFACE('',#19544,0.0002);
#3464=CYLINDRICAL_SURFACE('',#19551,0.00199545322288878);
#3465=CYLINDRICAL_SURFACE('',#19553,0.0017588879999111);
#3466=CYLINDRICAL_SURFACE('',#19557,0.000202286544194825);
#3467=CYLINDRICAL_SURFACE('',#19558,0.000203651032597172);
#3468=CYLINDRICAL_SURFACE('',#19562,0.0019892004500739);
#3469=CYLINDRICAL_SURFACE('',#19564,0.00197736746715445);
#3470=CYLINDRICAL_SURFACE('',#19566,0.00199576483991537);
#3471=CYLINDRICAL_SURFACE('',#19570,0.000200921696200641);
#3472=CYLINDRICAL_SURFACE('',#19571,0.0005);
#3473=CYLINDRICAL_SURFACE('',#19572,0.0005);
#3474=CYLINDRICAL_SURFACE('',#19573,0.0005);
#3475=CYLINDRICAL_SURFACE('',#19574,0.0005);
#3524=FACE_BOUND('',#5453,.T.);
#3525=FACE_BOUND('',#5454,.T.);
#3526=FACE_BOUND('',#5455,.T.);
#3527=FACE_BOUND('',#5456,.T.);
#3528=FACE_BOUND('',#5457,.T.);
#3529=FACE_BOUND('',#5461,.T.);
#3530=FACE_BOUND('',#5462,.T.);
#3531=FACE_BOUND('',#5463,.T.);
#3532=FACE_BOUND('',#5464,.T.);
#3533=FACE_BOUND('',#5465,.T.);
#3534=FACE_BOUND('',#5472,.T.);
#3535=FACE_BOUND('',#5473,.T.);
#3536=FACE_BOUND('',#5474,.T.);
#3537=FACE_BOUND('',#5476,.T.);
#3538=FACE_BOUND('',#5480,.T.);
#3539=FACE_BOUND('',#5482,.T.);
#3540=FACE_BOUND('',#5501,.T.);
#3541=FACE_BOUND('',#5502,.T.);
#3542=FACE_BOUND('',#5503,.T.);
#4390=FACE_OUTER_BOUND('',#5443,.T.);
#4391=FACE_OUTER_BOUND('',#5444,.T.);
#4392=FACE_OUTER_BOUND('',#5445,.T.);
#4393=FACE_OUTER_BOUND('',#5446,.T.);
#4394=FACE_OUTER_BOUND('',#5447,.T.);
#4395=FACE_OUTER_BOUND('',#5448,.T.);
#4396=FACE_OUTER_BOUND('',#5449,.T.);
#4397=FACE_OUTER_BOUND('',#5450,.T.);
#4398=FACE_OUTER_BOUND('',#5451,.T.);
#4399=FACE_OUTER_BOUND('',#5452,.T.);
#4400=FACE_OUTER_BOUND('',#5458,.T.);
#4401=FACE_OUTER_BOUND('',#5459,.T.);
#4402=FACE_OUTER_BOUND('',#5460,.T.);
#4403=FACE_OUTER_BOUND('',#5466,.T.);
#4404=FACE_OUTER_BOUND('',#5467,.T.);
#4405=FACE_OUTER_BOUND('',#5468,.T.);
#4406=FACE_OUTER_BOUND('',#5469,.T.);
#4407=FACE_OUTER_BOUND('',#5470,.T.);
#4408=FACE_OUTER_BOUND('',#5471,.T.);
#4409=FACE_OUTER_BOUND('',#5475,.T.);
#4410=FACE_OUTER_BOUND('',#5477,.T.);
#4411=FACE_OUTER_BOUND('',#5478,.T.);
#4412=FACE_OUTER_BOUND('',#5479,.T.);
#4413=FACE_OUTER_BOUND('',#5481,.T.);
#4414=FACE_OUTER_BOUND('',#5483,.T.);
#4415=FACE_OUTER_BOUND('',#5484,.T.);
#4416=FACE_OUTER_BOUND('',#5485,.T.);
#4417=FACE_OUTER_BOUND('',#5486,.T.);
#4418=FACE_OUTER_BOUND('',#5487,.T.);
#4419=FACE_OUTER_BOUND('',#5488,.T.);
#4420=FACE_OUTER_BOUND('',#5489,.T.);
#4421=FACE_OUTER_BOUND('',#5490,.T.);
#4422=FACE_OUTER_BOUND('',#5491,.T.);
#4423=FACE_OUTER_BOUND('',#5492,.T.);
#4424=FACE_OUTER_BOUND('',#5493,.T.);
#4425=FACE_OUTER_BOUND('',#5494,.T.);
#4426=FACE_OUTER_BOUND('',#5495,.T.);
#4427=FACE_OUTER_BOUND('',#5496,.T.);
#4428=FACE_OUTER_BOUND('',#5497,.T.);
#4429=FACE_OUTER_BOUND('',#5498,.T.);
#4430=FACE_OUTER_BOUND('',#5499,.T.);
#4431=FACE_OUTER_BOUND('',#5500,.T.);
#4432=FACE_OUTER_BOUND('',#5504,.T.);
#4433=FACE_OUTER_BOUND('',#5505,.T.);
#4434=FACE_OUTER_BOUND('',#5506,.T.);
#4435=FACE_OUTER_BOUND('',#5507,.T.);
#4436=FACE_OUTER_BOUND('',#5508,.T.);
#4437=FACE_OUTER_BOUND('',#5509,.T.);
#4438=FACE_OUTER_BOUND('',#5510,.T.);
#4439=FACE_OUTER_BOUND('',#5511,.T.);
#4440=FACE_OUTER_BOUND('',#5512,.T.);
#4441=FACE_OUTER_BOUND('',#5513,.T.);
#4442=FACE_OUTER_BOUND('',#5514,.T.);
#4443=FACE_OUTER_BOUND('',#5515,.T.);
#4444=FACE_OUTER_BOUND('',#5516,.T.);
#4445=FACE_OUTER_BOUND('',#5517,.T.);
#4446=FACE_OUTER_BOUND('',#5518,.T.);
#4447=FACE_OUTER_BOUND('',#5519,.T.);
#4448=FACE_OUTER_BOUND('',#5520,.T.);
#4449=FACE_OUTER_BOUND('',#5521,.T.);
#4450=FACE_OUTER_BOUND('',#5522,.T.);
#4451=FACE_OUTER_BOUND('',#5523,.T.);
#4452=FACE_OUTER_BOUND('',#5524,.T.);
#4453=FACE_OUTER_BOUND('',#5525,.T.);
#4454=FACE_OUTER_BOUND('',#5526,.T.);
#4455=FACE_OUTER_BOUND('',#5527,.T.);
#4456=FACE_OUTER_BOUND('',#5528,.T.);
#4457=FACE_OUTER_BOUND('',#5529,.T.);
#4458=FACE_OUTER_BOUND('',#5530,.T.);
#4459=FACE_OUTER_BOUND('',#5531,.T.);
#4460=FACE_OUTER_BOUND('',#5532,.T.);
#4461=FACE_OUTER_BOUND('',#5533,.T.);
#4462=FACE_OUTER_BOUND('',#5534,.T.);
#4463=FACE_OUTER_BOUND('',#5535,.T.);
#4464=FACE_OUTER_BOUND('',#5536,.T.);
#4465=FACE_OUTER_BOUND('',#5537,.T.);
#4466=FACE_OUTER_BOUND('',#5538,.T.);
#4467=FACE_OUTER_BOUND('',#5539,.T.);
#4468=FACE_OUTER_BOUND('',#5540,.T.);
#4469=FACE_OUTER_BOUND('',#5541,.T.);
#4470=FACE_OUTER_BOUND('',#5542,.T.);
#4471=FACE_OUTER_BOUND('',#5543,.T.);
#4472=FACE_OUTER_BOUND('',#5544,.T.);
#4473=FACE_OUTER_BOUND('',#5545,.T.);
#4474=FACE_OUTER_BOUND('',#5546,.T.);
#4475=FACE_OUTER_BOUND('',#5547,.T.);
#4476=FACE_OUTER_BOUND('',#5548,.T.);
#4477=FACE_OUTER_BOUND('',#5549,.T.);
#4478=FACE_OUTER_BOUND('',#5550,.T.);
#4479=FACE_OUTER_BOUND('',#5551,.T.);
#4480=FACE_OUTER_BOUND('',#5552,.T.);
#4481=FACE_OUTER_BOUND('',#5553,.T.);
#4482=FACE_OUTER_BOUND('',#5554,.T.);
#4483=FACE_OUTER_BOUND('',#5555,.T.);
#4484=FACE_OUTER_BOUND('',#5556,.T.);
#4485=FACE_OUTER_BOUND('',#5557,.T.);
#4486=FACE_OUTER_BOUND('',#5558,.T.);
#4487=FACE_OUTER_BOUND('',#5559,.T.);
#4488=FACE_OUTER_BOUND('',#5560,.T.);
#4489=FACE_OUTER_BOUND('',#5561,.T.);
#4490=FACE_OUTER_BOUND('',#5562,.T.);
#4491=FACE_OUTER_BOUND('',#5563,.T.);
#4492=FACE_OUTER_BOUND('',#5564,.T.);
#4493=FACE_OUTER_BOUND('',#5565,.T.);
#4494=FACE_OUTER_BOUND('',#5566,.T.);
#4495=FACE_OUTER_BOUND('',#5567,.T.);
#4496=FACE_OUTER_BOUND('',#5568,.T.);
#4497=FACE_OUTER_BOUND('',#5569,.T.);
#4498=FACE_OUTER_BOUND('',#5570,.T.);
#4499=FACE_OUTER_BOUND('',#5571,.T.);
#4500=FACE_OUTER_BOUND('',#5572,.T.);
#4501=FACE_OUTER_BOUND('',#5573,.T.);
#4502=FACE_OUTER_BOUND('',#5574,.T.);
#4503=FACE_OUTER_BOUND('',#5575,.T.);
#4504=FACE_OUTER_BOUND('',#5576,.T.);
#4505=FACE_OUTER_BOUND('',#5577,.T.);
#4506=FACE_OUTER_BOUND('',#5578,.T.);
#4507=FACE_OUTER_BOUND('',#5579,.T.);
#4508=FACE_OUTER_BOUND('',#5580,.T.);
#4509=FACE_OUTER_BOUND('',#5581,.T.);
#4510=FACE_OUTER_BOUND('',#5582,.T.);
#4511=FACE_OUTER_BOUND('',#5583,.T.);
#4512=FACE_OUTER_BOUND('',#5584,.T.);
#4513=FACE_OUTER_BOUND('',#5585,.T.);
#4514=FACE_OUTER_BOUND('',#5586,.T.);
#4515=FACE_OUTER_BOUND('',#5587,.T.);
#4516=FACE_OUTER_BOUND('',#5588,.T.);
#4517=FACE_OUTER_BOUND('',#5589,.T.);
#4518=FACE_OUTER_BOUND('',#5590,.T.);
#4519=FACE_OUTER_BOUND('',#5591,.T.);
#4520=FACE_OUTER_BOUND('',#5592,.T.);
#4521=FACE_OUTER_BOUND('',#5593,.T.);
#4522=FACE_OUTER_BOUND('',#5594,.T.);
#4523=FACE_OUTER_BOUND('',#5595,.T.);
#4524=FACE_OUTER_BOUND('',#5596,.T.);
#4525=FACE_OUTER_BOUND('',#5597,.T.);
#4526=FACE_OUTER_BOUND('',#5598,.T.);
#4527=FACE_OUTER_BOUND('',#5599,.T.);
#4528=FACE_OUTER_BOUND('',#5600,.T.);
#4529=FACE_OUTER_BOUND('',#5601,.T.);
#4530=FACE_OUTER_BOUND('',#5602,.T.);
#4531=FACE_OUTER_BOUND('',#5603,.T.);
#4532=FACE_OUTER_BOUND('',#5604,.T.);
#4533=FACE_OUTER_BOUND('',#5605,.T.);
#4534=FACE_OUTER_BOUND('',#5606,.T.);
#4535=FACE_OUTER_BOUND('',#5607,.T.);
#4536=FACE_OUTER_BOUND('',#5608,.T.);
#4537=FACE_OUTER_BOUND('',#5609,.T.);
#4538=FACE_OUTER_BOUND('',#5610,.T.);
#4539=FACE_OUTER_BOUND('',#5611,.T.);
#4540=FACE_OUTER_BOUND('',#5612,.T.);
#4541=FACE_OUTER_BOUND('',#5613,.T.);
#4542=FACE_OUTER_BOUND('',#5614,.T.);
#4543=FACE_OUTER_BOUND('',#5615,.T.);
#4544=FACE_OUTER_BOUND('',#5616,.T.);
#4545=FACE_OUTER_BOUND('',#5617,.T.);
#5443=EDGE_LOOP('',(#15753,#15754,#15755,#15756,#15757,#15758,#15759,#15760,
#15761,#15762));
#5444=EDGE_LOOP('',(#15763,#15764,#15765,#15766,#15767,#15768,#15769,#15770,
#15771,#15772));
#5445=EDGE_LOOP('',(#15773,#15774,#15775,#15776,#15777,#15778,#15779,#15780,
#15781,#15782));
#5446=EDGE_LOOP('',(#15783,#15784,#15785,#15786,#15787,#15788,#15789,#15790,
#15791,#15792));
#5447=EDGE_LOOP('',(#15793,#15794,#15795,#15796,#15797,#15798,#15799,#15800,
#15801,#15802));
#5448=EDGE_LOOP('',(#15803,#15804,#15805,#15806,#15807,#15808));
#5449=EDGE_LOOP('',(#15809,#15810,#15811,#15812));
#5450=EDGE_LOOP('',(#15813,#15814,#15815,#15816));
#5451=EDGE_LOOP('',(#15817,#15818,#15819,#15820));
#5452=EDGE_LOOP('',(#15821,#15822,#15823,#15824,#15825,#15826,#15827,#15828,
#15829,#15830));
#5453=EDGE_LOOP('',(#15831));
#5454=EDGE_LOOP('',(#15832));
#5455=EDGE_LOOP('',(#15833));
#5456=EDGE_LOOP('',(#15834));
#5457=EDGE_LOOP('',(#15835));
#5458=EDGE_LOOP('',(#15836,#15837,#15838,#15839,#15840,#15841));
#5459=EDGE_LOOP('',(#15842,#15843,#15844,#15845));
#5460=EDGE_LOOP('',(#15846,#15847,#15848,#15849,#15850,#15851,#15852,#15853,
#15854,#15855));
#5461=EDGE_LOOP('',(#15856,#15857));
#5462=EDGE_LOOP('',(#15858,#15859));
#5463=EDGE_LOOP('',(#15860,#15861));
#5464=EDGE_LOOP('',(#15862,#15863));
#5465=EDGE_LOOP('',(#15864,#15865));
#5466=EDGE_LOOP('',(#15866,#15867,#15868,#15869));
#5467=EDGE_LOOP('',(#15870,#15871,#15872,#15873));
#5468=EDGE_LOOP('',(#15874,#15875,#15876,#15877));
#5469=EDGE_LOOP('',(#15878,#15879,#15880,#15881));
#5470=EDGE_LOOP('',(#15882,#15883,#15884,#15885));
#5471=EDGE_LOOP('',(#15886,#15887,#15888,#15889,#15890,#15891,#15892,#15893,
#15894,#15895));
#5472=EDGE_LOOP('',(#15896));
#5473=EDGE_LOOP('',(#15897));
#5474=EDGE_LOOP('',(#15898));
#5475=EDGE_LOOP('',(#15899,#15900,#15901,#15902,#15903,#15904,#15905,#15906,
#15907,#15908,#15909,#15910));
#5476=EDGE_LOOP('',(#15911,#15912));
#5477=EDGE_LOOP('',(#15913,#15914,#15915,#15916));
#5478=EDGE_LOOP('',(#15917,#15918,#15919,#15920));
#5479=EDGE_LOOP('',(#15921,#15922));
#5480=EDGE_LOOP('',(#15923,#15924,#15925,#15926,#15927,#15928,#15929,#15930,
#15931,#15932,#15933,#15934));
#5481=EDGE_LOOP('',(#15935));
#5482=EDGE_LOOP('',(#15936));
#5483=EDGE_LOOP('',(#15937,#15938,#15939,#15940,#15941,#15942));
#5484=EDGE_LOOP('',(#15943,#15944,#15945,#15946,#15947,#15948,#15949,#15950,
#15951,#15952));
#5485=EDGE_LOOP('',(#15953,#15954,#15955,#15956,#15957,#15958,#15959,#15960,
#15961,#15962,#15963));
#5486=EDGE_LOOP('',(#15964,#15965,#15966,#15967,#15968,#15969));
#5487=EDGE_LOOP('',(#15970,#15971,#15972,#15973,#15974,#15975));
#5488=EDGE_LOOP('',(#15976,#15977,#15978,#15979,#15980,#15981,#15982));
#5489=EDGE_LOOP('',(#15983,#15984,#15985,#15986,#15987,#15988,#15989,#15990,
#15991));
#5490=EDGE_LOOP('',(#15992,#15993,#15994,#15995,#15996));
#5491=EDGE_LOOP('',(#15997));
#5492=EDGE_LOOP('',(#15998,#15999,#16000,#16001,#16002,#16003,#16004,#16005));
#5493=EDGE_LOOP('',(#16006,#16007,#16008,#16009,#16010,#16011,#16012,#16013));
#5494=EDGE_LOOP('',(#16014,#16015,#16016,#16017,#16018,#16019,#16020,#16021));
#5495=EDGE_LOOP('',(#16022,#16023,#16024,#16025,#16026,#16027,#16028,#16029));
#5496=EDGE_LOOP('',(#16030,#16031,#16032,#16033,#16034,#16035,#16036,#16037));
#5497=EDGE_LOOP('',(#16038,#16039,#16040,#16041));
#5498=EDGE_LOOP('',(#16042,#16043,#16044,#16045));
#5499=EDGE_LOOP('',(#16046,#16047,#16048,#16049));
#5500=EDGE_LOOP('',(#16050,#16051,#16052,#16053,#16054,#16055,#16056,#16057,
#16058,#16059,#16060,#16061));
#5501=EDGE_LOOP('',(#16062));
#5502=EDGE_LOOP('',(#16063));
#5503=EDGE_LOOP('',(#16064));
#5504=EDGE_LOOP('',(#16065,#16066,#16067,#16068));
#5505=EDGE_LOOP('',(#16069,#16070,#16071,#16072));
#5506=EDGE_LOOP('',(#16073,#16074,#16075,#16076));
#5507=EDGE_LOOP('',(#16077,#16078,#16079,#16080,#16081));
#5508=EDGE_LOOP('',(#16082,#16083,#16084,#16085));
#5509=EDGE_LOOP('',(#16086,#16087,#16088,#16089,#16090));
#5510=EDGE_LOOP('',(#16091,#16092,#16093,#16094,#16095,#16096));
#5511=EDGE_LOOP('',(#16097,#16098,#16099,#16100));
#5512=EDGE_LOOP('',(#16101,#16102,#16103,#16104,#16105,#16106));
#5513=EDGE_LOOP('',(#16107,#16108,#16109,#16110,#16111,#16112));
#5514=EDGE_LOOP('',(#16113,#16114,#16115));
#5515=EDGE_LOOP('',(#16116,#16117,#16118,#16119,#16120,#16121,#16122));
#5516=EDGE_LOOP('',(#16123,#16124,#16125));
#5517=EDGE_LOOP('',(#16126,#16127,#16128,#16129,#16130,#16131,#16132));
#5518=EDGE_LOOP('',(#16133,#16134,#16135));
#5519=EDGE_LOOP('',(#16136,#16137,#16138));
#5520=EDGE_LOOP('',(#16139,#16140,#16141,#16142,#16143,#16144));
#5521=EDGE_LOOP('',(#16145,#16146,#16147,#16148));
#5522=EDGE_LOOP('',(#16149,#16150,#16151,#16152));
#5523=EDGE_LOOP('',(#16153,#16154,#16155,#16156));
#5524=EDGE_LOOP('',(#16157,#16158,#16159,#16160));
#5525=EDGE_LOOP('',(#16161,#16162,#16163,#16164));
#5526=EDGE_LOOP('',(#16165,#16166,#16167,#16168,#16169));
#5527=EDGE_LOOP('',(#16170,#16171,#16172,#16173));
#5528=EDGE_LOOP('',(#16174,#16175,#16176,#16177));
#5529=EDGE_LOOP('',(#16178,#16179,#16180,#16181));
#5530=EDGE_LOOP('',(#16182,#16183,#16184,#16185));
#5531=EDGE_LOOP('',(#16186,#16187,#16188,#16189));
#5532=EDGE_LOOP('',(#16190,#16191,#16192,#16193,#16194));
#5533=EDGE_LOOP('',(#16195,#16196,#16197,#16198,#16199));
#5534=EDGE_LOOP('',(#16200,#16201,#16202,#16203));
#5535=EDGE_LOOP('',(#16204,#16205,#16206,#16207));
#5536=EDGE_LOOP('',(#16208,#16209,#16210,#16211));
#5537=EDGE_LOOP('',(#16212,#16213,#16214,#16215));
#5538=EDGE_LOOP('',(#16216,#16217,#16218,#16219));
#5539=EDGE_LOOP('',(#16220,#16221,#16222,#16223));
#5540=EDGE_LOOP('',(#16224,#16225,#16226,#16227,#16228));
#5541=EDGE_LOOP('',(#16229,#16230,#16231,#16232,#16233,#16234,#16235));
#5542=EDGE_LOOP('',(#16236,#16237,#16238,#16239));
#5543=EDGE_LOOP('',(#16240,#16241,#16242,#16243));
#5544=EDGE_LOOP('',(#16244,#16245,#16246,#16247));
#5545=EDGE_LOOP('',(#16248,#16249,#16250,#16251));
#5546=EDGE_LOOP('',(#16252,#16253,#16254,#16255));
#5547=EDGE_LOOP('',(#16256,#16257,#16258,#16259));
#5548=EDGE_LOOP('',(#16260,#16261,#16262));
#5549=EDGE_LOOP('',(#16263,#16264,#16265,#16266));
#5550=EDGE_LOOP('',(#16267,#16268,#16269,#16270,#16271,#16272,#16273));
#5551=EDGE_LOOP('',(#16274,#16275,#16276,#16277));
#5552=EDGE_LOOP('',(#16278,#16279,#16280,#16281));
#5553=EDGE_LOOP('',(#16282,#16283,#16284,#16285));
#5554=EDGE_LOOP('',(#16286,#16287,#16288,#16289));
#5555=EDGE_LOOP('',(#16290,#16291,#16292,#16293));
#5556=EDGE_LOOP('',(#16294,#16295,#16296,#16297));
#5557=EDGE_LOOP('',(#16298,#16299,#16300,#16301));
#5558=EDGE_LOOP('',(#16302,#16303,#16304,#16305,#16306));
#5559=EDGE_LOOP('',(#16307,#16308,#16309,#16310));
#5560=EDGE_LOOP('',(#16311,#16312,#16313,#16314));
#5561=EDGE_LOOP('',(#16315,#16316,#16317,#16318));
#5562=EDGE_LOOP('',(#16319,#16320,#16321));
#5563=EDGE_LOOP('',(#16322,#16323,#16324,#16325));
#5564=EDGE_LOOP('',(#16326,#16327,#16328,#16329,#16330,#16331));
#5565=EDGE_LOOP('',(#16332,#16333,#16334,#16335,#16336));
#5566=EDGE_LOOP('',(#16337,#16338,#16339,#16340));
#5567=EDGE_LOOP('',(#16341,#16342,#16343,#16344,#16345));
#5568=EDGE_LOOP('',(#16346,#16347,#16348,#16349,#16350));
#5569=EDGE_LOOP('',(#16351,#16352,#16353,#16354));
#5570=EDGE_LOOP('',(#16355,#16356,#16357,#16358));
#5571=EDGE_LOOP('',(#16359,#16360,#16361,#16362));
#5572=EDGE_LOOP('',(#16363,#16364,#16365,#16366,#16367));
#5573=EDGE_LOOP('',(#16368,#16369,#16370,#16371));
#5574=EDGE_LOOP('',(#16372,#16373,#16374,#16375));
#5575=EDGE_LOOP('',(#16376,#16377,#16378,#16379));
#5576=EDGE_LOOP('',(#16380,#16381,#16382,#16383,#16384));
#5577=EDGE_LOOP('',(#16385,#16386,#16387,#16388));
#5578=EDGE_LOOP('',(#16389,#16390,#16391,#16392));
#5579=EDGE_LOOP('',(#16393,#16394,#16395,#16396));
#5580=EDGE_LOOP('',(#16397,#16398,#16399,#16400,#16401));
#5581=EDGE_LOOP('',(#16402,#16403,#16404,#16405));
#5582=EDGE_LOOP('',(#16406,#16407,#16408));
#5583=EDGE_LOOP('',(#16409,#16410,#16411,#16412));
#5584=EDGE_LOOP('',(#16413,#16414,#16415));
#5585=EDGE_LOOP('',(#16416,#16417,#16418));
#5586=EDGE_LOOP('',(#16419,#16420,#16421,#16422));
#5587=EDGE_LOOP('',(#16423,#16424,#16425,#16426));
#5588=EDGE_LOOP('',(#16427,#16428,#16429,#16430));
#5589=EDGE_LOOP('',(#16431,#16432,#16433,#16434));
#5590=EDGE_LOOP('',(#16435,#16436,#16437,#16438,#16439));
#5591=EDGE_LOOP('',(#16440,#16441,#16442,#16443));
#5592=EDGE_LOOP('',(#16444,#16445,#16446,#16447));
#5593=EDGE_LOOP('',(#16448,#16449,#16450,#16451));
#5594=EDGE_LOOP('',(#16452,#16453,#16454,#16455));
#5595=EDGE_LOOP('',(#16456,#16457,#16458,#16459));
#5596=EDGE_LOOP('',(#16460,#16461,#16462));
#5597=EDGE_LOOP('',(#16463,#16464,#16465,#16466));
#5598=EDGE_LOOP('',(#16467,#16468,#16469,#16470));
#5599=EDGE_LOOP('',(#16471,#16472,#16473,#16474));
#5600=EDGE_LOOP('',(#16475,#16476,#16477,#16478));
#5601=EDGE_LOOP('',(#16479,#16480,#16481,#16482));
#5602=EDGE_LOOP('',(#16483,#16484,#16485,#16486));
#5603=EDGE_LOOP('',(#16487,#16488,#16489));
#5604=EDGE_LOOP('',(#16490,#16491,#16492));
#5605=EDGE_LOOP('',(#16493,#16494,#16495,#16496));
#5606=EDGE_LOOP('',(#16497,#16498,#16499,#16500));
#5607=EDGE_LOOP('',(#16501,#16502,#16503,#16504));
#5608=EDGE_LOOP('',(#16505,#16506,#16507,#16508));
#5609=EDGE_LOOP('',(#16509,#16510,#16511,#16512));
#5610=EDGE_LOOP('',(#16513,#16514,#16515,#16516));
#5611=EDGE_LOOP('',(#16517,#16518,#16519,#16520));
#5612=EDGE_LOOP('',(#16521,#16522,#16523));
#5613=EDGE_LOOP('',(#16524,#16525,#16526,#16527));
#5614=EDGE_LOOP('',(#16528,#16529,#16530,#16531));
#5615=EDGE_LOOP('',(#16532,#16533,#16534,#16535));
#5616=EDGE_LOOP('',(#16536,#16537,#16538,#16539));
#5617=EDGE_LOOP('',(#16540,#16541,#16542,#16543,#16544));
#6360=CIRCLE('',#19295,0.0125);
#6361=CIRCLE('',#19296,0.0125);
#6362=CIRCLE('',#19297,0.0125);
#6363=CIRCLE('',#19299,0.001);
#6364=CIRCLE('',#19300,0.001);
#6365=CIRCLE('',#19302,0.0132323601801219);
#6366=CIRCLE('',#19303,0.0132323601801219);
#6367=CIRCLE('',#19305,0.0132323601801219);
#6368=CIRCLE('',#19306,0.0132323601801219);
#6369=CIRCLE('',#19308,0.0123);
#6370=CIRCLE('',#19309,0.0127);
#6371=CIRCLE('',#19310,0.0125);
#6372=CIRCLE('',#19311,0.0130323601801219);
#6373=CIRCLE('',#19312,0.0004);
#6374=CIRCLE('',#19313,0.0013);
#6375=CIRCLE('',#19314,0.0130323601801219);
#6376=CIRCLE('',#19315,0.0013);
#6377=CIRCLE('',#19316,0.0004);
#6378=CIRCLE('',#19317,0.0130323601801219);
#6379=CIRCLE('',#19318,0.0005);
#6380=CIRCLE('',#19319,0.0005);
#6381=CIRCLE('',#19320,0.0005);
#6382=CIRCLE('',#19321,0.0005);
#6383=CIRCLE('',#19323,0.0125);
#6384=CIRCLE('',#19325,0.0125);
#6385=CIRCLE('',#19326,0.0125);
#6386=CIRCLE('',#19328,0.00500000000000001);
#6387=CIRCLE('',#19329,0.005);
#6388=CIRCLE('',#19330,0.005);
#6389=CIRCLE('',#19331,0.005);
#6390=CIRCLE('',#19332,0.005);
#6391=CIRCLE('',#19333,0.005);
#6392=CIRCLE('',#19335,0.0165);
#6393=CIRCLE('',#19336,0.0165);
#6394=CIRCLE('',#19339,0.0165);
#6395=CIRCLE('',#19340,0.0165);
#6396=CIRCLE('',#19343,0.0165);
#6397=CIRCLE('',#19344,0.0165);
#6398=CIRCLE('',#19346,0.0027);
#6399=CIRCLE('',#19347,0.0163);
#6400=CIRCLE('',#19348,0.0163);
#6401=CIRCLE('',#19349,0.0163);
#6402=CIRCLE('',#19350,0.0005);
#6403=CIRCLE('',#19351,0.0005);
#6404=CIRCLE('',#19352,0.0092);
#6405=CIRCLE('',#19354,0.0163);
#6406=CIRCLE('',#19355,0.0163);
#6407=CIRCLE('',#19356,0.0163);
#6408=CIRCLE('',#19357,0.0137);
#6409=CIRCLE('',#19358,0.0137);
#6410=CIRCLE('',#19360,0.0135);
#6411=CIRCLE('',#19361,0.0135);
#6412=CIRCLE('',#19363,0.0135);
#6413=CIRCLE('',#19364,0.0135);
#6414=CIRCLE('',#19366,0.0127);
#6415=CIRCLE('',#19367,0.0127);
#6416=CIRCLE('',#19368,0.0127);
#6417=CIRCLE('',#19369,0.0004);
#6418=CIRCLE('',#19370,0.0134323601801219);
#6419=CIRCLE('',#19371,0.0002);
#6420=CIRCLE('',#19372,0.0015);
#6421=CIRCLE('',#19373,0.0015);
#6422=CIRCLE('',#19374,0.0002);
#6423=CIRCLE('',#19375,0.0134323601801219);
#6424=CIRCLE('',#19376,0.0004);
#6425=CIRCLE('',#19378,0.0123);
#6426=CIRCLE('',#19379,0.0092);
#6427=CIRCLE('',#19381,0.009);
#6428=CIRCLE('',#19382,0.009);
#6429=CIRCLE('',#19383,0.009);
#6430=CIRCLE('',#19384,0.009);
#6431=CIRCLE('',#19390,0.004);
#6432=CIRCLE('',#19397,0.0132323601801219);
#6433=CIRCLE('',#19398,0.0132323601801219);
#6434=CIRCLE('',#19400,0.0015);
#6435=CIRCLE('',#19402,0.0015);
#6436=CIRCLE('',#19404,0.0023);
#6437=CIRCLE('',#19405,0.0012);
#6438=CIRCLE('',#19406,0.0005);
#6439=CIRCLE('',#19407,0.0005);
#6440=CIRCLE('',#19409,0.0025);
#6441=CIRCLE('',#19410,0.0025);
#6442=CIRCLE('',#19413,0.015);
#6443=CIRCLE('',#19414,0.015);
#6444=CIRCLE('',#19415,0.015);
#6445=CIRCLE('',#19416,0.015);
#6446=CIRCLE('',#19422,0.0002);
#6447=CIRCLE('',#19423,0.0002);
#6448=CIRCLE('',#19425,0.0002);
#6449=CIRCLE('',#19426,0.0002);
#6450=CIRCLE('',#19428,0.0002);
#6451=CIRCLE('',#19431,0.0002);
#6452=CIRCLE('',#19432,0.0002);
#6453=CIRCLE('',#19434,0.0002);
#6454=CIRCLE('',#19436,0.0002);
#6455=CIRCLE('',#19440,0.0002);
#6456=CIRCLE('',#19442,0.0002);
#6457=CIRCLE('',#19443,0.0002);
#6458=CIRCLE('',#19448,0.0002);
#6459=CIRCLE('',#19450,0.0002);
#6460=CIRCLE('',#19452,0.0002);
#6461=CIRCLE('',#19454,0.0002);
#6462=CIRCLE('',#19455,0.000199995253972718);
#6463=CIRCLE('',#19457,0.0002);
#6464=CIRCLE('',#19458,0.0002);
#6465=CIRCLE('',#19460,0.0002);
#6466=CIRCLE('',#19462,0.000200484899633866);
#6467=CIRCLE('',#19464,0.0002);
#6468=CIRCLE('',#19466,0.0002);
#6469=CIRCLE('',#19468,0.0002);
#6470=CIRCLE('',#19469,0.0002);
#6471=CIRCLE('',#19472,0.00017797030966603);
#6472=CIRCLE('',#19474,0.0002);
#6473=CIRCLE('',#19476,0.0002);
#6474=CIRCLE('',#19478,0.0002);
#6475=CIRCLE('',#19480,0.000199995408286236);
#6476=CIRCLE('',#19482,0.0002);
#6477=CIRCLE('',#19484,0.0002);
#6478=CIRCLE('',#19486,0.0002);
#6479=CIRCLE('',#19488,0.0002);
#6480=CIRCLE('',#19490,0.0002);
#6481=CIRCLE('',#19494,0.0002);
#6482=CIRCLE('',#19496,0.0002);
#6483=CIRCLE('',#19498,0.0002);
#6484=CIRCLE('',#19499,0.0002);
#6485=CIRCLE('',#19501,0.0002);
#6486=CIRCLE('',#19504,0.0125);
#6487=CIRCLE('',#19505,0.0002);
#6488=CIRCLE('',#19507,0.0002);
#6489=CIRCLE('',#19508,0.0002);
#6490=CIRCLE('',#19510,0.0002);
#6491=CIRCLE('',#19511,0.000200000000000081);
#6492=CIRCLE('',#19513,0.0002);
#6493=CIRCLE('',#19515,0.000199999999999959);
#6494=CIRCLE('',#19517,0.0002);
#6495=CIRCLE('',#19518,0.0002);
#6496=CIRCLE('',#19520,0.0002);
#6497=CIRCLE('',#19522,0.0002);
#6498=CIRCLE('',#19524,0.0002);
#6499=CIRCLE('',#19529,0.0002);
#6500=CIRCLE('',#19531,0.0002);
#6501=CIRCLE('',#19533,0.0002);
#6502=CIRCLE('',#19535,0.0002);
#6503=CIRCLE('',#19536,0.0002);
#6504=CIRCLE('',#19538,0.0002);
#6505=CIRCLE('',#19540,0.0002);
#6506=CIRCLE('',#19542,0.0002);
#6507=CIRCLE('',#19545,0.0002);
#6508=CIRCLE('',#19549,0.002);
#6509=CIRCLE('',#19550,0.00199565795815631);
#6510=CIRCLE('',#19552,0.00199545369122859);
#6511=CIRCLE('',#19554,0.00175917590714212);
#6512=CIRCLE('',#19555,0.002);
#6513=CIRCLE('',#19556,0.00199999989085889);
#6514=CIRCLE('',#19559,0.00199999684224345);
#6515=CIRCLE('',#19560,0.002);
#6516=CIRCLE('',#19561,0.00198947184167493);
#6517=CIRCLE('',#19563,0.00198949433969945);
#6518=CIRCLE('',#19565,0.00197761179274946);
#6519=CIRCLE('',#19567,0.00199597791916769);
#6520=CIRCLE('',#19568,0.002);
#6521=CIRCLE('',#19576,0.001);
#8073=VERTEX_POINT('',#49165);
#8074=VERTEX_POINT('',#49166);
#8075=VERTEX_POINT('',#49170);
#8076=VERTEX_POINT('',#49182);
#8077=VERTEX_POINT('',#49186);
#8078=VERTEX_POINT('',#49191);
#8079=VERTEX_POINT('',#49197);
#8080=VERTEX_POINT('',#49203);
#8081=VERTEX_POINT('',#49209);
#8082=VERTEX_POINT('',#49215);
#8083=VERTEX_POINT('',#49258);
#8084=VERTEX_POINT('',#49259);
#8085=VERTEX_POINT('',#49263);
#8086=VERTEX_POINT('',#49275);
#8087=VERTEX_POINT('',#49279);
#8088=VERTEX_POINT('',#49284);
#8089=VERTEX_POINT('',#49290);
#8090=VERTEX_POINT('',#49296);
#8091=VERTEX_POINT('',#49302);
#8092=VERTEX_POINT('',#49308);
#8093=VERTEX_POINT('',#49351);
#8094=VERTEX_POINT('',#49352);
#8095=VERTEX_POINT('',#49356);
#8096=VERTEX_POINT('',#49368);
#8097=VERTEX_POINT('',#49372);
#8098=VERTEX_POINT('',#49377);
#8099=VERTEX_POINT('',#49383);
#8100=VERTEX_POINT('',#49389);
#8101=VERTEX_POINT('',#49395);
#8102=VERTEX_POINT('',#49401);
#8103=VERTEX_POINT('',#49444);
#8104=VERTEX_POINT('',#49445);
#8105=VERTEX_POINT('',#49449);
#8106=VERTEX_POINT('',#49461);
#8107=VERTEX_POINT('',#49465);
#8108=VERTEX_POINT('',#49470);
#8109=VERTEX_POINT('',#49476);
#8110=VERTEX_POINT('',#49482);
#8111=VERTEX_POINT('',#49488);
#8112=VERTEX_POINT('',#49494);
#8113=VERTEX_POINT('',#49537);
#8114=VERTEX_POINT('',#49538);
#8115=VERTEX_POINT('',#49542);
#8116=VERTEX_POINT('',#49554);
#8117=VERTEX_POINT('',#49558);
#8118=VERTEX_POINT('',#49563);
#8119=VERTEX_POINT('',#49569);
#8120=VERTEX_POINT('',#49575);
#8121=VERTEX_POINT('',#49581);
#8122=VERTEX_POINT('',#49587);
#8123=VERTEX_POINT('',#49598);
#8124=VERTEX_POINT('',#49599);
#8125=VERTEX_POINT('',#49604);
#8126=VERTEX_POINT('',#49606);
#8127=VERTEX_POINT('',#49608);
#8128=VERTEX_POINT('',#49610);
#8129=VERTEX_POINT('',#49614);
#8130=VERTEX_POINT('',#49616);
#8131=VERTEX_POINT('',#49620);
#8132=VERTEX_POINT('',#49621);
#8133=VERTEX_POINT('',#49623);
#8134=VERTEX_POINT('',#49625);
#8135=VERTEX_POINT('',#49629);
#8136=VERTEX_POINT('',#49630);
#8137=VERTEX_POINT('',#49632);
#8138=VERTEX_POINT('',#49634);
#8139=VERTEX_POINT('',#49638);
#8140=VERTEX_POINT('',#49639);
#8141=VERTEX_POINT('',#49641);
#8142=VERTEX_POINT('',#49643);
#8143=VERTEX_POINT('',#49645);
#8144=VERTEX_POINT('',#49647);
#8145=VERTEX_POINT('',#49649);
#8146=VERTEX_POINT('',#49651);
#8147=VERTEX_POINT('',#49653);
#8148=VERTEX_POINT('',#49655);
#8149=VERTEX_POINT('',#49658);
#8150=VERTEX_POINT('',#49660);
#8151=VERTEX_POINT('',#49662);
#8152=VERTEX_POINT('',#49664);
#8153=VERTEX_POINT('',#49667);
#8154=VERTEX_POINT('',#49674);
#8155=VERTEX_POINT('',#49676);
#8156=VERTEX_POINT('',#49678);
#8157=VERTEX_POINT('',#49691);
#8158=VERTEX_POINT('',#49692);
#8159=VERTEX_POINT('',#49694);
#8160=VERTEX_POINT('',#49696);
#8161=VERTEX_POINT('',#49700);
#8162=VERTEX_POINT('',#49701);
#8163=VERTEX_POINT('',#49715);
#8164=VERTEX_POINT('',#49717);
#8165=VERTEX_POINT('',#49719);
#8166=VERTEX_POINT('',#49733);
#8167=VERTEX_POINT('',#49735);
#8168=VERTEX_POINT('',#49737);
#8169=VERTEX_POINT('',#49762);
#8170=VERTEX_POINT('',#49763);
#8171=VERTEX_POINT('',#49765);
#8172=VERTEX_POINT('',#49767);
#8173=VERTEX_POINT('',#49771);
#8174=VERTEX_POINT('',#49772);
#8175=VERTEX_POINT('',#49777);
#8176=VERTEX_POINT('',#49778);
#8177=VERTEX_POINT('',#49780);
#8178=VERTEX_POINT('',#49782);
#8179=VERTEX_POINT('',#49786);
#8180=VERTEX_POINT('',#49788);
#8181=VERTEX_POINT('',#49795);
#8182=VERTEX_POINT('',#49796);
#8183=VERTEX_POINT('',#49798);
#8184=VERTEX_POINT('',#49800);
#8185=VERTEX_POINT('',#49802);
#8186=VERTEX_POINT('',#49804);
#8187=VERTEX_POINT('',#49806);
#8188=VERTEX_POINT('',#49808);
#8189=VERTEX_POINT('',#49810);
#8190=VERTEX_POINT('',#49812);
#8191=VERTEX_POINT('',#49815);
#8192=VERTEX_POINT('',#49817);
#8193=VERTEX_POINT('',#49819);
#8194=VERTEX_POINT('',#49822);
#8195=VERTEX_POINT('',#49823);
#8196=VERTEX_POINT('',#49831);
#8197=VERTEX_POINT('',#49836);
#8198=VERTEX_POINT('',#49838);
#8199=VERTEX_POINT('',#49840);
#8200=VERTEX_POINT('',#49842);
#8201=VERTEX_POINT('',#49844);
#8202=VERTEX_POINT('',#49846);
#8203=VERTEX_POINT('',#49848);
#8204=VERTEX_POINT('',#49850);
#8205=VERTEX_POINT('',#49855);
#8206=VERTEX_POINT('',#49876);
#8207=VERTEX_POINT('',#49877);
#8208=VERTEX_POINT('',#49881);
#8209=VERTEX_POINT('',#49882);
#8210=VERTEX_POINT('',#49884);
#8211=VERTEX_POINT('',#49886);
#8212=VERTEX_POINT('',#49893);
#8213=VERTEX_POINT('',#49894);
#8214=VERTEX_POINT('',#49896);
#8215=VERTEX_POINT('',#49898);
#8216=VERTEX_POINT('',#49900);
#8217=VERTEX_POINT('',#49902);
#8218=VERTEX_POINT('',#49904);
#8219=VERTEX_POINT('',#49907);
#8220=VERTEX_POINT('',#49909);
#8221=VERTEX_POINT('',#49911);
#8222=VERTEX_POINT('',#49915);
#8223=VERTEX_POINT('',#49917);
#8224=VERTEX_POINT('',#49920);
#8225=VERTEX_POINT('',#49921);
#8226=VERTEX_POINT('',#49924);
#8227=VERTEX_POINT('',#49926);
#8228=VERTEX_POINT('',#49930);
#8229=VERTEX_POINT('',#49931);
#8230=VERTEX_POINT('',#49933);
#8231=VERTEX_POINT('',#49950);
#8232=VERTEX_POINT('',#49967);
#8233=VERTEX_POINT('',#49969);
#8234=VERTEX_POINT('',#49984);
#8235=VERTEX_POINT('',#49986);
#8236=VERTEX_POINT('',#49990);
#8237=VERTEX_POINT('',#49992);
#8238=VERTEX_POINT('',#50006);
#8239=VERTEX_POINT('',#50008);
#8240=VERTEX_POINT('',#50013);
#8241=VERTEX_POINT('',#50018);
#8242=VERTEX_POINT('',#50035);
#8243=VERTEX_POINT('',#50037);
#8244=VERTEX_POINT('',#50039);
#8245=VERTEX_POINT('',#50070);
#8246=VERTEX_POINT('',#50081);
#8247=VERTEX_POINT('',#50137);
#8248=VERTEX_POINT('',#50205);
#8249=VERTEX_POINT('',#50356);
#8250=VERTEX_POINT('',#50357);
#8251=VERTEX_POINT('',#50471);
#8252=VERTEX_POINT('',#50509);
#8253=VERTEX_POINT('',#50660);
#8254=VERTEX_POINT('',#50661);
#8255=VERTEX_POINT('',#50666);
#8256=VERTEX_POINT('',#50668);
#8257=VERTEX_POINT('',#50796);
#8258=VERTEX_POINT('',#50931);
#8259=VERTEX_POINT('',#50932);
#8260=VERTEX_POINT('',#50934);
#8261=VERTEX_POINT('',#50960);
#8262=VERTEX_POINT('',#51037);
#8263=VERTEX_POINT('',#51063);
#8264=VERTEX_POINT('',#51125);
#8265=VERTEX_POINT('',#51126);
#8266=VERTEX_POINT('',#51350);
#8267=VERTEX_POINT('',#51378);
#8268=VERTEX_POINT('',#51379);
#8269=VERTEX_POINT('',#51381);
#8270=VERTEX_POINT('',#51383);
#8271=VERTEX_POINT('',#51387);
#8272=VERTEX_POINT('',#51391);
#8273=VERTEX_POINT('',#51395);
#8274=VERTEX_POINT('',#51396);
#8275=VERTEX_POINT('',#51404);
#8276=VERTEX_POINT('',#51451);
#8277=VERTEX_POINT('',#51465);
#8278=VERTEX_POINT('',#51515);
#8279=VERTEX_POINT('',#51523);
#8280=VERTEX_POINT('',#51528);
#8281=VERTEX_POINT('',#51530);
#8282=VERTEX_POINT('',#51532);
#8283=VERTEX_POINT('',#51534);
#8284=VERTEX_POINT('',#51536);
#8285=VERTEX_POINT('',#51542);
#8286=VERTEX_POINT('',#51544);
#8287=VERTEX_POINT('',#51546);
#8288=VERTEX_POINT('',#51549);
#8289=VERTEX_POINT('',#51550);
#8290=VERTEX_POINT('',#51552);
#8291=VERTEX_POINT('',#51554);
#8292=VERTEX_POINT('',#51558);
#8293=VERTEX_POINT('',#51559);
#8294=VERTEX_POINT('',#51564);
#8295=VERTEX_POINT('',#51566);
#8296=VERTEX_POINT('',#51722);
#8297=VERTEX_POINT('',#51724);
#8298=VERTEX_POINT('',#51795);
#8299=VERTEX_POINT('',#51957);
#8300=VERTEX_POINT('',#52155);
#8301=VERTEX_POINT('',#52163);
#8302=VERTEX_POINT('',#52457);
#8303=VERTEX_POINT('',#52466);
#8304=VERTEX_POINT('',#52474);
#8305=VERTEX_POINT('',#52602);
#8306=VERTEX_POINT('',#52677);
#8307=VERTEX_POINT('',#52857);
#8308=VERTEX_POINT('',#52880);
#8309=VERTEX_POINT('',#53071);
#8310=VERTEX_POINT('',#53176);
#8311=VERTEX_POINT('',#53184);
#8312=VERTEX_POINT('',#53279);
#8313=VERTEX_POINT('',#53299);
#8314=VERTEX_POINT('',#53387);
#8315=VERTEX_POINT('',#53392);
#8316=VERTEX_POINT('',#53504);
#8317=VERTEX_POINT('',#53533);
#8318=VERTEX_POINT('',#53685);
#8319=VERTEX_POINT('',#53792);
#8320=VERTEX_POINT('',#53881);
#8321=VERTEX_POINT('',#53992);
#10668=EDGE_CURVE('',#8073,#8074,#1520,.T.);
#10669=EDGE_CURVE('',#8075,#8073,#1362,.T.);
#10670=EDGE_CURVE('',#8075,#8076,#1521,.T.);
#10671=EDGE_CURVE('',#8077,#8076,#1363,.T.);
#10672=EDGE_CURVE('',#8078,#8077,#1364,.T.);
#10673=EDGE_CURVE('',#8079,#8078,#1365,.T.);
#10674=EDGE_CURVE('',#8080,#8079,#1366,.T.);
#10675=EDGE_CURVE('',#8081,#8080,#1367,.T.);
#10676=EDGE_CURVE('',#8082,#8081,#1368,.T.);
#10677=EDGE_CURVE('',#8074,#8082,#1369,.T.);
#10678=EDGE_CURVE('',#8083,#8084,#1522,.T.);
#10679=EDGE_CURVE('',#8085,#8083,#1370,.T.);
#10680=EDGE_CURVE('',#8085,#8086,#1523,.T.);
#10681=EDGE_CURVE('',#8087,#8086,#1371,.T.);
#10682=EDGE_CURVE('',#8088,#8087,#1372,.T.);
#10683=EDGE_CURVE('',#8089,#8088,#1373,.T.);
#10684=EDGE_CURVE('',#8090,#8089,#1374,.T.);
#10685=EDGE_CURVE('',#8091,#8090,#1375,.T.);
#10686=EDGE_CURVE('',#8092,#8091,#1376,.T.);
#10687=EDGE_CURVE('',#8084,#8092,#1377,.T.);
#10688=EDGE_CURVE('',#8093,#8094,#1524,.T.);
#10689=EDGE_CURVE('',#8095,#8093,#1378,.T.);
#10690=EDGE_CURVE('',#8095,#8096,#1525,.T.);
#10691=EDGE_CURVE('',#8097,#8096,#1379,.T.);
#10692=EDGE_CURVE('',#8098,#8097,#1380,.T.);
#10693=EDGE_CURVE('',#8099,#8098,#1381,.T.);
#10694=EDGE_CURVE('',#8100,#8099,#1382,.T.);
#10695=EDGE_CURVE('',#8101,#8100,#1383,.T.);
#10696=EDGE_CURVE('',#8102,#8101,#1384,.T.);
#10697=EDGE_CURVE('',#8094,#8102,#1385,.T.);
#10698=EDGE_CURVE('',#8103,#8104,#1526,.T.);
#10699=EDGE_CURVE('',#8105,#8103,#1386,.T.);
#10700=EDGE_CURVE('',#8105,#8106,#1527,.T.);
#10701=EDGE_CURVE('',#8107,#8106,#1387,.T.);
#10702=EDGE_CURVE('',#8108,#8107,#1388,.T.);
#10703=EDGE_CURVE('',#8109,#8108,#1389,.T.);
#10704=EDGE_CURVE('',#8110,#8109,#1390,.T.);
#10705=EDGE_CURVE('',#8111,#8110,#1391,.T.);
#10706=EDGE_CURVE('',#8112,#8111,#1392,.T.);
#10707=EDGE_CURVE('',#8104,#8112,#1393,.T.);
#10708=EDGE_CURVE('',#8113,#8114,#1528,.T.);
#10709=EDGE_CURVE('',#8115,#8113,#1394,.T.);
#10710=EDGE_CURVE('',#8115,#8116,#1529,.T.);
#10711=EDGE_CURVE('',#8117,#8116,#1395,.T.);
#10712=EDGE_CURVE('',#8118,#8117,#1396,.T.);
#10713=EDGE_CURVE('',#8119,#8118,#1397,.T.);
#10714=EDGE_CURVE('',#8120,#8119,#1398,.T.);
#10715=EDGE_CURVE('',#8121,#8120,#1399,.T.);
#10716=EDGE_CURVE('',#8122,#8121,#1400,.T.);
#10717=EDGE_CURVE('',#8114,#8122,#1401,.T.);
#10718=EDGE_CURVE('',#8123,#8124,#1402,.T.);
#10719=EDGE_CURVE('',#8123,#8125,#2340,.T.);
#10720=EDGE_CURVE('',#8125,#8126,#6360,.F.);
#10721=EDGE_CURVE('',#8126,#8127,#2341,.F.);
#10722=EDGE_CURVE('',#8127,#8128,#6361,.T.);
#10723=EDGE_CURVE('',#8128,#8124,#6362,.T.);
#10724=EDGE_CURVE('',#8129,#8129,#6363,.F.);
#10725=EDGE_CURVE('',#8129,#8130,#2342,.T.);
#10726=EDGE_CURVE('',#8130,#8130,#6364,.T.);
#10727=EDGE_CURVE('',#8131,#8132,#6365,.T.);
#10728=EDGE_CURVE('',#8132,#8133,#2343,.F.);
#10729=EDGE_CURVE('',#8133,#8134,#6366,.F.);
#10730=EDGE_CURVE('',#8134,#8131,#2344,.T.);
#10731=EDGE_CURVE('',#8135,#8136,#2345,.F.);
#10732=EDGE_CURVE('',#8136,#8137,#6367,.T.);
#10733=EDGE_CURVE('',#8137,#8138,#2346,.T.);
#10734=EDGE_CURVE('',#8138,#8135,#6368,.F.);
#10735=EDGE_CURVE('',#8139,#8140,#6369,.F.);
#10736=EDGE_CURVE('',#8140,#8141,#6370,.T.);
#10737=EDGE_CURVE('',#8142,#8141,#6371,.T.);
#10738=EDGE_CURVE('',#8142,#8143,#6372,.F.);
#10739=EDGE_CURVE('',#8144,#8143,#6373,.F.);
#10740=EDGE_CURVE('',#8144,#8145,#6374,.F.);
#10741=EDGE_CURVE('',#8145,#8146,#6375,.F.);
#10742=EDGE_CURVE('',#8146,#8147,#6376,.F.);
#10743=EDGE_CURVE('',#8148,#8147,#6377,.F.);
#10744=EDGE_CURVE('',#8148,#8139,#6378,.F.);
#10745=EDGE_CURVE('',#8149,#8149,#6379,.T.);
#10746=EDGE_CURVE('',#8150,#8150,#6380,.T.);
#10747=EDGE_CURVE('',#8151,#8151,#6381,.T.);
#10748=EDGE_CURVE('',#8152,#8152,#6382,.T.);
#10749=EDGE_CURVE('',#8141,#8153,#1403,.T.);
#10750=EDGE_CURVE('',#8153,#8154,#2347,.T.);
#10751=EDGE_CURVE('',#8154,#8155,#6383,.F.);
#10752=EDGE_CURVE('',#8155,#8156,#2348,.F.);
#10753=EDGE_CURVE('',#8156,#8142,#1404,.T.);
#10754=EDGE_CURVE('',#8157,#8158,#6384,.F.);
#10755=EDGE_CURVE('',#8158,#8159,#2349,.F.);
#10756=EDGE_CURVE('',#8159,#8160,#6385,.T.);
#10757=EDGE_CURVE('',#8160,#8157,#2350,.T.);
#10758=EDGE_CURVE('',#8161,#8162,#1405,.F.);
#10759=EDGE_CURVE('',#8163,#8161,#6386,.F.);
#10760=EDGE_CURVE('',#8164,#8163,#6387,.F.);
#10761=EDGE_CURVE('',#8165,#8164,#1406,.F.);
#10762=EDGE_CURVE('',#8166,#8165,#6388,.T.);
#10763=EDGE_CURVE('',#8166,#8167,#2351,.T.);
#10764=EDGE_CURVE('',#8167,#8168,#6389,.F.);
#10765=EDGE_CURVE('',#8168,#8167,#6390,.F.);
#10766=EDGE_CURVE('',#8162,#8166,#6391,.T.);
#10767=EDGE_CURVE('',#8113,#8115,#1407,.T.);
#10768=EDGE_CURVE('',#8103,#8105,#1408,.T.);
#10769=EDGE_CURVE('',#8093,#8095,#1409,.T.);
#10770=EDGE_CURVE('',#8083,#8085,#1410,.T.);
#10771=EDGE_CURVE('',#8073,#8075,#1411,.T.);
#10772=EDGE_CURVE('',#8169,#8170,#2352,.T.);
#10773=EDGE_CURVE('',#8170,#8171,#6392,.T.);
#10774=EDGE_CURVE('',#8172,#8171,#2353,.T.);
#10775=EDGE_CURVE('',#8172,#8169,#6393,.F.);
#10776=EDGE_CURVE('',#8173,#8174,#2354,.T.);
#10777=EDGE_CURVE('',#8174,#8170,#2355,.F.);
#10778=EDGE_CURVE('',#8169,#8173,#2356,.T.);
#10779=EDGE_CURVE('',#8175,#8176,#2357,.T.);
#10780=EDGE_CURVE('',#8176,#8177,#6394,.T.);
#10781=EDGE_CURVE('',#8178,#8177,#2358,.T.);
#10782=EDGE_CURVE('',#8178,#8175,#6395,.F.);
#10783=EDGE_CURVE('',#8177,#8179,#2359,.T.);
#10784=EDGE_CURVE('',#8180,#8179,#2360,.T.);
#10785=EDGE_CURVE('',#8180,#8178,#2361,.F.);
#10786=EDGE_CURVE('',#8179,#8174,#6396,.T.);
#10787=EDGE_CURVE('',#8173,#8180,#6397,.F.);
#10788=EDGE_CURVE('',#8181,#8182,#2362,.F.);
#10789=EDGE_CURVE('',#8182,#8183,#6398,.F.);
#10790=EDGE_CURVE('',#8183,#8184,#2363,.F.);
#10791=EDGE_CURVE('',#8184,#8185,#2364,.T.);
#10792=EDGE_CURVE('',#8185,#8186,#6399,.T.);
#10793=EDGE_CURVE('',#8186,#8187,#2365,.T.);
#10794=EDGE_CURVE('',#8187,#8188,#6400,.T.);
#10795=EDGE_CURVE('',#8188,#8189,#2366,.F.);
#10796=EDGE_CURVE('',#8189,#8190,#6401,.T.);
#10797=EDGE_CURVE('',#8190,#8181,#2367,.T.);
#10798=EDGE_CURVE('',#8191,#8191,#6402,.T.);
#10799=EDGE_CURVE('',#8192,#8192,#6403,.T.);
#10800=EDGE_CURVE('',#8193,#8193,#6404,.F.);
#10801=EDGE_CURVE('',#8194,#8195,#1412,.T.);
#10802=EDGE_CURVE('',#8195,#8196,#1413,.T.);
#10803=EDGE_CURVE('',#8196,#8197,#2368,.F.);
#10804=EDGE_CURVE('',#8197,#8198,#6405,.F.);
#10805=EDGE_CURVE('',#8198,#8199,#2369,.T.);
#10806=EDGE_CURVE('',#8199,#8200,#6406,.F.);
#10807=EDGE_CURVE('',#8200,#8201,#2370,.F.);
#10808=EDGE_CURVE('',#8201,#8202,#6407,.F.);
#10809=EDGE_CURVE('',#8202,#8203,#2371,.F.);
#10810=EDGE_CURVE('',#8203,#8204,#1414,.T.);
#10811=EDGE_CURVE('',#8204,#8205,#1415,.T.);
#10812=EDGE_CURVE('',#8205,#8194,#1416,.T.);
#10813=EDGE_CURVE('',#8206,#8207,#6408,.T.);
#10814=EDGE_CURVE('',#8207,#8206,#6409,.T.);
#10815=EDGE_CURVE('',#8208,#8209,#2372,.T.);
#10816=EDGE_CURVE('',#8209,#8210,#6410,.F.);
#10817=EDGE_CURVE('',#8211,#8210,#2373,.T.);
#10818=EDGE_CURVE('',#8211,#8208,#6411,.T.);
#10819=EDGE_CURVE('',#8210,#8209,#6412,.F.);
#10820=EDGE_CURVE('',#8208,#8211,#6413,.T.);
#10821=EDGE_CURVE('',#8212,#8213,#6414,.T.);
#10822=EDGE_CURVE('',#8213,#8214,#6415,.T.);
#10823=EDGE_CURVE('',#8214,#8215,#6416,.T.);
#10824=EDGE_CURVE('',#8216,#8215,#6417,.F.);
#10825=EDGE_CURVE('',#8216,#8217,#6418,.T.);
#10826=EDGE_CURVE('',#8217,#8218,#6419,.F.);
#10827=EDGE_CURVE('',#8135,#8218,#6420,.T.);
#10828=EDGE_CURVE('',#8219,#8138,#6421,.T.);
#10829=EDGE_CURVE('',#8219,#8220,#6422,.F.);
#10830=EDGE_CURVE('',#8220,#8221,#6423,.T.);
#10831=EDGE_CURVE('',#8212,#8221,#6424,.F.);
#10832=EDGE_CURVE('',#8222,#8222,#6425,.F.);
#10833=EDGE_CURVE('',#8223,#8223,#6426,.T.);
#10834=EDGE_CURVE('',#8224,#8225,#6427,.T.);
#10835=EDGE_CURVE('',#8225,#8224,#6428,.T.);
#10836=EDGE_CURVE('',#8224,#8226,#2374,.T.);
#10837=EDGE_CURVE('',#8226,#8227,#6429,.F.);
#10838=EDGE_CURVE('',#8227,#8226,#6430,.F.);
#10839=EDGE_CURVE('',#8228,#8229,#2375,.F.);
#10840=EDGE_CURVE('',#8229,#8230,#1417,.T.);
#10841=EDGE_CURVE('',#8230,#8231,#1418,.T.);
#10842=EDGE_CURVE('',#8231,#8232,#2376,.T.);
#10843=EDGE_CURVE('',#8232,#8233,#1419,.T.);
#10844=EDGE_CURVE('',#8233,#8176,#2377,.T.);
#10845=EDGE_CURVE('',#8175,#8234,#2378,.F.);
#10846=EDGE_CURVE('',#8234,#8235,#2379,.F.);
#10847=EDGE_CURVE('',#8228,#8235,#124,.F.);
#10848=EDGE_CURVE('',#8171,#8236,#2380,.T.);
#10849=EDGE_CURVE('',#8236,#8237,#1420,.T.);
#10850=EDGE_CURVE('',#8237,#8238,#2381,.T.);
#10851=EDGE_CURVE('',#8238,#8239,#1421,.T.);
#10852=EDGE_CURVE('',#8239,#8240,#1422,.T.);
#10853=EDGE_CURVE('',#8240,#8241,#1423,.T.);
#10854=EDGE_CURVE('',#8241,#8242,#2382,.F.);
#10855=EDGE_CURVE('',#8243,#8242,#125,.F.);
#10856=EDGE_CURVE('',#8243,#8244,#2383,.T.);
#10857=EDGE_CURVE('',#8244,#8172,#2384,.F.);
#10858=EDGE_CURVE('',#8164,#8245,#1424,.F.);
#10859=EDGE_CURVE('',#8245,#8246,#1425,.T.);
#10860=EDGE_CURVE('',#8246,#8247,#1426,.T.);
#10861=EDGE_CURVE('',#8247,#8248,#1427,.T.);
#10862=EDGE_CURVE('',#8248,#8165,#1428,.F.);
#10863=EDGE_CURVE('',#8249,#8250,#1429,.T.);
#10864=EDGE_CURVE('',#8250,#8161,#1430,.F.);
#10865=EDGE_CURVE('',#8162,#8251,#1431,.F.);
#10866=EDGE_CURVE('',#8251,#8252,#1432,.T.);
#10867=EDGE_CURVE('',#8252,#8249,#1433,.T.);
#10868=EDGE_CURVE('',#8253,#8254,#1434,.F.);
#10869=EDGE_CURVE('',#8254,#8255,#2385,.F.);
#10870=EDGE_CURVE('',#8255,#8256,#1435,.T.);
#10871=EDGE_CURVE('',#8256,#8257,#1436,.T.);
#10872=EDGE_CURVE('',#8257,#8164,#1437,.F.);
#10873=EDGE_CURVE('',#8163,#8253,#1438,.T.);
#10874=EDGE_CURVE('',#8258,#8259,#2386,.F.);
#10875=EDGE_CURVE('',#8259,#8260,#1439,.F.);
#10876=EDGE_CURVE('',#8260,#8261,#1440,.T.);
#10877=EDGE_CURVE('',#8261,#8162,#1441,.F.);
#10878=EDGE_CURVE('',#8165,#8262,#1442,.F.);
#10879=EDGE_CURVE('',#8262,#8263,#1443,.T.);
#10880=EDGE_CURVE('',#8263,#8258,#1444,.T.);
#10881=EDGE_CURVE('',#8264,#8265,#1445,.T.);
#10882=EDGE_CURVE('',#8265,#8253,#1446,.F.);
#10883=EDGE_CURVE('',#8161,#8264,#1447,.F.);
#10884=EDGE_CURVE('',#8266,#8266,#6431,.T.);
#10885=EDGE_CURVE('',#8076,#8074,#1448,.T.);
#10886=EDGE_CURVE('',#8086,#8084,#1449,.T.);
#10887=EDGE_CURVE('',#8096,#8094,#1450,.T.);
#10888=EDGE_CURVE('',#8106,#8104,#1451,.T.);
#10889=EDGE_CURVE('',#8116,#8114,#1452,.T.);
#10890=EDGE_CURVE('',#8267,#8268,#6432,.F.);
#10891=EDGE_CURVE('',#8268,#8269,#2387,.T.);
#10892=EDGE_CURVE('',#8269,#8270,#6433,.T.);
#10893=EDGE_CURVE('',#8270,#8267,#2388,.F.);
#10894=EDGE_CURVE('',#8218,#8271,#2389,.F.);
#10895=EDGE_CURVE('',#8271,#8136,#6434,.T.);
#10896=EDGE_CURVE('',#8137,#8272,#6435,.T.);
#10897=EDGE_CURVE('',#8272,#8219,#2390,.T.);
#10898=EDGE_CURVE('',#8273,#8274,#1453,.T.);
#10899=EDGE_CURVE('',#8274,#8275,#1454,.T.);
#10900=EDGE_CURVE('',#8275,#8276,#1455,.T.);
#10901=EDGE_CURVE('',#8276,#8277,#1456,.T.);
#10902=EDGE_CURVE('',#8277,#8278,#1457,.T.);
#10903=EDGE_CURVE('',#8278,#8279,#1458,.T.);
#10904=EDGE_CURVE('',#8279,#8280,#2391,.T.);
#10905=EDGE_CURVE('',#8280,#8281,#2392,.F.);
#10906=EDGE_CURVE('',#8281,#8282,#6436,.T.);
#10907=EDGE_CURVE('',#8282,#8283,#2393,.F.);
#10908=EDGE_CURVE('',#8283,#8284,#2394,.T.);
#10909=EDGE_CURVE('',#8284,#8273,#1459,.T.);
#10910=EDGE_CURVE('',#8285,#8285,#6437,.F.);
#10911=EDGE_CURVE('',#8286,#8286,#6438,.T.);
#10912=EDGE_CURVE('',#8287,#8287,#6439,.T.);
#10913=EDGE_CURVE('',#8288,#8289,#2395,.T.);
#10914=EDGE_CURVE('',#8289,#8290,#6440,.T.);
#10915=EDGE_CURVE('',#8291,#8290,#2396,.T.);
#10916=EDGE_CURVE('',#8291,#8288,#6441,.F.);
#10917=EDGE_CURVE('',#8292,#8293,#2397,.T.);
#10918=EDGE_CURVE('',#8293,#8289,#2398,.T.);
#10919=EDGE_CURVE('',#8288,#8292,#2399,.T.);
#10920=EDGE_CURVE('',#8290,#8294,#2400,.T.);
#10921=EDGE_CURVE('',#8294,#8295,#2401,.F.);
#10922=EDGE_CURVE('',#8295,#8291,#2402,.T.);
#10923=EDGE_CURVE('',#8296,#8247,#6442,.F.);
#10924=EDGE_CURVE('',#8296,#8297,#1460,.T.);
#10925=EDGE_CURVE('',#8297,#8298,#1461,.T.);
#10926=EDGE_CURVE('',#8298,#8248,#1462,.T.);
#10927=EDGE_CURVE('',#8299,#8246,#6443,.F.);
#10928=EDGE_CURVE('',#8299,#8296,#1463,.F.);
#10929=EDGE_CURVE('',#8245,#8300,#1464,.T.);
#10930=EDGE_CURVE('',#8300,#8301,#1465,.T.);
#10931=EDGE_CURVE('',#8301,#8299,#1466,.T.);
#10932=EDGE_CURVE('',#8251,#8302,#1467,.T.);
#10933=EDGE_CURVE('',#8302,#8303,#1468,.F.);
#10934=EDGE_CURVE('',#8303,#8304,#1469,.F.);
#10935=EDGE_CURVE('',#8304,#8305,#1470,.F.);
#10936=EDGE_CURVE('',#8252,#8305,#6444,.F.);
#10937=EDGE_CURVE('',#8305,#8306,#1471,.F.);
#10938=EDGE_CURVE('',#8249,#8306,#6445,.T.);
#10939=EDGE_CURVE('',#8306,#8307,#1472,.F.);
#10940=EDGE_CURVE('',#8307,#8308,#1473,.F.);
#10941=EDGE_CURVE('',#8308,#8309,#1474,.F.);
#10942=EDGE_CURVE('',#8309,#8250,#1475,.T.);
#10943=EDGE_CURVE('',#8309,#8310,#1476,.T.);
#10944=EDGE_CURVE('',#8310,#8311,#1477,.T.);
#10945=EDGE_CURVE('',#8311,#8265,#1478,.T.);
#10946=EDGE_CURVE('',#8250,#8264,#1479,.T.);
#10947=EDGE_CURVE('',#8255,#8312,#1480,.T.);
#10948=EDGE_CURVE('',#8312,#8313,#1481,.T.);
#10949=EDGE_CURVE('',#8313,#8300,#1482,.T.);
#10950=EDGE_CURVE('',#8257,#8245,#1483,.T.);
#10951=EDGE_CURVE('',#8298,#8314,#1484,.T.);
#10952=EDGE_CURVE('',#8314,#8315,#1485,.T.);
#10953=EDGE_CURVE('',#8315,#8258,#1486,.T.);
#10954=EDGE_CURVE('',#8248,#8262,#1487,.T.);
#10955=EDGE_CURVE('',#8251,#8261,#1488,.F.);
#10956=EDGE_CURVE('',#8260,#8316,#1489,.T.);
#10957=EDGE_CURVE('',#8316,#8317,#1490,.T.);
#10958=EDGE_CURVE('',#8317,#8302,#1491,.T.);
#10959=EDGE_CURVE('',#8214,#8158,#6446,.T.);
#10960=EDGE_CURVE('',#8215,#8157,#6447,.T.);
#10961=EDGE_CURVE('',#8268,#8157,#6448,.F.);
#10962=EDGE_CURVE('',#8216,#8268,#6449,.F.);
#10963=EDGE_CURVE('',#8160,#8269,#6450,.F.);
#10964=EDGE_CURVE('',#8217,#8267,#1492,.T.);
#10965=EDGE_CURVE('',#8269,#8139,#6451,.F.);
#10966=EDGE_CURVE('',#8270,#8148,#6452,.T.);
#10967=EDGE_CURVE('',#8271,#8270,#6453,.T.);
#10968=EDGE_CURVE('',#8271,#8147,#6454,.F.);
#10969=EDGE_CURVE('',#8136,#8146,#1493,.T.);
#10970=EDGE_CURVE('',#8137,#8145,#1494,.T.);
#10971=EDGE_CURVE('',#8272,#8144,#6455,.T.);
#10972=EDGE_CURVE('',#8131,#8143,#6456,.F.);
#10973=EDGE_CURVE('',#8272,#8131,#6457,.F.);
#10974=EDGE_CURVE('',#8132,#8156,#126,.F.);
#10975=EDGE_CURVE('',#8220,#8134,#1495,.T.);
#10976=EDGE_CURVE('',#8133,#8155,#6458,.T.);
#10977=EDGE_CURVE('',#8221,#8133,#6459,.T.);
#10978=EDGE_CURVE('',#8212,#8155,#6460,.F.);
#10979=EDGE_CURVE('',#8154,#8213,#6461,.F.);
#10980=EDGE_CURVE('',#8317,#8279,#1496,.F.);
#10981=EDGE_CURVE('',#8302,#8278,#6462,.T.);
#10982=EDGE_CURVE('',#8175,#8185,#6463,.T.);
#10983=EDGE_CURVE('',#8186,#8178,#6464,.T.);
#10984=EDGE_CURVE('',#8279,#8318,#1497,.T.);
#10985=EDGE_CURVE('',#8318,#8229,#1498,.T.);
#10986=EDGE_CURVE('',#8280,#8228,#6465,.T.);
#10987=EDGE_CURVE('',#8305,#8276,#6466,.F.);
#10988=EDGE_CURVE('',#8187,#8180,#6467,.T.);
#10989=EDGE_CURVE('',#8234,#8184,#6468,.T.);
#10990=EDGE_CURVE('',#8235,#8292,#6469,.T.);
#10991=EDGE_CURVE('',#8293,#8234,#6470,.T.);
#10992=EDGE_CURVE('',#8280,#8292,#127,.T.);
#10993=EDGE_CURVE('',#8306,#8275,#6471,.F.);
#10994=EDGE_CURVE('',#8188,#8173,#6472,.T.);
#10995=EDGE_CURVE('',#8293,#8184,#6473,.F.);
#10996=EDGE_CURVE('',#8281,#8288,#6474,.T.);
#10997=EDGE_CURVE('',#8309,#8273,#6475,.F.);
#10998=EDGE_CURVE('',#8189,#8169,#6476,.T.);
#10999=EDGE_CURVE('',#8289,#8183,#6477,.T.);
#11000=EDGE_CURVE('',#8282,#8291,#6478,.T.);
#11001=EDGE_CURVE('',#8284,#8310,#1499,.F.);
#11002=EDGE_CURVE('',#8190,#8172,#6479,.T.);
#11003=EDGE_CURVE('',#8290,#8182,#6480,.T.);
#11004=EDGE_CURVE('',#8283,#8295,#128,.F.);
#11005=EDGE_CURVE('',#8241,#8319,#1500,.T.);
#11006=EDGE_CURVE('',#8319,#8284,#1501,.T.);
#11007=EDGE_CURVE('',#8242,#8283,#6481,.T.);
#11008=EDGE_CURVE('',#8181,#8244,#6482,.T.);
#11009=EDGE_CURVE('',#8294,#8181,#6483,.T.);
#11010=EDGE_CURVE('',#8243,#8295,#6484,.F.);
#11011=EDGE_CURVE('',#8294,#8244,#6485,.F.);
#11012=EDGE_CURVE('',#8124,#8127,#6486,.T.);
#11013=EDGE_CURVE('',#8128,#8222,#6487,.T.);
#11014=EDGE_CURVE('',#8223,#8227,#6488,.T.);
#11015=EDGE_CURVE('',#8203,#8314,#1502,.F.);
#11016=EDGE_CURVE('',#8204,#8298,#6489,.T.);
#11017=EDGE_CURVE('',#8233,#8320,#1503,.T.);
#11018=EDGE_CURVE('',#8320,#8203,#1504,.T.);
#11019=EDGE_CURVE('',#8176,#8202,#6490,.T.);
#11020=EDGE_CURVE('',#8205,#8296,#6491,.T.);
#11021=EDGE_CURVE('',#8177,#8201,#6492,.T.);
#11022=EDGE_CURVE('',#8194,#8299,#6493,.F.);
#11023=EDGE_CURVE('',#8179,#8200,#6494,.T.);
#11024=EDGE_CURVE('',#8195,#8300,#6495,.T.);
#11025=EDGE_CURVE('',#8174,#8199,#6496,.T.);
#11026=EDGE_CURVE('',#8313,#8196,#1505,.F.);
#11027=EDGE_CURVE('',#8170,#8198,#6497,.T.);
#11028=EDGE_CURVE('',#8196,#8321,#1506,.T.);
#11029=EDGE_CURVE('',#8321,#8236,#1507,.T.);
#11030=EDGE_CURVE('',#8197,#8171,#6498,.T.);
#11031=EDGE_CURVE('',#8210,#8206,#1508,.T.);
#11032=EDGE_CURVE('',#8207,#8209,#1509,.F.);
#11033=EDGE_CURVE('',#8225,#8193,#6499,.T.);
#11034=EDGE_CURVE('',#8130,#8285,#6500,.T.);
#11035=EDGE_CURVE('',#8139,#8160,#6501,.T.);
#11036=EDGE_CURVE('',#8214,#8125,#6502,.T.);
#11037=EDGE_CURVE('',#8126,#8213,#6503,.T.);
#11038=EDGE_CURVE('',#8158,#8125,#6504,.T.);
#11039=EDGE_CURVE('',#8126,#8154,#6505,.T.);
#11040=EDGE_CURVE('',#8159,#8123,#6506,.T.);
#11041=EDGE_CURVE('',#8140,#8159,#1510,.T.);
#11042=EDGE_CURVE('',#8127,#8153,#1511,.F.);
#11043=EDGE_CURVE('',#8140,#8124,#6507,.F.);
#11044=EDGE_CURVE('',#8314,#8320,#129,.F.);
#11045=EDGE_CURVE('',#8315,#8233,#6508,.T.);
#11046=EDGE_CURVE('',#8258,#8232,#6509,.T.);
#11047=EDGE_CURVE('',#8259,#8231,#6510,.F.);
#11048=EDGE_CURVE('',#8260,#8230,#6511,.F.);
#11049=EDGE_CURVE('',#8316,#8229,#6512,.T.);
#11050=EDGE_CURVE('',#8317,#8318,#6513,.T.);
#11051=EDGE_CURVE('',#8310,#8319,#6514,.F.);
#11052=EDGE_CURVE('',#8311,#8241,#6515,.T.);
#11053=EDGE_CURVE('',#8265,#8240,#6516,.T.);
#11054=EDGE_CURVE('',#8253,#8239,#6517,.F.);
#11055=EDGE_CURVE('',#8254,#8238,#6518,.F.);
#11056=EDGE_CURVE('',#8255,#8237,#6519,.F.);
#11057=EDGE_CURVE('',#8312,#8236,#6520,.T.);
#11058=EDGE_CURVE('',#8313,#8321,#130,.T.);
#11059=EDGE_CURVE('',#8287,#8152,#2403,.T.);
#11060=EDGE_CURVE('',#8286,#8151,#2404,.T.);
#11061=EDGE_CURVE('',#8192,#8150,#2405,.T.);
#11062=EDGE_CURVE('',#8191,#8149,#2406,.T.);
#11063=EDGE_CURVE('',#8266,#8168,#6521,.T.);
#15753=ORIENTED_EDGE('',*,*,#10668,.F.);
#15754=ORIENTED_EDGE('',*,*,#10669,.F.);
#15755=ORIENTED_EDGE('',*,*,#10670,.T.);
#15756=ORIENTED_EDGE('',*,*,#10671,.F.);
#15757=ORIENTED_EDGE('',*,*,#10672,.F.);
#15758=ORIENTED_EDGE('',*,*,#10673,.F.);
#15759=ORIENTED_EDGE('',*,*,#10674,.F.);
#15760=ORIENTED_EDGE('',*,*,#10675,.F.);
#15761=ORIENTED_EDGE('',*,*,#10676,.F.);
#15762=ORIENTED_EDGE('',*,*,#10677,.F.);
#15763=ORIENTED_EDGE('',*,*,#10678,.F.);
#15764=ORIENTED_EDGE('',*,*,#10679,.F.);
#15765=ORIENTED_EDGE('',*,*,#10680,.T.);
#15766=ORIENTED_EDGE('',*,*,#10681,.F.);
#15767=ORIENTED_EDGE('',*,*,#10682,.F.);
#15768=ORIENTED_EDGE('',*,*,#10683,.F.);
#15769=ORIENTED_EDGE('',*,*,#10684,.F.);
#15770=ORIENTED_EDGE('',*,*,#10685,.F.);
#15771=ORIENTED_EDGE('',*,*,#10686,.F.);
#15772=ORIENTED_EDGE('',*,*,#10687,.F.);
#15773=ORIENTED_EDGE('',*,*,#10688,.F.);
#15774=ORIENTED_EDGE('',*,*,#10689,.F.);
#15775=ORIENTED_EDGE('',*,*,#10690,.T.);
#15776=ORIENTED_EDGE('',*,*,#10691,.F.);
#15777=ORIENTED_EDGE('',*,*,#10692,.F.);
#15778=ORIENTED_EDGE('',*,*,#10693,.F.);
#15779=ORIENTED_EDGE('',*,*,#10694,.F.);
#15780=ORIENTED_EDGE('',*,*,#10695,.F.);
#15781=ORIENTED_EDGE('',*,*,#10696,.F.);
#15782=ORIENTED_EDGE('',*,*,#10697,.F.);
#15783=ORIENTED_EDGE('',*,*,#10698,.F.);
#15784=ORIENTED_EDGE('',*,*,#10699,.F.);
#15785=ORIENTED_EDGE('',*,*,#10700,.T.);
#15786=ORIENTED_EDGE('',*,*,#10701,.F.);
#15787=ORIENTED_EDGE('',*,*,#10702,.F.);
#15788=ORIENTED_EDGE('',*,*,#10703,.F.);
#15789=ORIENTED_EDGE('',*,*,#10704,.F.);
#15790=ORIENTED_EDGE('',*,*,#10705,.F.);
#15791=ORIENTED_EDGE('',*,*,#10706,.F.);
#15792=ORIENTED_EDGE('',*,*,#10707,.F.);
#15793=ORIENTED_EDGE('',*,*,#10708,.F.);
#15794=ORIENTED_EDGE('',*,*,#10709,.F.);
#15795=ORIENTED_EDGE('',*,*,#10710,.T.);
#15796=ORIENTED_EDGE('',*,*,#10711,.F.);
#15797=ORIENTED_EDGE('',*,*,#10712,.F.);
#15798=ORIENTED_EDGE('',*,*,#10713,.F.);
#15799=ORIENTED_EDGE('',*,*,#10714,.F.);
#15800=ORIENTED_EDGE('',*,*,#10715,.F.);
#15801=ORIENTED_EDGE('',*,*,#10716,.F.);
#15802=ORIENTED_EDGE('',*,*,#10717,.F.);
#15803=ORIENTED_EDGE('',*,*,#10718,.F.);
#15804=ORIENTED_EDGE('',*,*,#10719,.T.);
#15805=ORIENTED_EDGE('',*,*,#10720,.T.);
#15806=ORIENTED_EDGE('',*,*,#10721,.T.);
#15807=ORIENTED_EDGE('',*,*,#10722,.T.);
#15808=ORIENTED_EDGE('',*,*,#10723,.T.);
#15809=ORIENTED_EDGE('',*,*,#10724,.T.);
#15810=ORIENTED_EDGE('',*,*,#10725,.T.);
#15811=ORIENTED_EDGE('',*,*,#10726,.T.);
#15812=ORIENTED_EDGE('',*,*,#10725,.F.);
#15813=ORIENTED_EDGE('',*,*,#10727,.T.);
#15814=ORIENTED_EDGE('',*,*,#10728,.T.);
#15815=ORIENTED_EDGE('',*,*,#10729,.T.);
#15816=ORIENTED_EDGE('',*,*,#10730,.T.);
#15817=ORIENTED_EDGE('',*,*,#10731,.T.);
#15818=ORIENTED_EDGE('',*,*,#10732,.T.);
#15819=ORIENTED_EDGE('',*,*,#10733,.T.);
#15820=ORIENTED_EDGE('',*,*,#10734,.T.);
#15821=ORIENTED_EDGE('',*,*,#10735,.T.);
#15822=ORIENTED_EDGE('',*,*,#10736,.T.);
#15823=ORIENTED_EDGE('',*,*,#10737,.F.);
#15824=ORIENTED_EDGE('',*,*,#10738,.T.);
#15825=ORIENTED_EDGE('',*,*,#10739,.F.);
#15826=ORIENTED_EDGE('',*,*,#10740,.T.);
#15827=ORIENTED_EDGE('',*,*,#10741,.T.);
#15828=ORIENTED_EDGE('',*,*,#10742,.T.);
#15829=ORIENTED_EDGE('',*,*,#10743,.F.);
#15830=ORIENTED_EDGE('',*,*,#10744,.T.);
#15831=ORIENTED_EDGE('',*,*,#10745,.T.);
#15832=ORIENTED_EDGE('',*,*,#10746,.T.);
#15833=ORIENTED_EDGE('',*,*,#10747,.T.);
#15834=ORIENTED_EDGE('',*,*,#10748,.T.);
#15835=ORIENTED_EDGE('',*,*,#10724,.F.);
#15836=ORIENTED_EDGE('',*,*,#10749,.T.);
#15837=ORIENTED_EDGE('',*,*,#10750,.T.);
#15838=ORIENTED_EDGE('',*,*,#10751,.T.);
#15839=ORIENTED_EDGE('',*,*,#10752,.T.);
#15840=ORIENTED_EDGE('',*,*,#10753,.T.);
#15841=ORIENTED_EDGE('',*,*,#10737,.T.);
#15842=ORIENTED_EDGE('',*,*,#10754,.T.);
#15843=ORIENTED_EDGE('',*,*,#10755,.T.);
#15844=ORIENTED_EDGE('',*,*,#10756,.T.);
#15845=ORIENTED_EDGE('',*,*,#10757,.T.);
#15846=ORIENTED_EDGE('',*,*,#10758,.F.);
#15847=ORIENTED_EDGE('',*,*,#10759,.F.);
#15848=ORIENTED_EDGE('',*,*,#10760,.F.);
#15849=ORIENTED_EDGE('',*,*,#10761,.F.);
#15850=ORIENTED_EDGE('',*,*,#10762,.F.);
#15851=ORIENTED_EDGE('',*,*,#10763,.T.);
#15852=ORIENTED_EDGE('',*,*,#10764,.T.);
#15853=ORIENTED_EDGE('',*,*,#10765,.T.);
#15854=ORIENTED_EDGE('',*,*,#10763,.F.);
#15855=ORIENTED_EDGE('',*,*,#10766,.F.);
#15856=ORIENTED_EDGE('',*,*,#10709,.T.);
#15857=ORIENTED_EDGE('',*,*,#10767,.T.);
#15858=ORIENTED_EDGE('',*,*,#10699,.T.);
#15859=ORIENTED_EDGE('',*,*,#10768,.T.);
#15860=ORIENTED_EDGE('',*,*,#10689,.T.);
#15861=ORIENTED_EDGE('',*,*,#10769,.T.);
#15862=ORIENTED_EDGE('',*,*,#10679,.T.);
#15863=ORIENTED_EDGE('',*,*,#10770,.T.);
#15864=ORIENTED_EDGE('',*,*,#10669,.T.);
#15865=ORIENTED_EDGE('',*,*,#10771,.T.);
#15866=ORIENTED_EDGE('',*,*,#10772,.T.);
#15867=ORIENTED_EDGE('',*,*,#10773,.T.);
#15868=ORIENTED_EDGE('',*,*,#10774,.F.);
#15869=ORIENTED_EDGE('',*,*,#10775,.T.);
#15870=ORIENTED_EDGE('',*,*,#10776,.T.);
#15871=ORIENTED_EDGE('',*,*,#10777,.T.);
#15872=ORIENTED_EDGE('',*,*,#10772,.F.);
#15873=ORIENTED_EDGE('',*,*,#10778,.T.);
#15874=ORIENTED_EDGE('',*,*,#10779,.T.);
#15875=ORIENTED_EDGE('',*,*,#10780,.T.);
#15876=ORIENTED_EDGE('',*,*,#10781,.F.);
#15877=ORIENTED_EDGE('',*,*,#10782,.T.);
#15878=ORIENTED_EDGE('',*,*,#10781,.T.);
#15879=ORIENTED_EDGE('',*,*,#10783,.T.);
#15880=ORIENTED_EDGE('',*,*,#10784,.F.);
#15881=ORIENTED_EDGE('',*,*,#10785,.T.);
#15882=ORIENTED_EDGE('',*,*,#10784,.T.);
#15883=ORIENTED_EDGE('',*,*,#10786,.T.);
#15884=ORIENTED_EDGE('',*,*,#10776,.F.);
#15885=ORIENTED_EDGE('',*,*,#10787,.T.);
#15886=ORIENTED_EDGE('',*,*,#10788,.T.);
#15887=ORIENTED_EDGE('',*,*,#10789,.T.);
#15888=ORIENTED_EDGE('',*,*,#10790,.T.);
#15889=ORIENTED_EDGE('',*,*,#10791,.T.);
#15890=ORIENTED_EDGE('',*,*,#10792,.T.);
#15891=ORIENTED_EDGE('',*,*,#10793,.T.);
#15892=ORIENTED_EDGE('',*,*,#10794,.T.);
#15893=ORIENTED_EDGE('',*,*,#10795,.T.);
#15894=ORIENTED_EDGE('',*,*,#10796,.T.);
#15895=ORIENTED_EDGE('',*,*,#10797,.T.);
#15896=ORIENTED_EDGE('',*,*,#10798,.F.);
#15897=ORIENTED_EDGE('',*,*,#10799,.F.);
#15898=ORIENTED_EDGE('',*,*,#10800,.T.);
#15899=ORIENTED_EDGE('',*,*,#10801,.T.);
#15900=ORIENTED_EDGE('',*,*,#10802,.T.);
#15901=ORIENTED_EDGE('',*,*,#10803,.T.);
#15902=ORIENTED_EDGE('',*,*,#10804,.T.);
#15903=ORIENTED_EDGE('',*,*,#10805,.T.);
#15904=ORIENTED_EDGE('',*,*,#10806,.T.);
#15905=ORIENTED_EDGE('',*,*,#10807,.T.);
#15906=ORIENTED_EDGE('',*,*,#10808,.T.);
#15907=ORIENTED_EDGE('',*,*,#10809,.T.);
#15908=ORIENTED_EDGE('',*,*,#10810,.T.);
#15909=ORIENTED_EDGE('',*,*,#10811,.T.);
#15910=ORIENTED_EDGE('',*,*,#10812,.T.);
#15911=ORIENTED_EDGE('',*,*,#10813,.T.);
#15912=ORIENTED_EDGE('',*,*,#10814,.T.);
#15913=ORIENTED_EDGE('',*,*,#10815,.T.);
#15914=ORIENTED_EDGE('',*,*,#10816,.T.);
#15915=ORIENTED_EDGE('',*,*,#10817,.F.);
#15916=ORIENTED_EDGE('',*,*,#10818,.T.);
#15917=ORIENTED_EDGE('',*,*,#10817,.T.);
#15918=ORIENTED_EDGE('',*,*,#10819,.T.);
#15919=ORIENTED_EDGE('',*,*,#10815,.F.);
#15920=ORIENTED_EDGE('',*,*,#10820,.T.);
#15921=ORIENTED_EDGE('',*,*,#10818,.F.);
#15922=ORIENTED_EDGE('',*,*,#10820,.F.);
#15923=ORIENTED_EDGE('',*,*,#10821,.T.);
#15924=ORIENTED_EDGE('',*,*,#10822,.T.);
#15925=ORIENTED_EDGE('',*,*,#10823,.T.);
#15926=ORIENTED_EDGE('',*,*,#10824,.F.);
#15927=ORIENTED_EDGE('',*,*,#10825,.T.);
#15928=ORIENTED_EDGE('',*,*,#10826,.T.);
#15929=ORIENTED_EDGE('',*,*,#10827,.F.);
#15930=ORIENTED_EDGE('',*,*,#10734,.F.);
#15931=ORIENTED_EDGE('',*,*,#10828,.F.);
#15932=ORIENTED_EDGE('',*,*,#10829,.T.);
#15933=ORIENTED_EDGE('',*,*,#10830,.T.);
#15934=ORIENTED_EDGE('',*,*,#10831,.F.);
#15935=ORIENTED_EDGE('',*,*,#10832,.T.);
#15936=ORIENTED_EDGE('',*,*,#10833,.T.);
#15937=ORIENTED_EDGE('',*,*,#10834,.T.);
#15938=ORIENTED_EDGE('',*,*,#10835,.T.);
#15939=ORIENTED_EDGE('',*,*,#10836,.T.);
#15940=ORIENTED_EDGE('',*,*,#10837,.T.);
#15941=ORIENTED_EDGE('',*,*,#10838,.T.);
#15942=ORIENTED_EDGE('',*,*,#10836,.F.);
#15943=ORIENTED_EDGE('',*,*,#10839,.T.);
#15944=ORIENTED_EDGE('',*,*,#10840,.T.);
#15945=ORIENTED_EDGE('',*,*,#10841,.T.);
#15946=ORIENTED_EDGE('',*,*,#10842,.T.);
#15947=ORIENTED_EDGE('',*,*,#10843,.T.);
#15948=ORIENTED_EDGE('',*,*,#10844,.T.);
#15949=ORIENTED_EDGE('',*,*,#10779,.F.);
#15950=ORIENTED_EDGE('',*,*,#10845,.T.);
#15951=ORIENTED_EDGE('',*,*,#10846,.T.);
#15952=ORIENTED_EDGE('',*,*,#10847,.F.);
#15953=ORIENTED_EDGE('',*,*,#10848,.T.);
#15954=ORIENTED_EDGE('',*,*,#10849,.T.);
#15955=ORIENTED_EDGE('',*,*,#10850,.T.);
#15956=ORIENTED_EDGE('',*,*,#10851,.T.);
#15957=ORIENTED_EDGE('',*,*,#10852,.T.);
#15958=ORIENTED_EDGE('',*,*,#10853,.T.);
#15959=ORIENTED_EDGE('',*,*,#10854,.T.);
#15960=ORIENTED_EDGE('',*,*,#10855,.F.);
#15961=ORIENTED_EDGE('',*,*,#10856,.T.);
#15962=ORIENTED_EDGE('',*,*,#10857,.T.);
#15963=ORIENTED_EDGE('',*,*,#10774,.T.);
#15964=ORIENTED_EDGE('',*,*,#10761,.T.);
#15965=ORIENTED_EDGE('',*,*,#10858,.T.);
#15966=ORIENTED_EDGE('',*,*,#10859,.T.);
#15967=ORIENTED_EDGE('',*,*,#10860,.T.);
#15968=ORIENTED_EDGE('',*,*,#10861,.T.);
#15969=ORIENTED_EDGE('',*,*,#10862,.T.);
#15970=ORIENTED_EDGE('',*,*,#10863,.T.);
#15971=ORIENTED_EDGE('',*,*,#10864,.T.);
#15972=ORIENTED_EDGE('',*,*,#10758,.T.);
#15973=ORIENTED_EDGE('',*,*,#10865,.T.);
#15974=ORIENTED_EDGE('',*,*,#10866,.T.);
#15975=ORIENTED_EDGE('',*,*,#10867,.T.);
#15976=ORIENTED_EDGE('',*,*,#10868,.T.);
#15977=ORIENTED_EDGE('',*,*,#10869,.T.);
#15978=ORIENTED_EDGE('',*,*,#10870,.T.);
#15979=ORIENTED_EDGE('',*,*,#10871,.T.);
#15980=ORIENTED_EDGE('',*,*,#10872,.T.);
#15981=ORIENTED_EDGE('',*,*,#10760,.T.);
#15982=ORIENTED_EDGE('',*,*,#10873,.T.);
#15983=ORIENTED_EDGE('',*,*,#10874,.T.);
#15984=ORIENTED_EDGE('',*,*,#10875,.T.);
#15985=ORIENTED_EDGE('',*,*,#10876,.T.);
#15986=ORIENTED_EDGE('',*,*,#10877,.T.);
#15987=ORIENTED_EDGE('',*,*,#10766,.T.);
#15988=ORIENTED_EDGE('',*,*,#10762,.T.);
#15989=ORIENTED_EDGE('',*,*,#10878,.T.);
#15990=ORIENTED_EDGE('',*,*,#10879,.T.);
#15991=ORIENTED_EDGE('',*,*,#10880,.T.);
#15992=ORIENTED_EDGE('',*,*,#10881,.T.);
#15993=ORIENTED_EDGE('',*,*,#10882,.T.);
#15994=ORIENTED_EDGE('',*,*,#10873,.F.);
#15995=ORIENTED_EDGE('',*,*,#10759,.T.);
#15996=ORIENTED_EDGE('',*,*,#10883,.T.);
#15997=ORIENTED_EDGE('',*,*,#10884,.T.);
#15998=ORIENTED_EDGE('',*,*,#10885,.T.);
#15999=ORIENTED_EDGE('',*,*,#10677,.T.);
#16000=ORIENTED_EDGE('',*,*,#10676,.T.);
#16001=ORIENTED_EDGE('',*,*,#10675,.T.);
#16002=ORIENTED_EDGE('',*,*,#10674,.T.);
#16003=ORIENTED_EDGE('',*,*,#10673,.T.);
#16004=ORIENTED_EDGE('',*,*,#10672,.T.);
#16005=ORIENTED_EDGE('',*,*,#10671,.T.);
#16006=ORIENTED_EDGE('',*,*,#10886,.T.);
#16007=ORIENTED_EDGE('',*,*,#10687,.T.);
#16008=ORIENTED_EDGE('',*,*,#10686,.T.);
#16009=ORIENTED_EDGE('',*,*,#10685,.T.);
#16010=ORIENTED_EDGE('',*,*,#10684,.T.);
#16011=ORIENTED_EDGE('',*,*,#10683,.T.);
#16012=ORIENTED_EDGE('',*,*,#10682,.T.);
#16013=ORIENTED_EDGE('',*,*,#10681,.T.);
#16014=ORIENTED_EDGE('',*,*,#10887,.T.);
#16015=ORIENTED_EDGE('',*,*,#10697,.T.);
#16016=ORIENTED_EDGE('',*,*,#10696,.T.);
#16017=ORIENTED_EDGE('',*,*,#10695,.T.);
#16018=ORIENTED_EDGE('',*,*,#10694,.T.);
#16019=ORIENTED_EDGE('',*,*,#10693,.T.);
#16020=ORIENTED_EDGE('',*,*,#10692,.T.);
#16021=ORIENTED_EDGE('',*,*,#10691,.T.);
#16022=ORIENTED_EDGE('',*,*,#10888,.T.);
#16023=ORIENTED_EDGE('',*,*,#10707,.T.);
#16024=ORIENTED_EDGE('',*,*,#10706,.T.);
#16025=ORIENTED_EDGE('',*,*,#10705,.T.);
#16026=ORIENTED_EDGE('',*,*,#10704,.T.);
#16027=ORIENTED_EDGE('',*,*,#10703,.T.);
#16028=ORIENTED_EDGE('',*,*,#10702,.T.);
#16029=ORIENTED_EDGE('',*,*,#10701,.T.);
#16030=ORIENTED_EDGE('',*,*,#10889,.T.);
#16031=ORIENTED_EDGE('',*,*,#10717,.T.);
#16032=ORIENTED_EDGE('',*,*,#10716,.T.);
#16033=ORIENTED_EDGE('',*,*,#10715,.T.);
#16034=ORIENTED_EDGE('',*,*,#10714,.T.);
#16035=ORIENTED_EDGE('',*,*,#10713,.T.);
#16036=ORIENTED_EDGE('',*,*,#10712,.T.);
#16037=ORIENTED_EDGE('',*,*,#10711,.T.);
#16038=ORIENTED_EDGE('',*,*,#10890,.T.);
#16039=ORIENTED_EDGE('',*,*,#10891,.T.);
#16040=ORIENTED_EDGE('',*,*,#10892,.T.);
#16041=ORIENTED_EDGE('',*,*,#10893,.T.);
#16042=ORIENTED_EDGE('',*,*,#10894,.T.);
#16043=ORIENTED_EDGE('',*,*,#10895,.T.);
#16044=ORIENTED_EDGE('',*,*,#10731,.F.);
#16045=ORIENTED_EDGE('',*,*,#10827,.T.);
#16046=ORIENTED_EDGE('',*,*,#10733,.F.);
#16047=ORIENTED_EDGE('',*,*,#10896,.T.);
#16048=ORIENTED_EDGE('',*,*,#10897,.T.);
#16049=ORIENTED_EDGE('',*,*,#10828,.T.);
#16050=ORIENTED_EDGE('',*,*,#10898,.T.);
#16051=ORIENTED_EDGE('',*,*,#10899,.T.);
#16052=ORIENTED_EDGE('',*,*,#10900,.T.);
#16053=ORIENTED_EDGE('',*,*,#10901,.T.);
#16054=ORIENTED_EDGE('',*,*,#10902,.T.);
#16055=ORIENTED_EDGE('',*,*,#10903,.T.);
#16056=ORIENTED_EDGE('',*,*,#10904,.T.);
#16057=ORIENTED_EDGE('',*,*,#10905,.T.);
#16058=ORIENTED_EDGE('',*,*,#10906,.T.);
#16059=ORIENTED_EDGE('',*,*,#10907,.T.);
#16060=ORIENTED_EDGE('',*,*,#10908,.T.);
#16061=ORIENTED_EDGE('',*,*,#10909,.T.);
#16062=ORIENTED_EDGE('',*,*,#10910,.T.);
#16063=ORIENTED_EDGE('',*,*,#10911,.F.);
#16064=ORIENTED_EDGE('',*,*,#10912,.F.);
#16065=ORIENTED_EDGE('',*,*,#10913,.T.);
#16066=ORIENTED_EDGE('',*,*,#10914,.T.);
#16067=ORIENTED_EDGE('',*,*,#10915,.F.);
#16068=ORIENTED_EDGE('',*,*,#10916,.T.);
#16069=ORIENTED_EDGE('',*,*,#10917,.T.);
#16070=ORIENTED_EDGE('',*,*,#10918,.T.);
#16071=ORIENTED_EDGE('',*,*,#10913,.F.);
#16072=ORIENTED_EDGE('',*,*,#10919,.T.);
#16073=ORIENTED_EDGE('',*,*,#10915,.T.);
#16074=ORIENTED_EDGE('',*,*,#10920,.T.);
#16075=ORIENTED_EDGE('',*,*,#10921,.T.);
#16076=ORIENTED_EDGE('',*,*,#10922,.T.);
#16077=ORIENTED_EDGE('',*,*,#10923,.F.);
#16078=ORIENTED_EDGE('',*,*,#10924,.T.);
#16079=ORIENTED_EDGE('',*,*,#10925,.T.);
#16080=ORIENTED_EDGE('',*,*,#10926,.T.);
#16081=ORIENTED_EDGE('',*,*,#10861,.F.);
#16082=ORIENTED_EDGE('',*,*,#10927,.F.);
#16083=ORIENTED_EDGE('',*,*,#10928,.T.);
#16084=ORIENTED_EDGE('',*,*,#10923,.T.);
#16085=ORIENTED_EDGE('',*,*,#10860,.F.);
#16086=ORIENTED_EDGE('',*,*,#10929,.T.);
#16087=ORIENTED_EDGE('',*,*,#10930,.T.);
#16088=ORIENTED_EDGE('',*,*,#10931,.T.);
#16089=ORIENTED_EDGE('',*,*,#10927,.T.);
#16090=ORIENTED_EDGE('',*,*,#10859,.F.);
#16091=ORIENTED_EDGE('',*,*,#10932,.T.);
#16092=ORIENTED_EDGE('',*,*,#10933,.T.);
#16093=ORIENTED_EDGE('',*,*,#10934,.T.);
#16094=ORIENTED_EDGE('',*,*,#10935,.T.);
#16095=ORIENTED_EDGE('',*,*,#10936,.F.);
#16096=ORIENTED_EDGE('',*,*,#10866,.F.);
#16097=ORIENTED_EDGE('',*,*,#10936,.T.);
#16098=ORIENTED_EDGE('',*,*,#10937,.T.);
#16099=ORIENTED_EDGE('',*,*,#10938,.F.);
#16100=ORIENTED_EDGE('',*,*,#10867,.F.);
#16101=ORIENTED_EDGE('',*,*,#10938,.T.);
#16102=ORIENTED_EDGE('',*,*,#10939,.T.);
#16103=ORIENTED_EDGE('',*,*,#10940,.T.);
#16104=ORIENTED_EDGE('',*,*,#10941,.T.);
#16105=ORIENTED_EDGE('',*,*,#10942,.T.);
#16106=ORIENTED_EDGE('',*,*,#10863,.F.);
#16107=ORIENTED_EDGE('',*,*,#10943,.T.);
#16108=ORIENTED_EDGE('',*,*,#10944,.T.);
#16109=ORIENTED_EDGE('',*,*,#10945,.T.);
#16110=ORIENTED_EDGE('',*,*,#10881,.F.);
#16111=ORIENTED_EDGE('',*,*,#10946,.F.);
#16112=ORIENTED_EDGE('',*,*,#10942,.F.);
#16113=ORIENTED_EDGE('',*,*,#10883,.F.);
#16114=ORIENTED_EDGE('',*,*,#10864,.F.);
#16115=ORIENTED_EDGE('',*,*,#10946,.T.);
#16116=ORIENTED_EDGE('',*,*,#10947,.T.);
#16117=ORIENTED_EDGE('',*,*,#10948,.T.);
#16118=ORIENTED_EDGE('',*,*,#10949,.T.);
#16119=ORIENTED_EDGE('',*,*,#10929,.F.);
#16120=ORIENTED_EDGE('',*,*,#10950,.F.);
#16121=ORIENTED_EDGE('',*,*,#10871,.F.);
#16122=ORIENTED_EDGE('',*,*,#10870,.F.);
#16123=ORIENTED_EDGE('',*,*,#10858,.F.);
#16124=ORIENTED_EDGE('',*,*,#10872,.F.);
#16125=ORIENTED_EDGE('',*,*,#10950,.T.);
#16126=ORIENTED_EDGE('',*,*,#10951,.T.);
#16127=ORIENTED_EDGE('',*,*,#10952,.T.);
#16128=ORIENTED_EDGE('',*,*,#10953,.T.);
#16129=ORIENTED_EDGE('',*,*,#10880,.F.);
#16130=ORIENTED_EDGE('',*,*,#10879,.F.);
#16131=ORIENTED_EDGE('',*,*,#10954,.F.);
#16132=ORIENTED_EDGE('',*,*,#10926,.F.);
#16133=ORIENTED_EDGE('',*,*,#10878,.F.);
#16134=ORIENTED_EDGE('',*,*,#10862,.F.);
#16135=ORIENTED_EDGE('',*,*,#10954,.T.);
#16136=ORIENTED_EDGE('',*,*,#10865,.F.);
#16137=ORIENTED_EDGE('',*,*,#10877,.F.);
#16138=ORIENTED_EDGE('',*,*,#10955,.F.);
#16139=ORIENTED_EDGE('',*,*,#10956,.T.);
#16140=ORIENTED_EDGE('',*,*,#10957,.T.);
#16141=ORIENTED_EDGE('',*,*,#10958,.T.);
#16142=ORIENTED_EDGE('',*,*,#10932,.F.);
#16143=ORIENTED_EDGE('',*,*,#10955,.T.);
#16144=ORIENTED_EDGE('',*,*,#10876,.F.);
#16145=ORIENTED_EDGE('',*,*,#10823,.F.);
#16146=ORIENTED_EDGE('',*,*,#10959,.T.);
#16147=ORIENTED_EDGE('',*,*,#10754,.F.);
#16148=ORIENTED_EDGE('',*,*,#10960,.F.);
#16149=ORIENTED_EDGE('',*,*,#10824,.T.);
#16150=ORIENTED_EDGE('',*,*,#10960,.T.);
#16151=ORIENTED_EDGE('',*,*,#10961,.F.);
#16152=ORIENTED_EDGE('',*,*,#10962,.F.);
#16153=ORIENTED_EDGE('',*,*,#10757,.F.);
#16154=ORIENTED_EDGE('',*,*,#10963,.T.);
#16155=ORIENTED_EDGE('',*,*,#10891,.F.);
#16156=ORIENTED_EDGE('',*,*,#10961,.T.);
#16157=ORIENTED_EDGE('',*,*,#10962,.T.);
#16158=ORIENTED_EDGE('',*,*,#10890,.F.);
#16159=ORIENTED_EDGE('',*,*,#10964,.F.);
#16160=ORIENTED_EDGE('',*,*,#10825,.F.);
#16161=ORIENTED_EDGE('',*,*,#10892,.F.);
#16162=ORIENTED_EDGE('',*,*,#10965,.T.);
#16163=ORIENTED_EDGE('',*,*,#10744,.F.);
#16164=ORIENTED_EDGE('',*,*,#10966,.F.);
#16165=ORIENTED_EDGE('',*,*,#10964,.T.);
#16166=ORIENTED_EDGE('',*,*,#10893,.F.);
#16167=ORIENTED_EDGE('',*,*,#10967,.F.);
#16168=ORIENTED_EDGE('',*,*,#10894,.F.);
#16169=ORIENTED_EDGE('',*,*,#10826,.F.);
#16170=ORIENTED_EDGE('',*,*,#10966,.T.);
#16171=ORIENTED_EDGE('',*,*,#10743,.T.);
#16172=ORIENTED_EDGE('',*,*,#10968,.F.);
#16173=ORIENTED_EDGE('',*,*,#10967,.T.);
#16174=ORIENTED_EDGE('',*,*,#10968,.T.);
#16175=ORIENTED_EDGE('',*,*,#10742,.F.);
#16176=ORIENTED_EDGE('',*,*,#10969,.F.);
#16177=ORIENTED_EDGE('',*,*,#10895,.F.);
#16178=ORIENTED_EDGE('',*,*,#10969,.T.);
#16179=ORIENTED_EDGE('',*,*,#10741,.F.);
#16180=ORIENTED_EDGE('',*,*,#10970,.F.);
#16181=ORIENTED_EDGE('',*,*,#10732,.F.);
#16182=ORIENTED_EDGE('',*,*,#10970,.T.);
#16183=ORIENTED_EDGE('',*,*,#10740,.F.);
#16184=ORIENTED_EDGE('',*,*,#10971,.F.);
#16185=ORIENTED_EDGE('',*,*,#10896,.F.);
#16186=ORIENTED_EDGE('',*,*,#10971,.T.);
#16187=ORIENTED_EDGE('',*,*,#10739,.T.);
#16188=ORIENTED_EDGE('',*,*,#10972,.F.);
#16189=ORIENTED_EDGE('',*,*,#10973,.F.);
#16190=ORIENTED_EDGE('',*,*,#10738,.F.);
#16191=ORIENTED_EDGE('',*,*,#10753,.F.);
#16192=ORIENTED_EDGE('',*,*,#10974,.F.);
#16193=ORIENTED_EDGE('',*,*,#10727,.F.);
#16194=ORIENTED_EDGE('',*,*,#10972,.T.);
#16195=ORIENTED_EDGE('',*,*,#10973,.T.);
#16196=ORIENTED_EDGE('',*,*,#10730,.F.);
#16197=ORIENTED_EDGE('',*,*,#10975,.F.);
#16198=ORIENTED_EDGE('',*,*,#10829,.F.);
#16199=ORIENTED_EDGE('',*,*,#10897,.F.);
#16200=ORIENTED_EDGE('',*,*,#10974,.T.);
#16201=ORIENTED_EDGE('',*,*,#10752,.F.);
#16202=ORIENTED_EDGE('',*,*,#10976,.F.);
#16203=ORIENTED_EDGE('',*,*,#10728,.F.);
#16204=ORIENTED_EDGE('',*,*,#10975,.T.);
#16205=ORIENTED_EDGE('',*,*,#10729,.F.);
#16206=ORIENTED_EDGE('',*,*,#10977,.F.);
#16207=ORIENTED_EDGE('',*,*,#10830,.F.);
#16208=ORIENTED_EDGE('',*,*,#10977,.T.);
#16209=ORIENTED_EDGE('',*,*,#10976,.T.);
#16210=ORIENTED_EDGE('',*,*,#10978,.F.);
#16211=ORIENTED_EDGE('',*,*,#10831,.T.);
#16212=ORIENTED_EDGE('',*,*,#10751,.F.);
#16213=ORIENTED_EDGE('',*,*,#10979,.T.);
#16214=ORIENTED_EDGE('',*,*,#10821,.F.);
#16215=ORIENTED_EDGE('',*,*,#10978,.T.);
#16216=ORIENTED_EDGE('',*,*,#10958,.F.);
#16217=ORIENTED_EDGE('',*,*,#10980,.T.);
#16218=ORIENTED_EDGE('',*,*,#10903,.F.);
#16219=ORIENTED_EDGE('',*,*,#10981,.F.);
#16220=ORIENTED_EDGE('',*,*,#10982,.F.);
#16221=ORIENTED_EDGE('',*,*,#10782,.F.);
#16222=ORIENTED_EDGE('',*,*,#10983,.F.);
#16223=ORIENTED_EDGE('',*,*,#10792,.F.);
#16224=ORIENTED_EDGE('',*,*,#10904,.F.);
#16225=ORIENTED_EDGE('',*,*,#10984,.T.);
#16226=ORIENTED_EDGE('',*,*,#10985,.T.);
#16227=ORIENTED_EDGE('',*,*,#10839,.F.);
#16228=ORIENTED_EDGE('',*,*,#10986,.F.);
#16229=ORIENTED_EDGE('',*,*,#10981,.T.);
#16230=ORIENTED_EDGE('',*,*,#10902,.F.);
#16231=ORIENTED_EDGE('',*,*,#10901,.F.);
#16232=ORIENTED_EDGE('',*,*,#10987,.F.);
#16233=ORIENTED_EDGE('',*,*,#10935,.F.);
#16234=ORIENTED_EDGE('',*,*,#10934,.F.);
#16235=ORIENTED_EDGE('',*,*,#10933,.F.);
#16236=ORIENTED_EDGE('',*,*,#10983,.T.);
#16237=ORIENTED_EDGE('',*,*,#10785,.F.);
#16238=ORIENTED_EDGE('',*,*,#10988,.F.);
#16239=ORIENTED_EDGE('',*,*,#10793,.F.);
#16240=ORIENTED_EDGE('',*,*,#10982,.T.);
#16241=ORIENTED_EDGE('',*,*,#10791,.F.);
#16242=ORIENTED_EDGE('',*,*,#10989,.F.);
#16243=ORIENTED_EDGE('',*,*,#10845,.F.);
#16244=ORIENTED_EDGE('',*,*,#10990,.F.);
#16245=ORIENTED_EDGE('',*,*,#10846,.F.);
#16246=ORIENTED_EDGE('',*,*,#10991,.F.);
#16247=ORIENTED_EDGE('',*,*,#10917,.F.);
#16248=ORIENTED_EDGE('',*,*,#10847,.T.);
#16249=ORIENTED_EDGE('',*,*,#10990,.T.);
#16250=ORIENTED_EDGE('',*,*,#10992,.F.);
#16251=ORIENTED_EDGE('',*,*,#10986,.T.);
#16252=ORIENTED_EDGE('',*,*,#10987,.T.);
#16253=ORIENTED_EDGE('',*,*,#10900,.F.);
#16254=ORIENTED_EDGE('',*,*,#10993,.F.);
#16255=ORIENTED_EDGE('',*,*,#10937,.F.);
#16256=ORIENTED_EDGE('',*,*,#10988,.T.);
#16257=ORIENTED_EDGE('',*,*,#10787,.F.);
#16258=ORIENTED_EDGE('',*,*,#10994,.F.);
#16259=ORIENTED_EDGE('',*,*,#10794,.F.);
#16260=ORIENTED_EDGE('',*,*,#10991,.T.);
#16261=ORIENTED_EDGE('',*,*,#10989,.T.);
#16262=ORIENTED_EDGE('',*,*,#10995,.F.);
#16263=ORIENTED_EDGE('',*,*,#10992,.T.);
#16264=ORIENTED_EDGE('',*,*,#10919,.F.);
#16265=ORIENTED_EDGE('',*,*,#10996,.F.);
#16266=ORIENTED_EDGE('',*,*,#10905,.F.);
#16267=ORIENTED_EDGE('',*,*,#10993,.T.);
#16268=ORIENTED_EDGE('',*,*,#10899,.F.);
#16269=ORIENTED_EDGE('',*,*,#10898,.F.);
#16270=ORIENTED_EDGE('',*,*,#10997,.F.);
#16271=ORIENTED_EDGE('',*,*,#10941,.F.);
#16272=ORIENTED_EDGE('',*,*,#10940,.F.);
#16273=ORIENTED_EDGE('',*,*,#10939,.F.);
#16274=ORIENTED_EDGE('',*,*,#10994,.T.);
#16275=ORIENTED_EDGE('',*,*,#10778,.F.);
#16276=ORIENTED_EDGE('',*,*,#10998,.F.);
#16277=ORIENTED_EDGE('',*,*,#10795,.F.);
#16278=ORIENTED_EDGE('',*,*,#10995,.T.);
#16279=ORIENTED_EDGE('',*,*,#10790,.F.);
#16280=ORIENTED_EDGE('',*,*,#10999,.F.);
#16281=ORIENTED_EDGE('',*,*,#10918,.F.);
#16282=ORIENTED_EDGE('',*,*,#10996,.T.);
#16283=ORIENTED_EDGE('',*,*,#10916,.F.);
#16284=ORIENTED_EDGE('',*,*,#11000,.F.);
#16285=ORIENTED_EDGE('',*,*,#10906,.F.);
#16286=ORIENTED_EDGE('',*,*,#10909,.F.);
#16287=ORIENTED_EDGE('',*,*,#11001,.T.);
#16288=ORIENTED_EDGE('',*,*,#10943,.F.);
#16289=ORIENTED_EDGE('',*,*,#10997,.T.);
#16290=ORIENTED_EDGE('',*,*,#10998,.T.);
#16291=ORIENTED_EDGE('',*,*,#10775,.F.);
#16292=ORIENTED_EDGE('',*,*,#11002,.F.);
#16293=ORIENTED_EDGE('',*,*,#10796,.F.);
#16294=ORIENTED_EDGE('',*,*,#10999,.T.);
#16295=ORIENTED_EDGE('',*,*,#10789,.F.);
#16296=ORIENTED_EDGE('',*,*,#11003,.F.);
#16297=ORIENTED_EDGE('',*,*,#10914,.F.);
#16298=ORIENTED_EDGE('',*,*,#11000,.T.);
#16299=ORIENTED_EDGE('',*,*,#10922,.F.);
#16300=ORIENTED_EDGE('',*,*,#11004,.F.);
#16301=ORIENTED_EDGE('',*,*,#10907,.F.);
#16302=ORIENTED_EDGE('',*,*,#11005,.T.);
#16303=ORIENTED_EDGE('',*,*,#11006,.T.);
#16304=ORIENTED_EDGE('',*,*,#10908,.F.);
#16305=ORIENTED_EDGE('',*,*,#11007,.F.);
#16306=ORIENTED_EDGE('',*,*,#10854,.F.);
#16307=ORIENTED_EDGE('',*,*,#11002,.T.);
#16308=ORIENTED_EDGE('',*,*,#10857,.F.);
#16309=ORIENTED_EDGE('',*,*,#11008,.F.);
#16310=ORIENTED_EDGE('',*,*,#10797,.F.);
#16311=ORIENTED_EDGE('',*,*,#11003,.T.);
#16312=ORIENTED_EDGE('',*,*,#10788,.F.);
#16313=ORIENTED_EDGE('',*,*,#11009,.F.);
#16314=ORIENTED_EDGE('',*,*,#10920,.F.);
#16315=ORIENTED_EDGE('',*,*,#11007,.T.);
#16316=ORIENTED_EDGE('',*,*,#11004,.T.);
#16317=ORIENTED_EDGE('',*,*,#11010,.F.);
#16318=ORIENTED_EDGE('',*,*,#10855,.T.);
#16319=ORIENTED_EDGE('',*,*,#11009,.T.);
#16320=ORIENTED_EDGE('',*,*,#11008,.T.);
#16321=ORIENTED_EDGE('',*,*,#11011,.F.);
#16322=ORIENTED_EDGE('',*,*,#11010,.T.);
#16323=ORIENTED_EDGE('',*,*,#10921,.F.);
#16324=ORIENTED_EDGE('',*,*,#11011,.T.);
#16325=ORIENTED_EDGE('',*,*,#10856,.F.);
#16326=ORIENTED_EDGE('',*,*,#11012,.F.);
#16327=ORIENTED_EDGE('',*,*,#10723,.F.);
#16328=ORIENTED_EDGE('',*,*,#11013,.T.);
#16329=ORIENTED_EDGE('',*,*,#10832,.F.);
#16330=ORIENTED_EDGE('',*,*,#11013,.F.);
#16331=ORIENTED_EDGE('',*,*,#10722,.F.);
#16332=ORIENTED_EDGE('',*,*,#10833,.F.);
#16333=ORIENTED_EDGE('',*,*,#11014,.T.);
#16334=ORIENTED_EDGE('',*,*,#10837,.F.);
#16335=ORIENTED_EDGE('',*,*,#10838,.F.);
#16336=ORIENTED_EDGE('',*,*,#11014,.F.);
#16337=ORIENTED_EDGE('',*,*,#10810,.F.);
#16338=ORIENTED_EDGE('',*,*,#11015,.T.);
#16339=ORIENTED_EDGE('',*,*,#10951,.F.);
#16340=ORIENTED_EDGE('',*,*,#11016,.F.);
#16341=ORIENTED_EDGE('',*,*,#11017,.T.);
#16342=ORIENTED_EDGE('',*,*,#11018,.T.);
#16343=ORIENTED_EDGE('',*,*,#10809,.F.);
#16344=ORIENTED_EDGE('',*,*,#11019,.F.);
#16345=ORIENTED_EDGE('',*,*,#10844,.F.);
#16346=ORIENTED_EDGE('',*,*,#11016,.T.);
#16347=ORIENTED_EDGE('',*,*,#10925,.F.);
#16348=ORIENTED_EDGE('',*,*,#10924,.F.);
#16349=ORIENTED_EDGE('',*,*,#11020,.F.);
#16350=ORIENTED_EDGE('',*,*,#10811,.F.);
#16351=ORIENTED_EDGE('',*,*,#11019,.T.);
#16352=ORIENTED_EDGE('',*,*,#10808,.F.);
#16353=ORIENTED_EDGE('',*,*,#11021,.F.);
#16354=ORIENTED_EDGE('',*,*,#10780,.F.);
#16355=ORIENTED_EDGE('',*,*,#11020,.T.);
#16356=ORIENTED_EDGE('',*,*,#10928,.F.);
#16357=ORIENTED_EDGE('',*,*,#11022,.F.);
#16358=ORIENTED_EDGE('',*,*,#10812,.F.);
#16359=ORIENTED_EDGE('',*,*,#11021,.T.);
#16360=ORIENTED_EDGE('',*,*,#10807,.F.);
#16361=ORIENTED_EDGE('',*,*,#11023,.F.);
#16362=ORIENTED_EDGE('',*,*,#10783,.F.);
#16363=ORIENTED_EDGE('',*,*,#11022,.T.);
#16364=ORIENTED_EDGE('',*,*,#10931,.F.);
#16365=ORIENTED_EDGE('',*,*,#10930,.F.);
#16366=ORIENTED_EDGE('',*,*,#11024,.F.);
#16367=ORIENTED_EDGE('',*,*,#10801,.F.);
#16368=ORIENTED_EDGE('',*,*,#11023,.T.);
#16369=ORIENTED_EDGE('',*,*,#10806,.F.);
#16370=ORIENTED_EDGE('',*,*,#11025,.F.);
#16371=ORIENTED_EDGE('',*,*,#10786,.F.);
#16372=ORIENTED_EDGE('',*,*,#10949,.F.);
#16373=ORIENTED_EDGE('',*,*,#11026,.T.);
#16374=ORIENTED_EDGE('',*,*,#10802,.F.);
#16375=ORIENTED_EDGE('',*,*,#11024,.T.);
#16376=ORIENTED_EDGE('',*,*,#11025,.T.);
#16377=ORIENTED_EDGE('',*,*,#10805,.F.);
#16378=ORIENTED_EDGE('',*,*,#11027,.F.);
#16379=ORIENTED_EDGE('',*,*,#10777,.F.);
#16380=ORIENTED_EDGE('',*,*,#10803,.F.);
#16381=ORIENTED_EDGE('',*,*,#11028,.T.);
#16382=ORIENTED_EDGE('',*,*,#11029,.T.);
#16383=ORIENTED_EDGE('',*,*,#10848,.F.);
#16384=ORIENTED_EDGE('',*,*,#11030,.F.);
#16385=ORIENTED_EDGE('',*,*,#11027,.T.);
#16386=ORIENTED_EDGE('',*,*,#10804,.F.);
#16387=ORIENTED_EDGE('',*,*,#11030,.T.);
#16388=ORIENTED_EDGE('',*,*,#10773,.F.);
#16389=ORIENTED_EDGE('',*,*,#11031,.F.);
#16390=ORIENTED_EDGE('',*,*,#10816,.F.);
#16391=ORIENTED_EDGE('',*,*,#11032,.F.);
#16392=ORIENTED_EDGE('',*,*,#10813,.F.);
#16393=ORIENTED_EDGE('',*,*,#11032,.T.);
#16394=ORIENTED_EDGE('',*,*,#10819,.F.);
#16395=ORIENTED_EDGE('',*,*,#11031,.T.);
#16396=ORIENTED_EDGE('',*,*,#10814,.F.);
#16397=ORIENTED_EDGE('',*,*,#10834,.F.);
#16398=ORIENTED_EDGE('',*,*,#10835,.F.);
#16399=ORIENTED_EDGE('',*,*,#11033,.T.);
#16400=ORIENTED_EDGE('',*,*,#10800,.F.);
#16401=ORIENTED_EDGE('',*,*,#11033,.F.);
#16402=ORIENTED_EDGE('',*,*,#10726,.F.);
#16403=ORIENTED_EDGE('',*,*,#11034,.T.);
#16404=ORIENTED_EDGE('',*,*,#10910,.F.);
#16405=ORIENTED_EDGE('',*,*,#11034,.F.);
#16406=ORIENTED_EDGE('',*,*,#10965,.F.);
#16407=ORIENTED_EDGE('',*,*,#10963,.F.);
#16408=ORIENTED_EDGE('',*,*,#11035,.F.);
#16409=ORIENTED_EDGE('',*,*,#11036,.F.);
#16410=ORIENTED_EDGE('',*,*,#10822,.F.);
#16411=ORIENTED_EDGE('',*,*,#11037,.F.);
#16412=ORIENTED_EDGE('',*,*,#10720,.F.);
#16413=ORIENTED_EDGE('',*,*,#10959,.F.);
#16414=ORIENTED_EDGE('',*,*,#11036,.T.);
#16415=ORIENTED_EDGE('',*,*,#11038,.F.);
#16416=ORIENTED_EDGE('',*,*,#11037,.T.);
#16417=ORIENTED_EDGE('',*,*,#10979,.F.);
#16418=ORIENTED_EDGE('',*,*,#11039,.F.);
#16419=ORIENTED_EDGE('',*,*,#11038,.T.);
#16420=ORIENTED_EDGE('',*,*,#10719,.F.);
#16421=ORIENTED_EDGE('',*,*,#11040,.F.);
#16422=ORIENTED_EDGE('',*,*,#10755,.F.);
#16423=ORIENTED_EDGE('',*,*,#11035,.T.);
#16424=ORIENTED_EDGE('',*,*,#10756,.F.);
#16425=ORIENTED_EDGE('',*,*,#11041,.F.);
#16426=ORIENTED_EDGE('',*,*,#10735,.F.);
#16427=ORIENTED_EDGE('',*,*,#10750,.F.);
#16428=ORIENTED_EDGE('',*,*,#11042,.F.);
#16429=ORIENTED_EDGE('',*,*,#10721,.F.);
#16430=ORIENTED_EDGE('',*,*,#11039,.T.);
#16431=ORIENTED_EDGE('',*,*,#11040,.T.);
#16432=ORIENTED_EDGE('',*,*,#10718,.T.);
#16433=ORIENTED_EDGE('',*,*,#11043,.F.);
#16434=ORIENTED_EDGE('',*,*,#11041,.T.);
#16435=ORIENTED_EDGE('',*,*,#10749,.F.);
#16436=ORIENTED_EDGE('',*,*,#10736,.F.);
#16437=ORIENTED_EDGE('',*,*,#11043,.T.);
#16438=ORIENTED_EDGE('',*,*,#11012,.T.);
#16439=ORIENTED_EDGE('',*,*,#11042,.T.);
#16440=ORIENTED_EDGE('',*,*,#10708,.T.);
#16441=ORIENTED_EDGE('',*,*,#10889,.F.);
#16442=ORIENTED_EDGE('',*,*,#10710,.F.);
#16443=ORIENTED_EDGE('',*,*,#10767,.F.);
#16444=ORIENTED_EDGE('',*,*,#10698,.T.);
#16445=ORIENTED_EDGE('',*,*,#10888,.F.);
#16446=ORIENTED_EDGE('',*,*,#10700,.F.);
#16447=ORIENTED_EDGE('',*,*,#10768,.F.);
#16448=ORIENTED_EDGE('',*,*,#10688,.T.);
#16449=ORIENTED_EDGE('',*,*,#10887,.F.);
#16450=ORIENTED_EDGE('',*,*,#10690,.F.);
#16451=ORIENTED_EDGE('',*,*,#10769,.F.);
#16452=ORIENTED_EDGE('',*,*,#10678,.T.);
#16453=ORIENTED_EDGE('',*,*,#10886,.F.);
#16454=ORIENTED_EDGE('',*,*,#10680,.F.);
#16455=ORIENTED_EDGE('',*,*,#10770,.F.);
#16456=ORIENTED_EDGE('',*,*,#10668,.T.);
#16457=ORIENTED_EDGE('',*,*,#10885,.F.);
#16458=ORIENTED_EDGE('',*,*,#10670,.F.);
#16459=ORIENTED_EDGE('',*,*,#10771,.F.);
#16460=ORIENTED_EDGE('',*,*,#11015,.F.);
#16461=ORIENTED_EDGE('',*,*,#11018,.F.);
#16462=ORIENTED_EDGE('',*,*,#11044,.F.);
#16463=ORIENTED_EDGE('',*,*,#11044,.T.);
#16464=ORIENTED_EDGE('',*,*,#11017,.F.);
#16465=ORIENTED_EDGE('',*,*,#11045,.F.);
#16466=ORIENTED_EDGE('',*,*,#10952,.F.);
#16467=ORIENTED_EDGE('',*,*,#11045,.T.);
#16468=ORIENTED_EDGE('',*,*,#10843,.F.);
#16469=ORIENTED_EDGE('',*,*,#11046,.F.);
#16470=ORIENTED_EDGE('',*,*,#10953,.F.);
#16471=ORIENTED_EDGE('',*,*,#11046,.T.);
#16472=ORIENTED_EDGE('',*,*,#10842,.F.);
#16473=ORIENTED_EDGE('',*,*,#11047,.F.);
#16474=ORIENTED_EDGE('',*,*,#10874,.F.);
#16475=ORIENTED_EDGE('',*,*,#11047,.T.);
#16476=ORIENTED_EDGE('',*,*,#10841,.F.);
#16477=ORIENTED_EDGE('',*,*,#11048,.F.);
#16478=ORIENTED_EDGE('',*,*,#10875,.F.);
#16479=ORIENTED_EDGE('',*,*,#11048,.T.);
#16480=ORIENTED_EDGE('',*,*,#10840,.F.);
#16481=ORIENTED_EDGE('',*,*,#11049,.F.);
#16482=ORIENTED_EDGE('',*,*,#10956,.F.);
#16483=ORIENTED_EDGE('',*,*,#11049,.T.);
#16484=ORIENTED_EDGE('',*,*,#10985,.F.);
#16485=ORIENTED_EDGE('',*,*,#11050,.F.);
#16486=ORIENTED_EDGE('',*,*,#10957,.F.);
#16487=ORIENTED_EDGE('',*,*,#10984,.F.);
#16488=ORIENTED_EDGE('',*,*,#10980,.F.);
#16489=ORIENTED_EDGE('',*,*,#11050,.T.);
#16490=ORIENTED_EDGE('',*,*,#11001,.F.);
#16491=ORIENTED_EDGE('',*,*,#11006,.F.);
#16492=ORIENTED_EDGE('',*,*,#11051,.F.);
#16493=ORIENTED_EDGE('',*,*,#11051,.T.);
#16494=ORIENTED_EDGE('',*,*,#11005,.F.);
#16495=ORIENTED_EDGE('',*,*,#11052,.F.);
#16496=ORIENTED_EDGE('',*,*,#10944,.F.);
#16497=ORIENTED_EDGE('',*,*,#11052,.T.);
#16498=ORIENTED_EDGE('',*,*,#10853,.F.);
#16499=ORIENTED_EDGE('',*,*,#11053,.F.);
#16500=ORIENTED_EDGE('',*,*,#10945,.F.);
#16501=ORIENTED_EDGE('',*,*,#11053,.T.);
#16502=ORIENTED_EDGE('',*,*,#10852,.F.);
#16503=ORIENTED_EDGE('',*,*,#11054,.F.);
#16504=ORIENTED_EDGE('',*,*,#10882,.F.);
#16505=ORIENTED_EDGE('',*,*,#11054,.T.);
#16506=ORIENTED_EDGE('',*,*,#10851,.F.);
#16507=ORIENTED_EDGE('',*,*,#11055,.F.);
#16508=ORIENTED_EDGE('',*,*,#10868,.F.);
#16509=ORIENTED_EDGE('',*,*,#11055,.T.);
#16510=ORIENTED_EDGE('',*,*,#10850,.F.);
#16511=ORIENTED_EDGE('',*,*,#11056,.F.);
#16512=ORIENTED_EDGE('',*,*,#10869,.F.);
#16513=ORIENTED_EDGE('',*,*,#11056,.T.);
#16514=ORIENTED_EDGE('',*,*,#10849,.F.);
#16515=ORIENTED_EDGE('',*,*,#11057,.F.);
#16516=ORIENTED_EDGE('',*,*,#10947,.F.);
#16517=ORIENTED_EDGE('',*,*,#11057,.T.);
#16518=ORIENTED_EDGE('',*,*,#11029,.F.);
#16519=ORIENTED_EDGE('',*,*,#11058,.F.);
#16520=ORIENTED_EDGE('',*,*,#10948,.F.);
#16521=ORIENTED_EDGE('',*,*,#11028,.F.);
#16522=ORIENTED_EDGE('',*,*,#11026,.F.);
#16523=ORIENTED_EDGE('',*,*,#11058,.T.);
#16524=ORIENTED_EDGE('',*,*,#10912,.T.);
#16525=ORIENTED_EDGE('',*,*,#11059,.T.);
#16526=ORIENTED_EDGE('',*,*,#10748,.F.);
#16527=ORIENTED_EDGE('',*,*,#11059,.F.);
#16528=ORIENTED_EDGE('',*,*,#10911,.T.);
#16529=ORIENTED_EDGE('',*,*,#11060,.T.);
#16530=ORIENTED_EDGE('',*,*,#10747,.F.);
#16531=ORIENTED_EDGE('',*,*,#11060,.F.);
#16532=ORIENTED_EDGE('',*,*,#10799,.T.);
#16533=ORIENTED_EDGE('',*,*,#11061,.T.);
#16534=ORIENTED_EDGE('',*,*,#10746,.F.);
#16535=ORIENTED_EDGE('',*,*,#11061,.F.);
#16536=ORIENTED_EDGE('',*,*,#10798,.T.);
#16537=ORIENTED_EDGE('',*,*,#11062,.T.);
#16538=ORIENTED_EDGE('',*,*,#10745,.F.);
#16539=ORIENTED_EDGE('',*,*,#11062,.F.);
#16540=ORIENTED_EDGE('',*,*,#10884,.F.);
#16541=ORIENTED_EDGE('',*,*,#11063,.T.);
#16542=ORIENTED_EDGE('',*,*,#10764,.F.);
#16543=ORIENTED_EDGE('',*,*,#10765,.F.);
#16544=ORIENTED_EDGE('',*,*,#11063,.F.);
#16645=PLANE('',#19307);
#16646=PLANE('',#19337);
#16647=PLANE('',#19341);
#16648=PLANE('',#19345);
#16649=PLANE('',#19353);
#16650=PLANE('',#19365);
#16651=PLANE('',#19377);
#16652=PLANE('',#19385);
#16653=PLANE('',#19387);
#16654=PLANE('',#19389);
#16655=PLANE('',#19403);
#16656=PLANE('',#19411);
#16657=PLANE('',#19412);
#17506=ADVANCED_FACE('',(#4390),#1707,.T.);
#17507=ADVANCED_FACE('',(#4391),#1708,.T.);
#17508=ADVANCED_FACE('',(#4392),#1709,.T.);
#17509=ADVANCED_FACE('',(#4393),#1710,.T.);
#17510=ADVANCED_FACE('',(#4394),#1711,.T.);
#17511=ADVANCED_FACE('',(#4395),#3425,.F.);
#17512=ADVANCED_FACE('',(#4396),#3426,.F.);
#17513=ADVANCED_FACE('',(#4397),#3427,.F.);
#17514=ADVANCED_FACE('',(#4398),#3428,.F.);
#17515=ADVANCED_FACE('',(#4399,#3524,#3525,#3526,#3527,#3528),#16645,.F.);
#17516=ADVANCED_FACE('',(#4400),#3429,.F.);
#17517=ADVANCED_FACE('',(#4401),#3430,.F.);
#17518=ADVANCED_FACE('',(#4402,#3529,#3530,#3531,#3532,#3533),#3431,.T.);
#17519=ADVANCED_FACE('',(#4403),#3432,.T.);
#17520=ADVANCED_FACE('',(#4404),#16646,.T.);
#17521=ADVANCED_FACE('',(#4405),#3433,.T.);
#17522=ADVANCED_FACE('',(#4406),#16647,.F.);
#17523=ADVANCED_FACE('',(#4407),#3434,.T.);
#17524=ADVANCED_FACE('',(#4408,#3534,#3535,#3536),#16648,.T.);
#17525=ADVANCED_FACE('',(#4409,#3537),#16649,.F.);
#17526=ADVANCED_FACE('',(#4410),#3435,.F.);
#17527=ADVANCED_FACE('',(#4411),#3436,.F.);
#17528=ADVANCED_FACE('',(#4412,#3538),#16650,.F.);
#17529=ADVANCED_FACE('',(#4413,#3539),#16651,.F.);
#17530=ADVANCED_FACE('',(#4414),#3437,.F.);
#17531=ADVANCED_FACE('',(#4415),#16652,.F.);
#17532=ADVANCED_FACE('',(#4416),#16653,.F.);
#17533=ADVANCED_FACE('',(#4417),#337,.T.);
#17534=ADVANCED_FACE('',(#4418),#338,.T.);
#17535=ADVANCED_FACE('',(#4419),#339,.T.);
#17536=ADVANCED_FACE('',(#4420),#340,.T.);
#17537=ADVANCED_FACE('',(#4421),#341,.T.);
#17538=ADVANCED_FACE('',(#4422),#16654,.T.);
#17539=ADVANCED_FACE('',(#4423),#160,.F.);
#17540=ADVANCED_FACE('',(#4424),#161,.F.);
#17541=ADVANCED_FACE('',(#4425),#162,.F.);
#17542=ADVANCED_FACE('',(#4426),#163,.F.);
#17543=ADVANCED_FACE('',(#4427),#164,.F.);
#17544=ADVANCED_FACE('',(#4428),#3438,.F.);
#17545=ADVANCED_FACE('',(#4429),#3439,.F.);
#17546=ADVANCED_FACE('',(#4430),#3440,.F.);
#17547=ADVANCED_FACE('',(#4431,#3540,#3541,#3542),#16655,.T.);
#17548=ADVANCED_FACE('',(#4432),#3441,.F.);
#17549=ADVANCED_FACE('',(#4433),#16656,.F.);
#17550=ADVANCED_FACE('',(#4434),#16657,.F.);
#17551=ADVANCED_FACE('',(#4435),#1712,.F.);
#17552=ADVANCED_FACE('',(#4436),#1713,.F.);
#17553=ADVANCED_FACE('',(#4437),#1714,.F.);
#17554=ADVANCED_FACE('',(#4438),#1715,.F.);
#17555=ADVANCED_FACE('',(#4439),#1716,.F.);
#17556=ADVANCED_FACE('',(#4440),#1717,.F.);
#17557=ADVANCED_FACE('',(#4441),#1718,.T.);
#17558=ADVANCED_FACE('',(#4442),#283,.F.);
#17559=ADVANCED_FACE('',(#4443),#1719,.T.);
#17560=ADVANCED_FACE('',(#4444),#284,.F.);
#17561=ADVANCED_FACE('',(#4445),#342,.T.);
#17562=ADVANCED_FACE('',(#4446),#285,.F.);
#17563=ADVANCED_FACE('',(#4447),#286,.F.);
#17564=ADVANCED_FACE('',(#4448),#1720,.T.);
#17565=ADVANCED_FACE('',(#4449),#287,.T.);
#17566=ADVANCED_FACE('',(#4450),#288,.T.);
#17567=ADVANCED_FACE('',(#4451),#3442,.F.);
#17568=ADVANCED_FACE('',(#4452),#289,.T.);
#17569=ADVANCED_FACE('',(#4453),#290,.F.);
#17570=ADVANCED_FACE('',(#4454),#3443,.T.);
#17571=ADVANCED_FACE('',(#4455),#291,.F.);
#17572=ADVANCED_FACE('',(#4456),#292,.F.);
#17573=ADVANCED_FACE('',(#4457),#293,.F.);
#17574=ADVANCED_FACE('',(#4458),#294,.F.);
#17575=ADVANCED_FACE('',(#4459),#295,.F.);
#17576=ADVANCED_FACE('',(#4460),#296,.F.);
#17577=ADVANCED_FACE('',(#4461),#3444,.T.);
#17578=ADVANCED_FACE('',(#4462),#3445,.F.);
#17579=ADVANCED_FACE('',(#4463),#297,.T.);
#17580=ADVANCED_FACE('',(#4464),#298,.T.);
#17581=ADVANCED_FACE('',(#4465),#299,.T.);
#17582=ADVANCED_FACE('',(#4466),#1721,.T.);
#17583=ADVANCED_FACE('',(#4467),#300,.T.);
#17584=ADVANCED_FACE('',(#4468),#3446,.T.);
#17585=ADVANCED_FACE('',(#4469),#301,.F.);
#17586=ADVANCED_FACE('',(#4470),#3447,.T.);
#17587=ADVANCED_FACE('',(#4471),#3448,.T.);
#17588=ADVANCED_FACE('',(#4472),#3449,.T.);
#17589=ADVANCED_FACE('',(#4473),#1722,.T.);
#17590=ADVANCED_FACE('',(#4474),#302,.T.);
#17591=ADVANCED_FACE('',(#4475),#303,.T.);
#17592=ADVANCED_FACE('',(#4476),#165,.T.);
#17593=ADVANCED_FACE('',(#4477),#3450,.F.);
#17594=ADVANCED_FACE('',(#4478),#304,.F.);
#17595=ADVANCED_FACE('',(#4479),#3451,.T.);
#17596=ADVANCED_FACE('',(#4480),#3452,.T.);
#17597=ADVANCED_FACE('',(#4481),#305,.F.);
#17598=ADVANCED_FACE('',(#4482),#1723,.T.);
#17599=ADVANCED_FACE('',(#4483),#306,.T.);
#17600=ADVANCED_FACE('',(#4484),#307,.T.);
#17601=ADVANCED_FACE('',(#4485),#3453,.F.);
#17602=ADVANCED_FACE('',(#4486),#3454,.T.);
#17603=ADVANCED_FACE('',(#4487),#3455,.T.);
#17604=ADVANCED_FACE('',(#4488),#3456,.T.);
#17605=ADVANCED_FACE('',(#4489),#1724,.T.);
#17606=ADVANCED_FACE('',(#4490),#166,.T.);
#17607=ADVANCED_FACE('',(#4491),#3457,.T.);
#17608=ADVANCED_FACE('',(#4492),#308,.F.);
#17609=ADVANCED_FACE('',(#4493),#309,.T.);
#17610=ADVANCED_FACE('',(#4494),#1725,.T.);
#17611=ADVANCED_FACE('',(#4495),#3458,.T.);
#17612=ADVANCED_FACE('',(#4496),#1726,.T.);
#17613=ADVANCED_FACE('',(#4497),#310,.T.);
#17614=ADVANCED_FACE('',(#4498),#311,.T.);
#17615=ADVANCED_FACE('',(#4499),#3459,.T.);
#17616=ADVANCED_FACE('',(#4500),#1727,.T.);
#17617=ADVANCED_FACE('',(#4501),#312,.T.);
#17618=ADVANCED_FACE('',(#4502),#1728,.T.);
#17619=ADVANCED_FACE('',(#4503),#3460,.T.);
#17620=ADVANCED_FACE('',(#4504),#3461,.T.);
#17621=ADVANCED_FACE('',(#4505),#313,.T.);
#17622=ADVANCED_FACE('',(#4506),#314,.T.);
#17623=ADVANCED_FACE('',(#4507),#315,.T.);
#17624=ADVANCED_FACE('',(#4508),#316,.T.);
#17625=ADVANCED_FACE('',(#4509),#317,.T.);
#17626=ADVANCED_FACE('',(#4510),#167,.F.);
#17627=ADVANCED_FACE('',(#4511),#318,.T.);
#17628=ADVANCED_FACE('',(#4512),#168,.T.);
#17629=ADVANCED_FACE('',(#4513),#169,.T.);
#17630=ADVANCED_FACE('',(#4514),#3462,.T.);
#17631=ADVANCED_FACE('',(#4515),#319,.F.);
#17632=ADVANCED_FACE('',(#4516),#3463,.T.);
#17633=ADVANCED_FACE('',(#4517),#1729,.T.);
#17634=ADVANCED_FACE('',(#4518),#320,.T.);
#17635=ADVANCED_FACE('',(#4519),#1730,.T.);
#17636=ADVANCED_FACE('',(#4520),#1731,.T.);
#17637=ADVANCED_FACE('',(#4521),#1732,.T.);
#17638=ADVANCED_FACE('',(#4522),#1733,.T.);
#17639=ADVANCED_FACE('',(#4523),#1734,.T.);
#17640=ADVANCED_FACE('',(#4524),#321,.F.);
#17641=ADVANCED_FACE('',(#4525),#1735,.F.);
#17642=ADVANCED_FACE('',(#4526),#1736,.F.);
#17643=ADVANCED_FACE('',(#4527),#3464,.F.);
#17644=ADVANCED_FACE('',(#4528),#3465,.F.);
#17645=ADVANCED_FACE('',(#4529),#1737,.F.);
#17646=ADVANCED_FACE('',(#4530),#1738,.F.);
#17647=ADVANCED_FACE('',(#4531),#3466,.T.);
#17648=ADVANCED_FACE('',(#4532),#3467,.T.);
#17649=ADVANCED_FACE('',(#4533),#1739,.F.);
#17650=ADVANCED_FACE('',(#4534),#1740,.F.);
#17651=ADVANCED_FACE('',(#4535),#3468,.F.);
#17652=ADVANCED_FACE('',(#4536),#3469,.F.);
#17653=ADVANCED_FACE('',(#4537),#3470,.F.);
#17654=ADVANCED_FACE('',(#4538),#1741,.F.);
#17655=ADVANCED_FACE('',(#4539),#1742,.F.);
#17656=ADVANCED_FACE('',(#4540),#3471,.T.);
#17657=ADVANCED_FACE('',(#4541),#3472,.F.);
#17658=ADVANCED_FACE('',(#4542),#3473,.F.);
#17659=ADVANCED_FACE('',(#4543),#3474,.F.);
#17660=ADVANCED_FACE('',(#4544),#3475,.F.);
#17661=ADVANCED_FACE('',(#4545),#322,.T.);
#17678=CLOSED_SHELL('',(#17506,#17507,#17508,#17509,#17510,#17511,#17512,
#17513,#17514,#17515,#17516,#17517,#17518,#17519,#17520,#17521,#17522,#17523,
#17524,#17525,#17526,#17527,#17528,#17529,#17530,#17531,#17532,#17533,#17534,
#17535,#17536,#17537,#17538,#17539,#17540,#17541,#17542,#17543,#17544,#17545,
#17546,#17547,#17548,#17549,#17550,#17551,#17552,#17553,#17554,#17555,#17556,
#17557,#17558,#17559,#17560,#17561,#17562,#17563,#17564,#17565,#17566,#17567,
#17568,#17569,#17570,#17571,#17572,#17573,#17574,#17575,#17576,#17577,#17578,
#17579,#17580,#17581,#17582,#17583,#17584,#17585,#17586,#17587,#17588,#17589,
#17590,#17591,#17592,#17593,#17594,#17595,#17596,#17597,#17598,#17599,#17600,
#17601,#17602,#17603,#17604,#17605,#17606,#17607,#17608,#17609,#17610,#17611,
#17612,#17613,#17614,#17615,#17616,#17617,#17618,#17619,#17620,#17621,#17622,
#17623,#17624,#17625,#17626,#17627,#17628,#17629,#17630,#17631,#17632,#17633,
#17634,#17635,#17636,#17637,#17638,#17639,#17640,#17641,#17642,#17643,#17644,
#17645,#17646,#17647,#17648,#17649,#17650,#17651,#17652,#17653,#17654,#17655,
#17656,#17657,#17658,#17659,#17660,#17661));
#19293=AXIS2_PLACEMENT_3D('',#49131,#23042,#23043);
#19294=AXIS2_PLACEMENT_3D('',#49597,#23044,#23045);
#19295=AXIS2_PLACEMENT_3D('',#49607,#23047,#23048);
#19296=AXIS2_PLACEMENT_3D('',#49611,#23050,#23051);
#19297=AXIS2_PLACEMENT_3D('',#49612,#23052,#23053);
#19298=AXIS2_PLACEMENT_3D('',#49613,#23054,#23055);
#19299=AXIS2_PLACEMENT_3D('',#49615,#23056,#23057);
#19300=AXIS2_PLACEMENT_3D('',#49618,#23059,#23060);
#19301=AXIS2_PLACEMENT_3D('',#49619,#23061,#23062);
#19302=AXIS2_PLACEMENT_3D('',#49622,#23063,#23064);
#19303=AXIS2_PLACEMENT_3D('',#49626,#23066,#23067);
#19304=AXIS2_PLACEMENT_3D('',#49628,#23069,#23070);
#19305=AXIS2_PLACEMENT_3D('',#49633,#23072,#23073);
#19306=AXIS2_PLACEMENT_3D('',#49636,#23075,#23076);
#19307=AXIS2_PLACEMENT_3D('',#49637,#23077,#23078);
#19308=AXIS2_PLACEMENT_3D('',#49640,#23079,#23080);
#19309=AXIS2_PLACEMENT_3D('',#49642,#23081,#23082);
#19310=AXIS2_PLACEMENT_3D('',#49644,#23083,#23084);
#19311=AXIS2_PLACEMENT_3D('',#49646,#23085,#23086);
#19312=AXIS2_PLACEMENT_3D('',#49648,#23087,#23088);
#19313=AXIS2_PLACEMENT_3D('',#49650,#23089,#23090);
#19314=AXIS2_PLACEMENT_3D('',#49652,#23091,#23092);
#19315=AXIS2_PLACEMENT_3D('',#49654,#23093,#23094);
#19316=AXIS2_PLACEMENT_3D('',#49656,#23095,#23096);
#19317=AXIS2_PLACEMENT_3D('',#49657,#23097,#23098);
#19318=AXIS2_PLACEMENT_3D('',#49659,#23099,#23100);
#19319=AXIS2_PLACEMENT_3D('',#49661,#23101,#23102);
#19320=AXIS2_PLACEMENT_3D('',#49663,#23103,#23104);
#19321=AXIS2_PLACEMENT_3D('',#49665,#23105,#23106);
#19322=AXIS2_PLACEMENT_3D('',#49666,#23107,#23108);
#19323=AXIS2_PLACEMENT_3D('',#49677,#23110,#23111);
#19324=AXIS2_PLACEMENT_3D('',#49690,#23113,#23114);
#19325=AXIS2_PLACEMENT_3D('',#49693,#23115,#23116);
#19326=AXIS2_PLACEMENT_3D('',#49697,#23118,#23119);
#19327=AXIS2_PLACEMENT_3D('',#49699,#23121,#23122);
#19328=AXIS2_PLACEMENT_3D('',#49716,#23123,#23124);
#19329=AXIS2_PLACEMENT_3D('',#49718,#23125,#23126);
#19330=AXIS2_PLACEMENT_3D('',#49734,#23127,#23128);
#19331=AXIS2_PLACEMENT_3D('',#49738,#23130,#23131);
#19332=AXIS2_PLACEMENT_3D('',#49739,#23132,#23133);
#19333=AXIS2_PLACEMENT_3D('',#49740,#23134,#23135);
#19334=AXIS2_PLACEMENT_3D('',#49761,#23136,#23137);
#19335=AXIS2_PLACEMENT_3D('',#49766,#23139,#23140);
#19336=AXIS2_PLACEMENT_3D('',#49769,#23142,#23143);
#19337=AXIS2_PLACEMENT_3D('',#49770,#23144,#23145);
#19338=AXIS2_PLACEMENT_3D('',#49776,#23149,#23150);
#19339=AXIS2_PLACEMENT_3D('',#49781,#23152,#23153);
#19340=AXIS2_PLACEMENT_3D('',#49784,#23155,#23156);
#19341=AXIS2_PLACEMENT_3D('',#49785,#23157,#23158);
#19342=AXIS2_PLACEMENT_3D('',#49791,#23162,#23163);
#19343=AXIS2_PLACEMENT_3D('',#49792,#23164,#23165);
#19344=AXIS2_PLACEMENT_3D('',#49793,#23166,#23167);
#19345=AXIS2_PLACEMENT_3D('',#49794,#23168,#23169);
#19346=AXIS2_PLACEMENT_3D('',#49799,#23171,#23172);
#19347=AXIS2_PLACEMENT_3D('',#49805,#23175,#23176);
#19348=AXIS2_PLACEMENT_3D('',#49809,#23178,#23179);
#19349=AXIS2_PLACEMENT_3D('',#49813,#23181,#23182);
#19350=AXIS2_PLACEMENT_3D('',#49816,#23184,#23185);
#19351=AXIS2_PLACEMENT_3D('',#49818,#23186,#23187);
#19352=AXIS2_PLACEMENT_3D('',#49820,#23188,#23189);
#19353=AXIS2_PLACEMENT_3D('',#49821,#23190,#23191);
#19354=AXIS2_PLACEMENT_3D('',#49839,#23193,#23194);
#19355=AXIS2_PLACEMENT_3D('',#49843,#23196,#23197);
#19356=AXIS2_PLACEMENT_3D('',#49847,#23199,#23200);
#19357=AXIS2_PLACEMENT_3D('',#49878,#23202,#23203);
#19358=AXIS2_PLACEMENT_3D('',#49879,#23204,#23205);
#19359=AXIS2_PLACEMENT_3D('',#49880,#23206,#23207);
#19360=AXIS2_PLACEMENT_3D('',#49885,#23209,#23210);
#19361=AXIS2_PLACEMENT_3D('',#49888,#23212,#23213);
#19362=AXIS2_PLACEMENT_3D('',#49889,#23214,#23215);
#19363=AXIS2_PLACEMENT_3D('',#49890,#23216,#23217);
#19364=AXIS2_PLACEMENT_3D('',#49891,#23218,#23219);
#19365=AXIS2_PLACEMENT_3D('',#49892,#23220,#23221);
#19366=AXIS2_PLACEMENT_3D('',#49895,#23222,#23223);
#19367=AXIS2_PLACEMENT_3D('',#49897,#23224,#23225);
#19368=AXIS2_PLACEMENT_3D('',#49899,#23226,#23227);
#19369=AXIS2_PLACEMENT_3D('',#49901,#23228,#23229);
#19370=AXIS2_PLACEMENT_3D('',#49903,#23230,#23231);
#19371=AXIS2_PLACEMENT_3D('',#49905,#23232,#23233);
#19372=AXIS2_PLACEMENT_3D('',#49906,#23234,#23235);
#19373=AXIS2_PLACEMENT_3D('',#49908,#23236,#23237);
#19374=AXIS2_PLACEMENT_3D('',#49910,#23238,#23239);
#19375=AXIS2_PLACEMENT_3D('',#49912,#23240,#23241);
#19376=AXIS2_PLACEMENT_3D('',#49913,#23242,#23243);
#19377=AXIS2_PLACEMENT_3D('',#49914,#23244,#23245);
#19378=AXIS2_PLACEMENT_3D('',#49916,#23246,#23247);
#19379=AXIS2_PLACEMENT_3D('',#49918,#23248,#23249);
#19380=AXIS2_PLACEMENT_3D('',#49919,#23250,#23251);
#19381=AXIS2_PLACEMENT_3D('',#49922,#23252,#23253);
#19382=AXIS2_PLACEMENT_3D('',#49923,#23254,#23255);
#19383=AXIS2_PLACEMENT_3D('',#49927,#23257,#23258);
#19384=AXIS2_PLACEMENT_3D('',#49928,#23259,#23260);
#19385=AXIS2_PLACEMENT_3D('',#49929,#23261,#23262);
#19386=AXIS2_PLACEMENT_3D('',#49988,#23268,#23269);
#19387=AXIS2_PLACEMENT_3D('',#49989,#23270,#23271);
#19388=AXIS2_PLACEMENT_3D('',#50038,#23275,#23276);
#19389=AXIS2_PLACEMENT_3D('',#51349,#23281,#23282);
#19390=AXIS2_PLACEMENT_3D('',#51351,#23283,#23284);
#19391=AXIS2_PLACEMENT_3D('',#51352,#23285,#23286);
#19392=AXIS2_PLACEMENT_3D('',#51357,#23287,#23288);
#19393=AXIS2_PLACEMENT_3D('',#51362,#23289,#23290);
#19394=AXIS2_PLACEMENT_3D('',#51367,#23291,#23292);
#19395=AXIS2_PLACEMENT_3D('',#51372,#23293,#23294);
#19396=AXIS2_PLACEMENT_3D('',#51377,#23295,#23296);
#19397=AXIS2_PLACEMENT_3D('',#51380,#23297,#23298);
#19398=AXIS2_PLACEMENT_3D('',#51384,#23300,#23301);
#19399=AXIS2_PLACEMENT_3D('',#51386,#23303,#23304);
#19400=AXIS2_PLACEMENT_3D('',#51389,#23306,#23307);
#19401=AXIS2_PLACEMENT_3D('',#51390,#23308,#23309);
#19402=AXIS2_PLACEMENT_3D('',#51392,#23310,#23311);
#19403=AXIS2_PLACEMENT_3D('',#51394,#23313,#23314);
#19404=AXIS2_PLACEMENT_3D('',#51533,#23317,#23318);
#19405=AXIS2_PLACEMENT_3D('',#51543,#23321,#23322);
#19406=AXIS2_PLACEMENT_3D('',#51545,#23323,#23324);
#19407=AXIS2_PLACEMENT_3D('',#51547,#23325,#23326);
#19408=AXIS2_PLACEMENT_3D('',#51548,#23327,#23328);
#19409=AXIS2_PLACEMENT_3D('',#51553,#23330,#23331);
#19410=AXIS2_PLACEMENT_3D('',#51556,#23333,#23334);
#19411=AXIS2_PLACEMENT_3D('',#51557,#23335,#23336);
#19412=AXIS2_PLACEMENT_3D('',#51563,#23340,#23341);
#19413=AXIS2_PLACEMENT_3D('',#51723,#23345,#23346);
#19414=AXIS2_PLACEMENT_3D('',#51958,#23347,#23348);
#19415=AXIS2_PLACEMENT_3D('',#52649,#23349,#23350);
#19416=AXIS2_PLACEMENT_3D('',#52691,#23351,#23352);
#19417=AXIS2_PLACEMENT_3D('',#53230,#23353,#23354);
#19418=AXIS2_PLACEMENT_3D('',#53342,#23355,#23356);
#19419=AXIS2_PLACEMENT_3D('',#53450,#23357,#23358);
#19420=AXIS2_PLACEMENT_3D('',#53451,#23359,#23360);
#19421=AXIS2_PLACEMENT_3D('',#53575,#23361,#23362);
#19422=AXIS2_PLACEMENT_3D('',#53576,#23363,#23364);
#19423=AXIS2_PLACEMENT_3D('',#53577,#23365,#23366);
#19424=AXIS2_PLACEMENT_3D('',#53578,#23367,#23368);
#19425=AXIS2_PLACEMENT_3D('',#53579,#23369,#23370);
#19426=AXIS2_PLACEMENT_3D('',#53580,#23371,#23372);
#19427=AXIS2_PLACEMENT_3D('',#53581,#23373,#23374);
#19428=AXIS2_PLACEMENT_3D('',#53582,#23375,#23376);
#19429=AXIS2_PLACEMENT_3D('',#53583,#23377,#23378);
#19430=AXIS2_PLACEMENT_3D('',#53596,#23379,#23380);
#19431=AXIS2_PLACEMENT_3D('',#53597,#23381,#23382);
#19432=AXIS2_PLACEMENT_3D('',#53598,#23383,#23384);
#19433=AXIS2_PLACEMENT_3D('',#53599,#23385,#23386);
#19434=AXIS2_PLACEMENT_3D('',#53600,#23387,#23388);
#19435=AXIS2_PLACEMENT_3D('',#53601,#23389,#23390);
#19436=AXIS2_PLACEMENT_3D('',#53602,#23391,#23392);
#19437=AXIS2_PLACEMENT_3D('',#53603,#23393,#23394);
#19438=AXIS2_PLACEMENT_3D('',#53618,#23395,#23396);
#19439=AXIS2_PLACEMENT_3D('',#53633,#23397,#23398);
#19440=AXIS2_PLACEMENT_3D('',#53634,#23399,#23400);
#19441=AXIS2_PLACEMENT_3D('',#53635,#23401,#23402);
#19442=AXIS2_PLACEMENT_3D('',#53636,#23403,#23404);
#19443=AXIS2_PLACEMENT_3D('',#53637,#23405,#23406);
#19444=AXIS2_PLACEMENT_3D('',#53638,#23407,#23408);
#19445=AXIS2_PLACEMENT_3D('',#53639,#23409,#23410);
#19446=AXIS2_PLACEMENT_3D('',#53640,#23411,#23412);
#19447=AXIS2_PLACEMENT_3D('',#53653,#23413,#23414);
#19448=AXIS2_PLACEMENT_3D('',#53654,#23415,#23416);
#19449=AXIS2_PLACEMENT_3D('',#53655,#23417,#23418);
#19450=AXIS2_PLACEMENT_3D('',#53656,#23419,#23420);
#19451=AXIS2_PLACEMENT_3D('',#53657,#23421,#23422);
#19452=AXIS2_PLACEMENT_3D('',#53658,#23423,#23424);
#19453=AXIS2_PLACEMENT_3D('',#53659,#23425,#23426);
#19454=AXIS2_PLACEMENT_3D('',#53660,#23427,#23428);
#19455=AXIS2_PLACEMENT_3D('',#53680,#23429,#23430);
#19456=AXIS2_PLACEMENT_3D('',#53681,#23431,#23432);
#19457=AXIS2_PLACEMENT_3D('',#53682,#23433,#23434);
#19458=AXIS2_PLACEMENT_3D('',#53683,#23435,#23436);
#19459=AXIS2_PLACEMENT_3D('',#53684,#23437,#23438);
#19460=AXIS2_PLACEMENT_3D('',#53724,#23439,#23440);
#19461=AXIS2_PLACEMENT_3D('',#53725,#23441,#23442);
#19462=AXIS2_PLACEMENT_3D('',#53726,#23443,#23444);
#19463=AXIS2_PLACEMENT_3D('',#53727,#23445,#23446);
#19464=AXIS2_PLACEMENT_3D('',#53728,#23447,#23448);
#19465=AXIS2_PLACEMENT_3D('',#53729,#23449,#23450);
#19466=AXIS2_PLACEMENT_3D('',#53730,#23451,#23452);
#19467=AXIS2_PLACEMENT_3D('',#53731,#23453,#23454);
#19468=AXIS2_PLACEMENT_3D('',#53732,#23455,#23456);
#19469=AXIS2_PLACEMENT_3D('',#53733,#23457,#23458);
#19470=AXIS2_PLACEMENT_3D('',#53749,#23459,#23460);
#19471=AXIS2_PLACEMENT_3D('',#53750,#23461,#23462);
#19472=AXIS2_PLACEMENT_3D('',#53751,#23463,#23464);
#19473=AXIS2_PLACEMENT_3D('',#53752,#23465,#23466);
#19474=AXIS2_PLACEMENT_3D('',#53753,#23467,#23468);
#19475=AXIS2_PLACEMENT_3D('',#53754,#23469,#23470);
#19476=AXIS2_PLACEMENT_3D('',#53755,#23471,#23472);
#19477=AXIS2_PLACEMENT_3D('',#53756,#23473,#23474);
#19478=AXIS2_PLACEMENT_3D('',#53757,#23475,#23476);
#19479=AXIS2_PLACEMENT_3D('',#53758,#23477,#23478);
#19480=AXIS2_PLACEMENT_3D('',#53759,#23479,#23480);
#19481=AXIS2_PLACEMENT_3D('',#53760,#23481,#23482);
#19482=AXIS2_PLACEMENT_3D('',#53761,#23483,#23484);
#19483=AXIS2_PLACEMENT_3D('',#53762,#23485,#23486);
#19484=AXIS2_PLACEMENT_3D('',#53763,#23487,#23488);
#19485=AXIS2_PLACEMENT_3D('',#53764,#23489,#23490);
#19486=AXIS2_PLACEMENT_3D('',#53765,#23491,#23492);
#19487=AXIS2_PLACEMENT_3D('',#53785,#23493,#23494);
#19488=AXIS2_PLACEMENT_3D('',#53786,#23495,#23496);
#19489=AXIS2_PLACEMENT_3D('',#53787,#23497,#23498);
#19490=AXIS2_PLACEMENT_3D('',#53788,#23499,#23500);
#19491=AXIS2_PLACEMENT_3D('',#53789,#23501,#23502);
#19492=AXIS2_PLACEMENT_3D('',#53790,#23503,#23504);
#19493=AXIS2_PLACEMENT_3D('',#53791,#23505,#23506);
#19494=AXIS2_PLACEMENT_3D('',#53831,#23507,#23508);
#19495=AXIS2_PLACEMENT_3D('',#53832,#23509,#23510);
#19496=AXIS2_PLACEMENT_3D('',#53833,#23511,#23512);
#19497=AXIS2_PLACEMENT_3D('',#53834,#23513,#23514);
#19498=AXIS2_PLACEMENT_3D('',#53835,#23515,#23516);
#19499=AXIS2_PLACEMENT_3D('',#53851,#23517,#23518);
#19500=AXIS2_PLACEMENT_3D('',#53852,#23519,#23520);
#19501=AXIS2_PLACEMENT_3D('',#53853,#23521,#23522);
#19502=AXIS2_PLACEMENT_3D('',#53854,#23523,#23524);
#19503=AXIS2_PLACEMENT_3D('',#53855,#23525,#23526);
#19504=AXIS2_PLACEMENT_3D('',#53856,#23527,#23528);
#19505=AXIS2_PLACEMENT_3D('',#53857,#23529,#23530);
#19506=AXIS2_PLACEMENT_3D('',#53858,#23531,#23532);
#19507=AXIS2_PLACEMENT_3D('',#53859,#23533,#23534);
#19508=AXIS2_PLACEMENT_3D('',#53879,#23535,#23536);
#19509=AXIS2_PLACEMENT_3D('',#53880,#23537,#23538);
#19510=AXIS2_PLACEMENT_3D('',#53929,#23539,#23540);
#19511=AXIS2_PLACEMENT_3D('',#53945,#23541,#23542);
#19512=AXIS2_PLACEMENT_3D('',#53946,#23543,#23544);
#19513=AXIS2_PLACEMENT_3D('',#53947,#23545,#23546);
#19514=AXIS2_PLACEMENT_3D('',#53948,#23547,#23548);
#19515=AXIS2_PLACEMENT_3D('',#53949,#23549,#23550);
#19516=AXIS2_PLACEMENT_3D('',#53950,#23551,#23552);
#19517=AXIS2_PLACEMENT_3D('',#53951,#23553,#23554);
#19518=AXIS2_PLACEMENT_3D('',#53967,#23555,#23556);
#19519=AXIS2_PLACEMENT_3D('',#53968,#23557,#23558);
#19520=AXIS2_PLACEMENT_3D('',#53969,#23559,#23560);
#19521=AXIS2_PLACEMENT_3D('',#53989,#23561,#23562);
#19522=AXIS2_PLACEMENT_3D('',#53990,#23563,#23564);
#19523=AXIS2_PLACEMENT_3D('',#53991,#23565,#23566);
#19524=AXIS2_PLACEMENT_3D('',#54031,#23567,#23568);
#19525=AXIS2_PLACEMENT_3D('',#54032,#23569,#23570);
#19526=AXIS2_PLACEMENT_3D('',#54033,#23571,#23572);
#19527=AXIS2_PLACEMENT_3D('',#54062,#23573,#23574);
#19528=AXIS2_PLACEMENT_3D('',#54063,#23575,#23576);
#19529=AXIS2_PLACEMENT_3D('',#54064,#23577,#23578);
#19530=AXIS2_PLACEMENT_3D('',#54065,#23579,#23580);
#19531=AXIS2_PLACEMENT_3D('',#54066,#23581,#23582);
#19532=AXIS2_PLACEMENT_3D('',#54067,#23583,#23584);
#19533=AXIS2_PLACEMENT_3D('',#54068,#23585,#23586);
#19534=AXIS2_PLACEMENT_3D('',#54069,#23587,#23588);
#19535=AXIS2_PLACEMENT_3D('',#54070,#23589,#23590);
#19536=AXIS2_PLACEMENT_3D('',#54071,#23591,#23592);
#19537=AXIS2_PLACEMENT_3D('',#54072,#23593,#23594);
#19538=AXIS2_PLACEMENT_3D('',#54073,#23595,#23596);
#19539=AXIS2_PLACEMENT_3D('',#54074,#23597,#23598);
#19540=AXIS2_PLACEMENT_3D('',#54075,#23599,#23600);
#19541=AXIS2_PLACEMENT_3D('',#54076,#23601,#23602);
#19542=AXIS2_PLACEMENT_3D('',#54077,#23603,#23604);
#19543=AXIS2_PLACEMENT_3D('',#54078,#23605,#23606);
#19544=AXIS2_PLACEMENT_3D('',#54110,#23607,#23608);
#19545=AXIS2_PLACEMENT_3D('',#54133,#23609,#23610);
#19546=AXIS2_PLACEMENT_3D('',#54134,#23611,#23612);
#19547=AXIS2_PLACEMENT_3D('',#54300,#23613,#23614);
#19548=AXIS2_PLACEMENT_3D('',#54301,#23615,#23616);
#19549=AXIS2_PLACEMENT_3D('',#54326,#23617,#23618);
#19550=AXIS2_PLACEMENT_3D('',#54348,#23619,#23620);
#19551=AXIS2_PLACEMENT_3D('',#54349,#23621,#23622);
#19552=AXIS2_PLACEMENT_3D('',#54350,#23623,#23624);
#19553=AXIS2_PLACEMENT_3D('',#54351,#23625,#23626);
#19554=AXIS2_PLACEMENT_3D('',#54352,#23627,#23628);
#19555=AXIS2_PLACEMENT_3D('',#54377,#23629,#23630);
#19556=AXIS2_PLACEMENT_3D('',#54402,#23631,#23632);
#19557=AXIS2_PLACEMENT_3D('',#54403,#23633,#23634);
#19558=AXIS2_PLACEMENT_3D('',#54404,#23635,#23636);
#19559=AXIS2_PLACEMENT_3D('',#54405,#23637,#23638);
#19560=AXIS2_PLACEMENT_3D('',#54430,#23639,#23640);
#19561=AXIS2_PLACEMENT_3D('',#54455,#23641,#23642);
#19562=AXIS2_PLACEMENT_3D('',#54456,#23643,#23644);
#19563=AXIS2_PLACEMENT_3D('',#54457,#23645,#23646);
#19564=AXIS2_PLACEMENT_3D('',#54458,#23647,#23648);
#19565=AXIS2_PLACEMENT_3D('',#54459,#23649,#23650);
#19566=AXIS2_PLACEMENT_3D('',#54460,#23651,#23652);
#19567=AXIS2_PLACEMENT_3D('',#54461,#23653,#23654);
#19568=AXIS2_PLACEMENT_3D('',#54483,#23655,#23656);
#19569=AXIS2_PLACEMENT_3D('',#54508,#23657,#23658);
#19570=AXIS2_PLACEMENT_3D('',#54509,#23659,#23660);
#19571=AXIS2_PLACEMENT_3D('',#54510,#23661,#23662);
#19572=AXIS2_PLACEMENT_3D('',#54512,#23664,#23665);
#19573=AXIS2_PLACEMENT_3D('',#54514,#23667,#23668);
#19574=AXIS2_PLACEMENT_3D('',#54516,#23670,#23671);
#19575=AXIS2_PLACEMENT_3D('',#54518,#23673,#23674);
#19576=AXIS2_PLACEMENT_3D('',#54519,#23675,#23676);
#23042=DIRECTION('axis',(0.,0.,1.));
#23043=DIRECTION('refdir',(1.,0.,0.));
#23044=DIRECTION('center_axis',(0.,-1.,0.));
#23045=DIRECTION('ref_axis',(0.999832864782553,0.,-0.0182823002030212));
#23046=DIRECTION('',(0.,-1.,0.));
#23047=DIRECTION('center_axis',(0.,1.,0.));
#23048=DIRECTION('ref_axis',(0.,0.,1.));
#23049=DIRECTION('',(0.,-1.,0.));
#23050=DIRECTION('center_axis',(0.,1.,0.));
#23051=DIRECTION('ref_axis',(0.,0.,1.));
#23052=DIRECTION('center_axis',(0.,1.,0.));
#23053=DIRECTION('ref_axis',(0.,0.,1.));
#23054=DIRECTION('center_axis',(0.,1.,0.));
#23055=DIRECTION('ref_axis',(0.,0.,1.));
#23056=DIRECTION('center_axis',(0.,1.,0.));
#23057=DIRECTION('ref_axis',(0.,0.,1.));
#23058=DIRECTION('',(0.,1.,0.));
#23059=DIRECTION('center_axis',(0.,1.,0.));
#23060=DIRECTION('ref_axis',(0.,0.,1.));
#23061=DIRECTION('center_axis',(0.,1.,0.));
#23062=DIRECTION('ref_axis',(0.,0.,1.));
#23063=DIRECTION('center_axis',(0.,1.,0.));
#23064=DIRECTION('ref_axis',(0.,0.,1.));
#23065=DIRECTION('',(0.,1.,0.));
#23066=DIRECTION('center_axis',(0.,1.,0.));
#23067=DIRECTION('ref_axis',(0.,0.,1.));
#23068=DIRECTION('',(0.,1.,0.));
#23069=DIRECTION('center_axis',(0.,1.,0.));
#23070=DIRECTION('ref_axis',(0.,0.,1.));
#23071=DIRECTION('',(0.,-1.,0.));
#23072=DIRECTION('center_axis',(0.,1.,0.));
#23073=DIRECTION('ref_axis',(0.,0.,1.));
#23074=DIRECTION('',(0.,-1.,0.));
#23075=DIRECTION('center_axis',(0.,1.,0.));
#23076=DIRECTION('ref_axis',(0.,0.,1.));
#23077=DIRECTION('center_axis',(0.,1.,0.));
#23078=DIRECTION('ref_axis',(0.,0.,1.));
#23079=DIRECTION('center_axis',(0.,1.,0.));
#23080=DIRECTION('ref_axis',(0.,0.,1.));
#23081=DIRECTION('center_axis',(0.,1.,0.));
#23082=DIRECTION('ref_axis',(0.,0.,1.));
#23083=DIRECTION('center_axis',(0.,1.,0.));
#23084=DIRECTION('ref_axis',(0.,0.,1.));
#23085=DIRECTION('center_axis',(0.,1.,0.));
#23086=DIRECTION('ref_axis',(0.,0.,1.));
#23087=DIRECTION('center_axis',(0.,1.,0.));
#23088=DIRECTION('ref_axis',(0.,0.,1.));
#23089=DIRECTION('center_axis',(0.,1.,0.));
#23090=DIRECTION('ref_axis',(0.,0.,1.));
#23091=DIRECTION('center_axis',(0.,1.,0.));
#23092=DIRECTION('ref_axis',(0.,0.,1.));
#23093=DIRECTION('center_axis',(0.,1.,0.));
#23094=DIRECTION('ref_axis',(0.,0.,1.));
#23095=DIRECTION('center_axis',(0.,1.,0.));
#23096=DIRECTION('ref_axis',(0.,0.,1.));
#23097=DIRECTION('center_axis',(0.,1.,0.));
#23098=DIRECTION('ref_axis',(0.,0.,1.));
#23099=DIRECTION('center_axis',(0.,1.,0.));
#23100=DIRECTION('ref_axis',(0.,0.,1.));
#23101=DIRECTION('center_axis',(0.,1.,0.));
#23102=DIRECTION('ref_axis',(0.,0.,1.));
#23103=DIRECTION('center_axis',(0.,1.,0.));
#23104=DIRECTION('ref_axis',(0.,0.,1.));
#23105=DIRECTION('center_axis',(0.,1.,0.));
#23106=DIRECTION('ref_axis',(0.,0.,1.));
#23107=DIRECTION('center_axis',(0.,-1.,0.));
#23108=DIRECTION('ref_axis',(0.240266771391976,0.,0.970706896320859));
#23109=DIRECTION('',(0.,-1.,0.));
#23110=DIRECTION('center_axis',(0.,1.,0.));
#23111=DIRECTION('ref_axis',(0.,0.,1.));
#23112=DIRECTION('',(0.,-1.,0.));
#23113=DIRECTION('center_axis',(0.,-1.,0.));
#23114=DIRECTION('ref_axis',(0.,0.,-1.));
#23115=DIRECTION('center_axis',(0.,1.,0.));
#23116=DIRECTION('ref_axis',(0.,0.,1.));
#23117=DIRECTION('',(0.,-1.,0.));
#23118=DIRECTION('center_axis',(0.,1.,0.));
#23119=DIRECTION('ref_axis',(0.,0.,1.));
#23120=DIRECTION('',(0.,-1.,0.));
#23121=DIRECTION('center_axis',(1.,0.,0.));
#23122=DIRECTION('ref_axis',(0.,0.,-1.));
#23123=DIRECTION('center_axis',(-1.,0.,0.));
#23124=DIRECTION('ref_axis',(0.,-1.55431223447522E-15,-1.));
#23125=DIRECTION('center_axis',(-1.,0.,0.));
#23126=DIRECTION('ref_axis',(0.,-0.493494070811408,-0.869749160433044));
#23127=DIRECTION('center_axis',(1.,0.,0.));
#23128=DIRECTION('ref_axis',(0.,0.,-1.));
#23129=DIRECTION('',(-1.,0.,0.));
#23130=DIRECTION('center_axis',(-1.,0.,0.));
#23131=DIRECTION('ref_axis',(0.,0.,1.));
#23132=DIRECTION('center_axis',(-1.,0.,0.));
#23133=DIRECTION('ref_axis',(0.,0.,1.));
#23134=DIRECTION('center_axis',(1.,0.,0.));
#23135=DIRECTION('ref_axis',(0.,0.,-1.));
#23136=DIRECTION('center_axis',(0.,-1.,0.));
#23137=DIRECTION('ref_axis',(0.,0.,-1.));
#23138=DIRECTION('',(0.,-1.,0.));
#23139=DIRECTION('center_axis',(0.,1.,0.));
#23140=DIRECTION('ref_axis',(0.,0.,1.));
#23141=DIRECTION('',(0.,-1.,0.));
#23142=DIRECTION('center_axis',(0.,1.,0.));
#23143=DIRECTION('ref_axis',(0.,0.,1.));
#23144=DIRECTION('center_axis',(-2.77555756156289E-16,0.,-1.));
#23145=DIRECTION('ref_axis',(-1.,0.,2.77555756156289E-16));
#23146=DIRECTION('',(0.,-1.,0.));
#23147=DIRECTION('',(1.,0.,-2.77555756156289E-16));
#23148=DIRECTION('',(1.,0.,-2.77555756156289E-16));
#23149=DIRECTION('center_axis',(0.,-1.,0.));
#23150=DIRECTION('ref_axis',(0.,0.,-1.));
#23151=DIRECTION('',(0.,-1.,0.));
#23152=DIRECTION('center_axis',(0.,1.,0.));
#23153=DIRECTION('ref_axis',(0.,0.,1.));
#23154=DIRECTION('',(0.,-1.,0.));
#23155=DIRECTION('center_axis',(0.,1.,0.));
#23156=DIRECTION('ref_axis',(0.,0.,1.));
#23157=DIRECTION('center_axis',(-2.77555756156289E-16,0.,-1.));
#23158=DIRECTION('ref_axis',(-1.,0.,2.77555756156289E-16));
#23159=DIRECTION('',(1.,0.,-2.77555756156289E-16));
#23160=DIRECTION('',(0.,-1.,0.));
#23161=DIRECTION('',(1.,0.,-2.77555756156289E-16));
#23162=DIRECTION('center_axis',(0.,-1.,0.));
#23163=DIRECTION('ref_axis',(0.,0.,-1.));
#23164=DIRECTION('center_axis',(0.,1.,0.));
#23165=DIRECTION('ref_axis',(0.,0.,1.));
#23166=DIRECTION('center_axis',(0.,1.,0.));
#23167=DIRECTION('ref_axis',(0.,0.,1.));
#23168=DIRECTION('center_axis',(0.,1.,0.));
#23169=DIRECTION('ref_axis',(0.,0.,1.));
#23170=DIRECTION('',(-0.885876528532327,0.,-0.463921088328083));
#23171=DIRECTION('center_axis',(0.,1.,0.));
#23172=DIRECTION('ref_axis',(0.,0.,1.));
#23173=DIRECTION('',(0.885876528532327,0.,-0.463921088328083));
#23174=DIRECTION('',(0.860841979634012,0.,0.508872367200063));
#23175=DIRECTION('center_axis',(0.,1.,0.));
#23176=DIRECTION('ref_axis',(0.,0.,1.));
#23177=DIRECTION('',(1.,0.,-2.77555756156289E-16));
#23178=DIRECTION('center_axis',(0.,1.,0.));
#23179=DIRECTION('ref_axis',(0.,0.,1.));
#23180=DIRECTION('',(1.,0.,-2.77555756156289E-16));
#23181=DIRECTION('center_axis',(0.,1.,0.));
#23182=DIRECTION('ref_axis',(0.,0.,1.));
#23183=DIRECTION('',(-0.860841979634012,0.,0.508872367200063));
#23184=DIRECTION('center_axis',(0.,1.,0.));
#23185=DIRECTION('ref_axis',(0.,0.,1.));
#23186=DIRECTION('center_axis',(0.,1.,0.));
#23187=DIRECTION('ref_axis',(0.,0.,1.));
#23188=DIRECTION('center_axis',(0.,1.,0.));
#23189=DIRECTION('ref_axis',(0.,0.,1.));
#23190=DIRECTION('center_axis',(0.,1.,0.));
#23191=DIRECTION('ref_axis',(0.,0.,1.));
#23192=DIRECTION('',(-0.860841979634012,0.,0.508872367200063));
#23193=DIRECTION('center_axis',(0.,1.,0.));
#23194=DIRECTION('ref_axis',(0.,0.,1.));
#23195=DIRECTION('',(1.,0.,-2.77555756156289E-16));
#23196=DIRECTION('center_axis',(0.,1.,0.));
#23197=DIRECTION('ref_axis',(0.,0.,1.));
#23198=DIRECTION('',(1.,0.,-2.77555756156289E-16));
#23199=DIRECTION('center_axis',(0.,1.,0.));
#23200=DIRECTION('ref_axis',(0.,0.,1.));
#23201=DIRECTION('',(0.860841979634012,0.,0.508872367200063));
#23202=DIRECTION('center_axis',(0.,1.,0.));
#23203=DIRECTION('ref_axis',(0.,0.,1.));
#23204=DIRECTION('center_axis',(0.,1.,0.));
#23205=DIRECTION('ref_axis',(0.,0.,1.));
#23206=DIRECTION('center_axis',(0.,-1.,0.));
#23207=DIRECTION('ref_axis',(-1.,0.,1.83697019872103E-16));
#23208=DIRECTION('',(0.,-1.,0.));
#23209=DIRECTION('center_axis',(0.,1.,0.));
#23210=DIRECTION('ref_axis',(0.,0.,1.));
#23211=DIRECTION('',(0.,-1.,0.));
#23212=DIRECTION('center_axis',(0.,1.,0.));
#23213=DIRECTION('ref_axis',(0.,0.,1.));
#23214=DIRECTION('center_axis',(0.,-1.,0.));
#23215=DIRECTION('ref_axis',(1.,0.,-5.0532154980743E-16));
#23216=DIRECTION('center_axis',(0.,1.,0.));
#23217=DIRECTION('ref_axis',(0.,0.,1.));
#23218=DIRECTION('center_axis',(0.,1.,0.));
#23219=DIRECTION('ref_axis',(0.,0.,1.));
#23220=DIRECTION('center_axis',(0.,1.,0.));
#23221=DIRECTION('ref_axis',(0.,0.,1.));
#23222=DIRECTION('center_axis',(0.,1.,0.));
#23223=DIRECTION('ref_axis',(0.,0.,1.));
#23224=DIRECTION('center_axis',(0.,1.,0.));
#23225=DIRECTION('ref_axis',(0.,0.,1.));
#23226=DIRECTION('center_axis',(0.,1.,0.));
#23227=DIRECTION('ref_axis',(0.,0.,1.));
#23228=DIRECTION('center_axis',(0.,1.,0.));
#23229=DIRECTION('ref_axis',(0.,0.,1.));
#23230=DIRECTION('center_axis',(0.,1.,0.));
#23231=DIRECTION('ref_axis',(0.,0.,1.));
#23232=DIRECTION('center_axis',(0.,1.,0.));
#23233=DIRECTION('ref_axis',(0.,0.,1.));
#23234=DIRECTION('center_axis',(0.,-1.,0.));
#23235=DIRECTION('ref_axis',(0.,0.,1.));
#23236=DIRECTION('center_axis',(0.,-1.,0.));
#23237=DIRECTION('ref_axis',(0.,0.,-1.));
#23238=DIRECTION('center_axis',(0.,1.,0.));
#23239=DIRECTION('ref_axis',(0.,0.,1.));
#23240=DIRECTION('center_axis',(0.,1.,0.));
#23241=DIRECTION('ref_axis',(0.,0.,1.));
#23242=DIRECTION('center_axis',(0.,1.,0.));
#23243=DIRECTION('ref_axis',(0.,0.,1.));
#23244=DIRECTION('center_axis',(0.,1.,0.));
#23245=DIRECTION('ref_axis',(0.,0.,1.));
#23246=DIRECTION('center_axis',(0.,1.,0.));
#23247=DIRECTION('ref_axis',(0.,0.,1.));
#23248=DIRECTION('center_axis',(0.,1.,0.));
#23249=DIRECTION('ref_axis',(0.,0.,1.));
#23250=DIRECTION('center_axis',(0.,-1.,0.));
#23251=DIRECTION('ref_axis',(0.,0.,-1.));
#23252=DIRECTION('center_axis',(0.,1.,0.));
#23253=DIRECTION('ref_axis',(0.,0.,1.));
#23254=DIRECTION('center_axis',(0.,1.,0.));
#23255=DIRECTION('ref_axis',(0.,0.,1.));
#23256=DIRECTION('',(0.,-1.,0.));
#23257=DIRECTION('center_axis',(0.,1.,0.));
#23258=DIRECTION('ref_axis',(0.,0.,1.));
#23259=DIRECTION('center_axis',(0.,1.,0.));
#23260=DIRECTION('ref_axis',(0.,0.,1.));
#23261=DIRECTION('center_axis',(0.508872367200063,0.,-0.860841979634012));
#23262=DIRECTION('ref_axis',(-0.860841979634012,0.,-0.508872367200063));
#23263=DIRECTION('',(0.860841979634012,0.,0.508872367200063));
#23264=DIRECTION('',(-0.00269325522461897,-0.999995099755979,-0.00159588230306779));
#23265=DIRECTION('',(0.860841979634012,0.,0.508872367200063));
#23266=DIRECTION('',(0.860841979634012,0.,0.508872367200063));
#23267=DIRECTION('',(0.,1.,0.));
#23268=DIRECTION('center_axis',(0.508872367200063,0.,-0.860841979634012));
#23269=DIRECTION('ref_axis',(-0.860841979634012,0.,-0.508872367200063));
#23270=DIRECTION('center_axis',(0.508872367200063,0.,0.860841979634012));
#23271=DIRECTION('ref_axis',(0.860841979634012,0.,-0.508872367200063));
#23272=DIRECTION('',(-0.860841979634012,0.,0.508872367200063));
#23273=DIRECTION('',(-0.0188132396443243,0.999761206246989,0.0111172162725081));
#23274=DIRECTION('',(-0.860841979634012,0.,0.508872367200063));
#23275=DIRECTION('center_axis',(0.508872367200063,0.,0.860841979634012));
#23276=DIRECTION('ref_axis',(0.860841979634012,0.,-0.508872367200063));
#23277=DIRECTION('',(0.,1.,0.));
#23278=DIRECTION('',(-0.860841979634012,0.,0.508872367200063));
#23279=DIRECTION('',(-0.0248338283987128,0.999591512051479,0.0141453173064702));
#23280=DIRECTION('',(0.003001304709461,-0.999994675620979,0.0012809760867381));
#23281=DIRECTION('center_axis',(-1.,0.,0.));
#23282=DIRECTION('ref_axis',(0.,0.,1.));
#23283=DIRECTION('center_axis',(-1.,0.,0.));
#23284=DIRECTION('ref_axis',(0.,0.,1.));
#23285=DIRECTION('center_axis',(0.,0.,-1.));
#23286=DIRECTION('ref_axis',(1.,0.,0.));
#23287=DIRECTION('center_axis',(0.,0.,-1.));
#23288=DIRECTION('ref_axis',(1.,0.,0.));
#23289=DIRECTION('center_axis',(0.,0.,-1.));
#23290=DIRECTION('ref_axis',(1.,0.,0.));
#23291=DIRECTION('center_axis',(0.,0.,-1.));
#23292=DIRECTION('ref_axis',(1.,0.,0.));
#23293=DIRECTION('center_axis',(0.,0.,-1.));
#23294=DIRECTION('ref_axis',(1.,0.,0.));
#23295=DIRECTION('center_axis',(0.,1.,0.));
#23296=DIRECTION('ref_axis',(0.,0.,1.));
#23297=DIRECTION('center_axis',(0.,1.,0.));
#23298=DIRECTION('ref_axis',(0.,0.,1.));
#23299=DIRECTION('',(0.,1.,0.));
#23300=DIRECTION('center_axis',(0.,1.,0.));
#23301=DIRECTION('ref_axis',(0.,0.,1.));
#23302=DIRECTION('',(0.,1.,0.));
#23303=DIRECTION('center_axis',(0.,-1.,0.));
#23304=DIRECTION('ref_axis',(-0.988127879018848,0.,-0.153633637936853));
#23305=DIRECTION('',(0.,-1.,0.));
#23306=DIRECTION('center_axis',(0.,1.,0.));
#23307=DIRECTION('ref_axis',(0.,0.,1.));
#23308=DIRECTION('center_axis',(0.,-1.,0.));
#23309=DIRECTION('ref_axis',(-0.988127879018849,0.,0.153633637936853));
#23310=DIRECTION('center_axis',(0.,1.,0.));
#23311=DIRECTION('ref_axis',(0.,0.,1.));
#23312=DIRECTION('',(0.,-1.,0.));
#23313=DIRECTION('center_axis',(0.,1.,0.));
#23314=DIRECTION('ref_axis',(0.,0.,1.));
#23315=DIRECTION('',(0.860841979634012,0.,0.508872367200063));
#23316=DIRECTION('',(-0.885876528532327,0.,0.463921088328083));
#23317=DIRECTION('center_axis',(0.,1.,0.));
#23318=DIRECTION('ref_axis',(0.,0.,1.));
#23319=DIRECTION('',(0.885876528532327,0.,0.463921088328083));
#23320=DIRECTION('',(-0.860841979634012,0.,0.508872367200063));
#23321=DIRECTION('center_axis',(0.,1.,0.));
#23322=DIRECTION('ref_axis',(0.,0.,1.));
#23323=DIRECTION('center_axis',(0.,1.,0.));
#23324=DIRECTION('ref_axis',(0.,0.,1.));
#23325=DIRECTION('center_axis',(0.,1.,0.));
#23326=DIRECTION('ref_axis',(0.,0.,1.));
#23327=DIRECTION('center_axis',(0.,1.,0.));
#23328=DIRECTION('ref_axis',(0.,0.,1.));
#23329=DIRECTION('',(0.,1.,0.));
#23330=DIRECTION('center_axis',(0.,1.,0.));
#23331=DIRECTION('ref_axis',(0.,0.,1.));
#23332=DIRECTION('',(0.,1.,0.));
#23333=DIRECTION('center_axis',(0.,1.,0.));
#23334=DIRECTION('ref_axis',(0.,0.,1.));
#23335=DIRECTION('center_axis',(0.463921088328083,0.,0.885876528532327));
#23336=DIRECTION('ref_axis',(0.885876528532327,0.,-0.463921088328083));
#23337=DIRECTION('',(0.,1.,0.));
#23338=DIRECTION('',(0.885876528532327,0.,-0.463921088328083));
#23339=DIRECTION('',(-0.885876528532327,0.,0.463921088328083));
#23340=DIRECTION('center_axis',(0.463921088328083,0.,-0.885876528532327));
#23341=DIRECTION('ref_axis',(-0.885876528532327,0.,-0.463921088328083));
#23342=DIRECTION('',(-0.885876528532327,0.,-0.463921088328083));
#23343=DIRECTION('',(0.,1.,0.));
#23344=DIRECTION('',(0.885876528532327,0.,0.463921088328083));
#23345=DIRECTION('center_axis',(-0.509699705555825,-0.478496577218806,-0.715015549303784));
#23346=DIRECTION('ref_axis',(-0.814285578254856,1.53671303241302E-16,0.580464466652485));
#23347=DIRECTION('center_axis',(0.510097528065447,0.478091211432643,-0.715003010771556));
#23348=DIRECTION('ref_axis',(-0.814066621565784,2.26446044253015E-17,-0.580771500378996));
#23349=DIRECTION('center_axis',(-0.377407413767257,0.379597766708892,-0.844671048126507));
#23350=DIRECTION('ref_axis',(2.42466011867008E-16,0.912125144520788,0.409911845075172));
#23351=DIRECTION('center_axis',(-0.376533159226498,0.380305963034329,0.844742655773606));
#23352=DIRECTION('ref_axis',(-3.15051401839995E-16,-0.911852106514195,0.410518861741607));
#23353=DIRECTION('center_axis',(0.993761383166,0.0477842249653497,-0.100771926509617));
#23354=DIRECTION('ref_axis',(-0.100887171794749,0.,-0.99489787343589));
#23355=DIRECTION('center_axis',(0.997000202168049,-0.0364823216717374,-0.06826153442686));
#23356=DIRECTION('ref_axis',(-0.0683070065019442,0.,-0.997664348798103));
#23357=DIRECTION('center_axis',(0.997510682482232,-0.0331317236572203,0.0622473069404123));
#23358=DIRECTION('ref_axis',(0.0622814998737367,0.,-0.998058622914244));
#23359=DIRECTION('center_axis',(0.993950716469454,0.0467448536050328,0.0993825532540959));
#23360=DIRECTION('ref_axis',(0.0994913110012255,0.,-0.99503843093383));
#23361=DIRECTION('center_axis',(0.,1.,0.));
#23362=DIRECTION('ref_axis',(0.240266771391976,0.,-0.97070689632086));
#23363=DIRECTION('center_axis',(-0.87052398911462,0.,-0.492125984251968));
#23364=DIRECTION('ref_axis',(-0.492125984251968,0.,0.87052398911462));
#23365=DIRECTION('center_axis',(-0.99957228042324,0.,0.0292447637959857));
#23366=DIRECTION('ref_axis',(0.0292447637959857,0.,0.99957228042324));
#23367=DIRECTION('center_axis',(0.,1.,0.));
#23368=DIRECTION('ref_axis',(0.,0.,1.));
#23369=DIRECTION('center_axis',(0.,1.,0.));
#23370=DIRECTION('ref_axis',(0.,0.,1.));
#23371=DIRECTION('center_axis',(0.943400802255207,0.,-0.331654830063173));
#23372=DIRECTION('ref_axis',(-0.331654830063173,0.,-0.943400802255207));
#23373=DIRECTION('center_axis',(0.,-1.,0.));
#23374=DIRECTION('ref_axis',(0.,0.,-1.));
#23375=DIRECTION('center_axis',(0.,-1.,0.));
#23376=DIRECTION('ref_axis',(0.,0.,-1.));
#23377=DIRECTION('center_axis',(0.,1.,0.));
#23378=DIRECTION('ref_axis',(0.,0.,1.));
#23379=DIRECTION('center_axis',(0.,1.,0.));
#23380=DIRECTION('ref_axis',(0.,0.,1.));
#23381=DIRECTION('center_axis',(-0.943400802255207,0.,0.331654830063173));
#23382=DIRECTION('ref_axis',(0.331654830063173,0.,0.943400802255207));
#23383=DIRECTION('center_axis',(0.341538277837768,0.,-0.939867865591548));
#23384=DIRECTION('ref_axis',(-0.939867865591548,0.,-0.341538277837768));
#23385=DIRECTION('center_axis',(0.,-1.,0.));
#23386=DIRECTION('ref_axis',(0.41535894332624,0.,0.909657599428988));
#23387=DIRECTION('center_axis',(0.,1.,0.));
#23388=DIRECTION('ref_axis',(0.,0.,1.));
#23389=DIRECTION('center_axis',(0.,1.,0.));
#23390=DIRECTION('ref_axis',(0.,0.,1.));
#23391=DIRECTION('center_axis',(-0.933920684244367,0.,-0.357480286925774));
#23392=DIRECTION('ref_axis',(-0.357480286925774,0.,0.933920684244367));
#23393=DIRECTION('center_axis',(0.,1.,0.));
#23394=DIRECTION('ref_axis',(-0.998212936683536,0.,-0.0597572843896898));
#23395=DIRECTION('center_axis',(0.,1.,0.));
#23396=DIRECTION('ref_axis',(0.,0.,1.));
#23397=DIRECTION('center_axis',(0.,1.,0.));
#23398=DIRECTION('ref_axis',(-0.998212936683537,0.,0.0597572843896886));
#23399=DIRECTION('center_axis',(-0.933920684244367,0.,0.357480286925774));
#23400=DIRECTION('ref_axis',(0.357480286925774,0.,0.933920684244367));
#23401=DIRECTION('center_axis',(0.,1.,0.));
#23402=DIRECTION('ref_axis',(0.41535894332623,0.,-0.909657599428993));
#23403=DIRECTION('center_axis',(0.341538277837768,0.,0.939867865591548));
#23404=DIRECTION('ref_axis',(0.939867865591548,0.,-0.341538277837768));
#23405=DIRECTION('center_axis',(0.,1.,0.));
#23406=DIRECTION('ref_axis',(0.,0.,1.));
#23407=DIRECTION('center_axis',(0.,1.,0.));
#23408=DIRECTION('ref_axis',(0.,0.,1.));
#23409=DIRECTION('center_axis',(0.664990346018686,-0.709768435883733,0.232414730869427));
#23410=DIRECTION('ref_axis',(0.667995465406688,0.704421904797486,0.239941322488609));
#23411=DIRECTION('center_axis',(0.,1.,0.));
#23412=DIRECTION('ref_axis',(0.415358943326241,0.,-0.909657599428988));
#23413=DIRECTION('center_axis',(0.,-1.,0.));
#23414=DIRECTION('ref_axis',(0.,0.,-1.));
#23415=DIRECTION('center_axis',(0.,1.,0.));
#23416=DIRECTION('ref_axis',(0.,0.,1.));
#23417=DIRECTION('center_axis',(0.,1.,0.));
#23418=DIRECTION('ref_axis',(0.,0.,1.));
#23419=DIRECTION('center_axis',(0.943400802255207,0.,0.331654830063173));
#23420=DIRECTION('ref_axis',(0.331654830063173,0.,-0.943400802255207));
#23421=DIRECTION('center_axis',(0.,1.,0.));
#23422=DIRECTION('ref_axis',(0.,0.,1.));
#23423=DIRECTION('center_axis',(-0.99957228042324,0.,-0.0292447637959857));
#23424=DIRECTION('ref_axis',(-0.0292447637959857,0.,0.99957228042324));
#23425=DIRECTION('center_axis',(0.,1.,0.));
#23426=DIRECTION('ref_axis',(0.,0.,1.));
#23427=DIRECTION('center_axis',(0.87052398911462,0.,-0.492125984251969));
#23428=DIRECTION('ref_axis',(-0.492125984251969,0.,-0.87052398911462));
#23429=DIRECTION('center_axis',(-0.859125449034146,0.00660004002305416,
-0.511722485624358));
#23430=DIRECTION('ref_axis',(0.00325484628249352,0.999967079615338,0.00743274251192558));
#23431=DIRECTION('center_axis',(0.,1.,0.));
#23432=DIRECTION('ref_axis',(0.,0.,1.));
#23433=DIRECTION('center_axis',(-0.860841979634013,0.,-0.508872367200061));
#23434=DIRECTION('ref_axis',(-0.508872367200061,0.,0.860841979634013));
#23435=DIRECTION('center_axis',(1.,0.,-2.77555756156291E-16));
#23436=DIRECTION('ref_axis',(-2.77555756156291E-16,0.,-1.));
#23437=DIRECTION('center_axis',(-0.860841979634012,0.,-0.508872367200063));
#23438=DIRECTION('ref_axis',(-0.508872367200063,0.,0.860841979634012));
#23439=DIRECTION('center_axis',(0.860841979634011,0.,0.508872367200065));
#23440=DIRECTION('ref_axis',(0.508872367200065,0.,-0.860841979634011));
#23441=DIRECTION('center_axis',(0.863246210589165,-0.00473021077503891,
0.504760938474315));
#23442=DIRECTION('ref_axis',(0.504766585555321,-4.22748313639192E-18,-0.863255868272451));
#23443=DIRECTION('center_axis',(0.864784496230593,-0.00574209397403801,
0.502110349859464));
#23444=DIRECTION('ref_axis',(-0.283224646410217,0.820121494130974,0.497176562732181));
#23445=DIRECTION('center_axis',(-1.,0.,2.77555756156289E-16));
#23446=DIRECTION('ref_axis',(2.77555756156289E-16,0.,1.));
#23447=DIRECTION('center_axis',(1.,0.,-8.67361737988409E-15));
#23448=DIRECTION('ref_axis',(-8.67361737988409E-15,0.,-1.));
#23449=DIRECTION('center_axis',(-0.860841979634012,0.,-0.508872367200063));
#23450=DIRECTION('ref_axis',(-0.508872367200063,0.,0.860841979634012));
#23451=DIRECTION('center_axis',(-0.860841979634013,-1.05194637034855E-14,
-0.508872367200061));
#23452=DIRECTION('ref_axis',(-0.508872367200061,-3.69238341666438E-31,0.860841979634013));
#23453=DIRECTION('center_axis',(0.,1.,0.));
#23454=DIRECTION('ref_axis',(0.,0.,1.));
#23455=DIRECTION('center_axis',(0.,-1.,0.));
#23456=DIRECTION('ref_axis',(0.,0.,-1.));
#23457=DIRECTION('center_axis',(-9.03800051153415E-15,1.,4.73307385236553E-15));
#23458=DIRECTION('ref_axis',(-1.,-9.03800051153415E-15,0.));
#23459=DIRECTION('center_axis',(-0.195513569438188,0.,0.980700996311077));
#23460=DIRECTION('ref_axis',(-0.980700996311077,0.,-0.195513569438188));
#23461=DIRECTION('center_axis',(-0.000553346312781574,0.999999846903545,
8.62668738358512E-7));
#23462=DIRECTION('ref_axis',(-0.999999846903917,-0.00055334631278159,0.));
#23463=DIRECTION('center_axis',(-0.863024574373895,-0.00477577234771503,
0.505139362973467));
#23464=DIRECTION('ref_axis',(-0.333722054577103,0.756073495912651,-0.563011952863578));
#23465=DIRECTION('center_axis',(0.,1.,0.));
#23466=DIRECTION('ref_axis',(0.,0.,1.));
#23467=DIRECTION('center_axis',(-1.,0.,0.));
#23468=DIRECTION('ref_axis',(0.,0.,1.));
#23469=DIRECTION('center_axis',(-1.7347234759768E-14,1.,8.67361737988401E-15));
#23470=DIRECTION('ref_axis',(-1.,-1.73472347597682E-14,0.));
#23471=DIRECTION('center_axis',(-0.885876528532336,0.,0.463921088328067));
#23472=DIRECTION('ref_axis',(0.463921088328067,0.,0.885876528532336));
#23473=DIRECTION('center_axis',(-0.885876528532327,0.,0.463921088328083));
#23474=DIRECTION('ref_axis',(0.463921088328083,0.,0.885876528532327));
#23475=DIRECTION('center_axis',(-0.885876528532327,0.,0.463921088328084));
#23476=DIRECTION('ref_axis',(0.463921088328084,0.,0.885876528532327));
#23477=DIRECTION('center_axis',(0.863167213322135,-0.00464466166563832,
-0.504896810213445));
#23478=DIRECTION('ref_axis',(-0.504902256341213,0.,-0.863176523974993));
#23479=DIRECTION('center_axis',(-0.859070797571545,0.00649965078107082,
0.511815512953167));
#23480=DIRECTION('ref_axis',(-0.360863243714502,0.701451263689212,-0.614608691774413));
#23481=DIRECTION('center_axis',(1.,0.,-2.77555756156289E-16));
#23482=DIRECTION('ref_axis',(-2.77555756156289E-16,0.,-1.));
#23483=DIRECTION('center_axis',(-1.,0.,3.4302489988858E-15));
#23484=DIRECTION('ref_axis',(3.4302489988858E-15,0.,1.));
#23485=DIRECTION('center_axis',(-0.885876528532327,0.,0.463921088328083));
#23486=DIRECTION('ref_axis',(0.463921088328083,0.,0.885876528532327));
#23487=DIRECTION('center_axis',(0.885876528532327,9.09984937312614E-17,
-0.463921088328084));
#23488=DIRECTION('ref_axis',(-0.463921088328084,-3.29612034119983E-33,-0.885876528532327));
#23489=DIRECTION('center_axis',(0.,1.,0.));
#23490=DIRECTION('ref_axis',(0.,0.,1.));
#23491=DIRECTION('center_axis',(0.885876528532327,0.,0.463921088328083));
#23492=DIRECTION('ref_axis',(0.463921088328083,0.,-0.885876528532327));
#23493=DIRECTION('center_axis',(0.,1.,0.));
#23494=DIRECTION('ref_axis',(0.,0.,1.));
#23495=DIRECTION('center_axis',(-0.860841979634015,0.,0.508872367200058));
#23496=DIRECTION('ref_axis',(0.508872367200058,0.,0.860841979634015));
#23497=DIRECTION('center_axis',(0.,1.,0.));
#23498=DIRECTION('ref_axis',(0.,0.,1.));
#23499=DIRECTION('center_axis',(-0.885876528532327,0.,-0.463921088328084));
#23500=DIRECTION('ref_axis',(-0.463921088328084,0.,0.885876528532327));
#23501=DIRECTION('center_axis',(0.885876528532327,0.,0.463921088328083));
#23502=DIRECTION('ref_axis',(0.463921088328083,0.,-0.885876528532327));
#23503=DIRECTION('center_axis',(-0.195513569438188,0.,-0.980700996311077));
#23504=DIRECTION('ref_axis',(0.980700996311077,0.,-0.195513569438188));
#23505=DIRECTION('center_axis',(0.860841979634012,0.,-0.508872367200063));
#23506=DIRECTION('ref_axis',(-0.508872367200063,0.,-0.860841979634012));
#23507=DIRECTION('center_axis',(0.860841979634013,0.,-0.508872367200061));
#23508=DIRECTION('ref_axis',(-0.508872367200061,0.,-0.860841979634013));
#23509=DIRECTION('center_axis',(0.860841979634012,0.,-0.508872367200063));
#23510=DIRECTION('ref_axis',(-0.508872367200063,0.,-0.860841979634012));
#23511=DIRECTION('center_axis',(-0.860841979634021,0.,0.508872367200048));
#23512=DIRECTION('ref_axis',(0.508872367200048,0.,0.860841979634021));
#23513=DIRECTION('center_axis',(0.885876528532327,0.,0.463921088328083));
#23514=DIRECTION('ref_axis',(0.463921088328083,0.,-0.885876528532327));
#23515=DIRECTION('center_axis',(-0.885876528532327,-1.93913821232359E-14,
-0.463921088328084));
#23516=DIRECTION('ref_axis',(-0.463921088328084,-1.07766259570539E-30,0.885876528532327));
#23517=DIRECTION('center_axis',(0.,-1.,0.));
#23518=DIRECTION('ref_axis',(0.,0.,-1.));
#23519=DIRECTION('center_axis',(-1.7347234759768E-14,1.,0.));
#23520=DIRECTION('ref_axis',(-1.,-1.73472347597682E-14,0.));
#23521=DIRECTION('center_axis',(8.7825899001661E-15,1.,-5.19168142165297E-15));
#23522=DIRECTION('ref_axis',(-1.,8.7825899001661E-15,0.));
#23523=DIRECTION('center_axis',(0.,1.,0.));
#23524=DIRECTION('ref_axis',(0.,0.,1.));
#23525=DIRECTION('center_axis',(0.,1.,0.));
#23526=DIRECTION('ref_axis',(0.,0.,1.));
#23527=DIRECTION('center_axis',(0.,1.,0.));
#23528=DIRECTION('ref_axis',(0.,0.,1.));
#23529=DIRECTION('center_axis',(1.,0.,-1.77635683940025E-16));
#23530=DIRECTION('ref_axis',(-1.77635683940025E-16,0.,-1.));
#23531=DIRECTION('center_axis',(0.,1.,0.));
#23532=DIRECTION('ref_axis',(0.,0.,1.));
#23533=DIRECTION('center_axis',(-1.,0.,2.36217664813863E-16));
#23534=DIRECTION('ref_axis',(-2.36217664813863E-16,0.,-1.));
#23535=DIRECTION('center_axis',(-0.857824537815853,0.,-0.513942664429622));
#23536=DIRECTION('ref_axis',(-0.513942664429622,0.,0.857824537815853));
#23537=DIRECTION('center_axis',(0.860841979634012,0.,0.508872367200063));
#23538=DIRECTION('ref_axis',(0.508872367200063,0.,-0.860841979634012));
#23539=DIRECTION('center_axis',(0.860841979634013,0.,0.508872367200061));
#23540=DIRECTION('ref_axis',(0.508872367200061,0.,-0.860841979634013));
#23541=DIRECTION('center_axis',(-0.86396885760878,-3.77362398313829E-13,
-0.503545244324857));
#23542=DIRECTION('ref_axis',(-0.40193736700939,-0.602372654072851,0.689632901351718));
#23543=DIRECTION('center_axis',(0.,1.,0.));
#23544=DIRECTION('ref_axis',(0.,0.,1.));
#23545=DIRECTION('center_axis',(1.,0.,0.));
#23546=DIRECTION('ref_axis',(0.,0.,-1.));
#23547=DIRECTION('center_axis',(0.000484671251441277,0.999999882395689,
-1.73892337407491E-5));
#23548=DIRECTION('ref_axis',(-0.999999882546882,0.000484671251514543,0.));
#23549=DIRECTION('center_axis',(-0.863965003980117,8.6132890394033E-13,
0.503551856215065));
#23550=DIRECTION('ref_axis',(-6.88338275267738E-13,-1.,5.35682609381748E-13));
#23551=DIRECTION('center_axis',(1.,0.,-2.77555756156289E-16));
#23552=DIRECTION('ref_axis',(-2.77555756156289E-16,0.,-1.));
#23553=DIRECTION('center_axis',(1.,0.,0.));
#23554=DIRECTION('ref_axis',(0.,0.,-1.));
#23555=DIRECTION('center_axis',(0.857823788622072,0.,-0.513943914911028));
#23556=DIRECTION('ref_axis',(-0.513943914911028,0.,-0.857823788622072));
#23557=DIRECTION('center_axis',(0.,1.,0.));
#23558=DIRECTION('ref_axis',(0.,0.,1.));
#23559=DIRECTION('center_axis',(-1.,0.,0.));
#23560=DIRECTION('ref_axis',(0.,0.,1.));
#23561=DIRECTION('center_axis',(-1.,0.,2.77555756156289E-16));
#23562=DIRECTION('ref_axis',(2.77555756156289E-16,0.,1.));
#23563=DIRECTION('center_axis',(-1.,-3.15269324272952E-15,2.7755575615626E-16));
#23564=DIRECTION('ref_axis',(3.15269324272952E-15,-1.,-5.15124444202338E-47));
#23565=DIRECTION('center_axis',(-0.860841979634012,0.,0.508872367200063));
#23566=DIRECTION('ref_axis',(0.508872367200063,0.,0.860841979634012));
#23567=DIRECTION('center_axis',(0.860841979634013,0.,-0.508872367200061));
#23568=DIRECTION('ref_axis',(-0.508872367200061,0.,-0.860841979634013));
#23569=DIRECTION('center_axis',(0.,1.,0.));
#23570=DIRECTION('ref_axis',(0.,0.,1.));
#23571=DIRECTION('center_axis',(0.,1.,0.));
#23572=DIRECTION('ref_axis',(-1.,0.,-1.83697019872103E-16));
#23573=DIRECTION('center_axis',(0.,1.,0.));
#23574=DIRECTION('ref_axis',(1.,0.,6.12323399573677E-17));
#23575=DIRECTION('center_axis',(0.,1.,0.));
#23576=DIRECTION('ref_axis',(0.,0.,1.));
#23577=DIRECTION('center_axis',(-1.,0.,2.36217664813863E-16));
#23578=DIRECTION('ref_axis',(-2.36217664813863E-16,0.,-1.));
#23579=DIRECTION('center_axis',(0.,1.,0.));
#23580=DIRECTION('ref_axis',(0.,0.,1.));
#23581=DIRECTION('center_axis',(-1.,0.,0.));
#23582=DIRECTION('ref_axis',(0.,0.,-1.));
#23583=DIRECTION('center_axis',(1.,0.,0.));
#23584=DIRECTION('ref_axis',(0.,-1.,0.));
#23585=DIRECTION('center_axis',(-0.99957228042324,4.08129586043321E-15,
0.029244763795984));
#23586=DIRECTION('ref_axis',(0.029244763795984,-9.77391875425212E-33,0.99957228042324));
#23587=DIRECTION('center_axis',(0.,1.,0.));
#23588=DIRECTION('ref_axis',(1.,0.,7.04481399828022E-16));
#23589=DIRECTION('center_axis',(-0.87052398911462,0.,0.492125984251969));
#23590=DIRECTION('ref_axis',(0.492125984251969,0.,0.87052398911462));
#23591=DIRECTION('center_axis',(-0.87052398911462,-4.26851249010043E-15,
-0.492125984251969));
#23592=DIRECTION('ref_axis',(-0.492125984251969,3.56763598725556E-30,0.87052398911462));
#23593=DIRECTION('center_axis',(0.492125984251969,0.,0.87052398911462));
#23594=DIRECTION('ref_axis',(0.870523989114618,0.,-0.492125984251973));
#23595=DIRECTION('center_axis',(0.,1.,0.));
#23596=DIRECTION('ref_axis',(0.,0.,1.));
#23597=DIRECTION('center_axis',(0.492125984251969,0.,-0.87052398911462));
#23598=DIRECTION('ref_axis',(-0.870523989114623,0.,-0.492125984251964));
#23599=DIRECTION('center_axis',(0.,1.,0.));
#23600=DIRECTION('ref_axis',(0.,0.,1.));
#23601=DIRECTION('center_axis',(0.,-1.,0.));
#23602=DIRECTION('ref_axis',(-2.20819958125884E-14,0.,1.));
#23603=DIRECTION('center_axis',(0.,1.,0.));
#23604=DIRECTION('ref_axis',(0.,0.,1.));
#23605=DIRECTION('center_axis',(0.,1.,0.));
#23606=DIRECTION('ref_axis',(0.240266771500873,0.,-0.970706896293906));
#23607=DIRECTION('center_axis',(0.,-1.,0.));
#23608=DIRECTION('ref_axis',(0.,0.,-1.));
#23609=DIRECTION('center_axis',(0.851950674417188,3.69474708821441E-15,
-0.523622047244097));
#23610=DIRECTION('ref_axis',(-0.523622047244097,7.84320521258019E-32,-0.851950674417188));
#23611=DIRECTION('center_axis',(0.,1.,0.));
#23612=DIRECTION('ref_axis',(0.,0.,1.));
#23613=DIRECTION('center_axis',(0.875811224577025,6.4333293152058E-5,0.48265380425945));
#23614=DIRECTION('ref_axis',(0.482653805258247,0.,-0.875811226389417));
#23615=DIRECTION('center_axis',(-0.224058013086413,0.885784476176752,0.406428183737356));
#23616=DIRECTION('ref_axis',(0.890655349196501,0.0168104402479641,0.454368196561257));
#23617=DIRECTION('center_axis',(-0.822444407952205,-0.295329920203461,-0.486174283627554));
#23618=DIRECTION('ref_axis',(-0.508872367200061,2.60023830660238E-16,0.860841979634013));
#23619=DIRECTION('center_axis',(-0.00270036335398834,-0.999995105202431,
-0.00158038252836222));
#23620=DIRECTION('ref_axis',(0.509072475055034,-1.44080963018857E-5,-0.860723657705392));
#23621=DIRECTION('center_axis',(0.00227714854045241,0.999996496446841,0.00134969943612062));
#23622=DIRECTION('ref_axis',(-0.999997407289178,0.00227715061458298,-6.8912051966359E-21));
#23623=DIRECTION('center_axis',(0.0027029442948384,0.999995097323232,0.00158095592591226));
#23624=DIRECTION('ref_axis',(0.444580341019544,0.000214448963012711,-0.895738954378221));
#23625=DIRECTION('center_axis',(0.000103527088607853,0.999999992623769,
6.35185350686548E-5));
#23626=DIRECTION('ref_axis',(-0.999999994641071,0.000103527088816698,-3.76084161841949E-23));
#23627=DIRECTION('center_axis',(-0.00214831185033822,0.999997022148358,
-0.00115777830791125));
#23628=DIRECTION('ref_axis',(0.438135237678527,-9.94865870677395E-5,-0.898909063035188));
#23629=DIRECTION('center_axis',(0.819672096105927,-0.305553637946519,0.484535477754687));
#23630=DIRECTION('ref_axis',(0.508872367200059,1.84629072854334E-16,-0.860841979634014));
#23631=DIRECTION('center_axis',(-0.282731426109906,-0.801305881909544,0.527230333257702));
#23632=DIRECTION('ref_axis',(0.407870460957109,-0.59792211370622,-0.690022342406187));
#23633=DIRECTION('center_axis',(0.881188233597026,-0.00024684095531491,
0.472765519089217));
#23634=DIRECTION('ref_axis',(0.472765533492127,-2.08912278962891E-20,-0.881188260442628));
#23635=DIRECTION('center_axis',(0.881643835712412,-0.000205864534824282,
-0.471915357421328));
#23636=DIRECTION('ref_axis',(-0.471915367421263,4.31856925775005E-20,-0.881643854394536));
#23637=DIRECTION('center_axis',(-0.285649301116541,-0.795890144086274,-0.533819590609002));
#23638=DIRECTION('ref_axis',(0.345501431459368,-0.605095435813926,0.717278380000877));
#23639=DIRECTION('center_axis',(-0.81846149474772,0.309901812552962,0.483819850969052));
#23640=DIRECTION('ref_axis',(0.508872367200115,1.08402883170529E-16,0.860841979633981));
#23641=DIRECTION('center_axis',(-0.0235631216677967,0.999626094909593,0.0138726231501557));
#23642=DIRECTION('ref_axis',(0.509367231127245,6.42305444620244E-5,0.860549254678778));
#23643=DIRECTION('center_axis',(-0.0224243417675557,0.999660615912144,0.0132590305243092));
#23644=DIRECTION('ref_axis',(-0.999748498612813,-0.0224263131483262,1.07790531220658E-18));
#23645=DIRECTION('center_axis',(0.0214414384172488,-0.999689035276165,-0.012731750359262));
#23646=DIRECTION('ref_axis',(0.435401828077164,-0.00212657061748541,0.900233706214376));
#23647=DIRECTION('center_axis',(-0.0204053358968825,0.999719111022908,0.0120549293860458));
#23648=DIRECTION('ref_axis',(-0.999791759192672,-0.0204068187236985,-4.51782575218622E-19));
#23649=DIRECTION('center_axis',(0.0187793084075624,-0.999761209584918,-0.0111741391183278));
#23650=DIRECTION('ref_axis',(0.442592142534916,-0.00170892344078755,0.896721403194452));
#23651=DIRECTION('center_axis',(-0.0192244218537273,0.999750649496634,0.0113604769023756));
#23652=DIRECTION('ref_axis',(-0.999815169869054,-0.0192256625299481,-2.76063375332087E-19));
#23653=DIRECTION('center_axis',(0.0188072437744052,-0.999761138089071,-0.0111334787221499));
#23654=DIRECTION('ref_axis',(0.446265374922732,-0.00157069574366981,0.894899294926504));
#23655=DIRECTION('center_axis',(0.821930410018369,0.297254628825937,-0.4858704423286));
#23656=DIRECTION('ref_axis',(-0.508872367200098,1.3431595397086E-16,-0.860841979633991));
#23657=DIRECTION('center_axis',(-0.224582549367916,0.885152773348463,-0.407513492234224));
#23658=DIRECTION('ref_axis',(0.423300985656642,0.465295843830645,0.777377677358981));
#23659=DIRECTION('center_axis',(0.875783254496798,9.66947566949944E-5,-0.482704549173841));
#23660=DIRECTION('ref_axis',(-0.482704551430455,-1.00776139250218E-19,-0.87578325859103));
#23661=DIRECTION('center_axis',(0.,-1.,0.));
#23662=DIRECTION('ref_axis',(0.,0.,-1.));
#23663=DIRECTION('',(0.,-1.,0.));
#23664=DIRECTION('center_axis',(0.,-1.,0.));
#23665=DIRECTION('ref_axis',(0.,0.,-1.));
#23666=DIRECTION('',(0.,-1.,0.));
#23667=DIRECTION('center_axis',(0.,-1.,0.));
#23668=DIRECTION('ref_axis',(0.,0.,-1.));
#23669=DIRECTION('',(0.,-1.,0.));
#23670=DIRECTION('center_axis',(0.,-1.,0.));
#23671=DIRECTION('ref_axis',(0.,0.,-1.));
#23672=DIRECTION('',(0.,-1.,0.));
#23673=DIRECTION('center_axis',(-1.,0.,0.));
#23674=DIRECTION('ref_axis',(0.,0.,1.));
#23675=DIRECTION('center_axis',(0.,-1.,2.22044604925031E-16));
#23676=DIRECTION('ref_axis',(0.,-2.22044604925031E-16,-1.));
#49131=CARTESIAN_POINT('',(0.,0.,0.));
#49132=CARTESIAN_POINT('Ctrl Pts',(-0.047521969753009,0.00292791234232007,
0.0014375007351075));
#49133=CARTESIAN_POINT('Ctrl Pts',(-0.0475217905822521,0.00272283848633948,
0.00149851530284684));
#49134=CARTESIAN_POINT('Ctrl Pts',(-0.0475249292449862,0.00279751942631425,
0.00169899223914139));
#49135=CARTESIAN_POINT('Ctrl Pts',(-0.0471359306861318,0.00292980295225596,
0.00144284563795755));
#49136=CARTESIAN_POINT('Ctrl Pts',(-0.0471283033320531,0.0027246802372573,
0.00150425289890676));
#49137=CARTESIAN_POINT('Ctrl Pts',(-0.0470869890419856,0.00279975471284071,
0.00170530652254621));
#49138=CARTESIAN_POINT('Ctrl Pts',(-0.0463597555989418,0.00281040271795959,
0.00116400921661837));
#49139=CARTESIAN_POINT('Ctrl Pts',(-0.0463911712050714,0.00262787967136623,
0.00125349479954789));
#49140=CARTESIAN_POINT('Ctrl Pts',(-0.0462058670420217,0.0026583834282292,
0.00137542120560276));
#49141=CARTESIAN_POINT('Ctrl Pts',(-0.0458448108046749,0.00261243102946703,
2.73686784603569E-5));
#49142=CARTESIAN_POINT('Ctrl Pts',(-0.0458094820998151,0.00243981891809829,
3.02504277461982E-5));
#49143=CARTESIAN_POINT('Ctrl Pts',(-0.0456221070083461,0.00242419343546418,
3.23331464450899E-5));
#49144=CARTESIAN_POINT('Ctrl Pts',(-0.0463246614268507,0.00279922894991229,
-0.00113315917795547));
#49145=CARTESIAN_POINT('Ctrl Pts',(-0.0463534248332843,0.00261785874660286,
-0.00122287857653879));
#49146=CARTESIAN_POINT('Ctrl Pts',(-0.0461660653383145,0.00264516117224189,
-0.00133894667362545));
#49147=CARTESIAN_POINT('Ctrl Pts',(-0.047475667560966,0.00298937709191257,
-0.00158152248003427));
#49148=CARTESIAN_POINT('Ctrl Pts',(-0.0474776982153359,0.0027762552545778,
-0.00163733766341943));
#49149=CARTESIAN_POINT('Ctrl Pts',(-0.0474723735075983,0.00287024649410696,
-0.00186926883315251));
#49150=CARTESIAN_POINT('Ctrl Pts',(-0.0486390883124264,0.00281072577948571,
-0.00116572585728214));
#49151=CARTESIAN_POINT('Ctrl Pts',(-0.048607647449207,0.00262816948297617,
-0.00125530022942588));
#49152=CARTESIAN_POINT('Ctrl Pts',(-0.0487928212048197,0.00265876571215968,
-0.00137744992107542));
#49153=CARTESIAN_POINT('Ctrl Pts',(-0.0491553277660853,0.00261238743571346,
-2.56552014422379E-5));
#49154=CARTESIAN_POINT('Ctrl Pts',(-0.0491906502037132,0.00243978444592517,
-2.85609443699274E-5));
#49155=CARTESIAN_POINT('Ctrl Pts',(-0.0493780503329557,0.00242414178609795,
-3.03066921536269E-5));
#49156=CARTESIAN_POINT('Ctrl Pts',(-0.0486760035727277,0.00279905892909024,
0.00113193946402892));
#49157=CARTESIAN_POINT('Ctrl Pts',(-0.0486472257773982,0.00261770650436948,
0.00122160652879805));
#49158=CARTESIAN_POINT('Ctrl Pts',(-0.0488346894846697,0.00264495997721764,
0.00133750508047801));
#49159=CARTESIAN_POINT('Ctrl Pts',(-0.0479080088854605,0.00292602173206304,
0.00143215583134954));
#49160=CARTESIAN_POINT('Ctrl Pts',(-0.0479147483545036,0.00272099921368874,
0.00149278542731809));
#49161=CARTESIAN_POINT('Ctrl Pts',(-0.0479628751525174,0.00279528411067136,
0.00169267787348785));
#49162=CARTESIAN_POINT('Ctrl Pts',(-0.047521969753009,0.00292791234232007,
0.0014375007351075));
#49163=CARTESIAN_POINT('Ctrl Pts',(-0.0475217905822521,0.00272283848633948,
0.00149851530284684));
#49164=CARTESIAN_POINT('Ctrl Pts',(-0.0475249292449862,0.00279751942631425,
0.00169899223914139));
#49165=CARTESIAN_POINT('',(-0.0475248989283422,0.00279679729590145,0.00169705696579711));
#49166=CARTESIAN_POINT('',(-0.047521969610817,0.00292787381968359,0.00143750579808091));
#49167=CARTESIAN_POINT('Ctrl Pts',(-0.047524898940367,0.0027968083975309,
0.00169705296016689));
#49168=CARTESIAN_POINT('Ctrl Pts',(-0.0475217930237305,0.00272496362417165,
0.00149792539327892));
#49169=CARTESIAN_POINT('Ctrl Pts',(-0.0475219697209349,0.00292787557066265,
0.00143751167942811));
#49170=CARTESIAN_POINT('',(-0.0475,0.002796875,0.00169723753033423));
#49171=CARTESIAN_POINT('Ctrl Pts',(-0.0475,0.002796875,0.00169723753033423));
#49172=CARTESIAN_POINT('Ctrl Pts',(-0.0470556118872741,0.00279685666170104,
0.00169708273941662));
#49173=CARTESIAN_POINT('Ctrl Pts',(-0.0461665719179776,0.00264539629297986,
0.00133451307288424));
#49174=CARTESIAN_POINT('Ctrl Pts',(-0.0456341151866447,0.00242721165967408,
2.04143110301131E-6));
#49175=CARTESIAN_POINT('Ctrl Pts',(-0.0461678030184114,0.00264575759329887,
-0.00133706644457989));
#49176=CARTESIAN_POINT('Ctrl Pts',(-0.0475004674124815,0.00287245605236691,
-0.00187753708326946));
#49177=CARTESIAN_POINT('Ctrl Pts',(-0.0488323000379284,0.00264566812967151,
-0.00133621021713015));
#49178=CARTESIAN_POINT('Ctrl Pts',(-0.0493659912919883,0.00242720638772112,
8.03570479835991E-8));
#49179=CARTESIAN_POINT('Ctrl Pts',(-0.0488362194957707,0.00264414723702811,
0.00132712816164593));
#49180=CARTESIAN_POINT('Ctrl Pts',(-0.0479609366490351,0.00279406634542388,
0.00169058598422321));
#49181=CARTESIAN_POINT('Ctrl Pts',(-0.0475248989283412,0.00279679729590146,
0.00169705696579713));
#49182=CARTESIAN_POINT('',(-0.0475,0.00292794117647059,0.00143766002569487));
#49183=CARTESIAN_POINT('Ctrl Pts',(-0.0474999999943631,0.00279686254156731,
0.00169724202650596));
#49184=CARTESIAN_POINT('Ctrl Pts',(-0.047499419575665,0.00272498843318775,
0.00149808548501933));
#49185=CARTESIAN_POINT('Ctrl Pts',(-0.0475000000046904,0.00292793913822137,
0.00143765318065731));
#49186=CARTESIAN_POINT('',(-0.0464613877374918,0.00280559596990715,0.00103824715833725));
#49187=CARTESIAN_POINT('Ctrl Pts',(-0.0464613877374919,0.00280559596990715,
0.00103824715833725));
#49188=CARTESIAN_POINT('Ctrl Pts',(-0.0467365913194384,0.0028677273296309,
0.00129598001878092));
#49189=CARTESIAN_POINT('Ctrl Pts',(-0.0471182158646947,0.0029279629632896,
0.00143762672627057));
#49190=CARTESIAN_POINT('Ctrl Pts',(-0.0475,0.00292794117647059,0.00143766002569487));
#49191=CARTESIAN_POINT('',(-0.0460105501879809,0.00267652225571725,2.02991083324788E-5));
#49192=CARTESIAN_POINT('Ctrl Pts',(-0.0460105501879809,0.00267652225571725,
2.02991083324788E-5));
#49193=CARTESIAN_POINT('Ctrl Pts',(-0.0460158709169045,0.0026785745264266,
0.000396779691601982));
#49194=CARTESIAN_POINT('Ctrl Pts',(-0.0461825726657913,0.00274235049501108,
0.000774645398476074));
#49195=CARTESIAN_POINT('Ctrl Pts',(-0.0464582351392805,0.00280488422330797,
0.00103529469620324));
#49196=CARTESIAN_POINT('Ctrl Pts',(-0.0464613877374919,0.00280559596990715,
0.00103824715833725));
#49197=CARTESIAN_POINT('',(-0.0464522715406983,0.00280353121836822,-0.00102962802751535));
#49198=CARTESIAN_POINT('Ctrl Pts',(-0.0464522715406983,0.00280353121836822,
-0.00102962802751535));
#49199=CARTESIAN_POINT('Ctrl Pts',(-0.0461764109517263,0.00274067965092877,
-0.000765636240703534));
#49200=CARTESIAN_POINT('Ctrl Pts',(-0.0460077424451037,0.00267543025507494,
-0.000375293469169163));
#49201=CARTESIAN_POINT('Ctrl Pts',(-0.0460104603923367,0.0026764876204308,
1.39454081202657E-5));
#49202=CARTESIAN_POINT('Ctrl Pts',(-0.0460105501879809,0.00267652225571725,
2.02991083324788E-5));
#49203=CARTESIAN_POINT('',(-0.0485379243677292,0.0028057609228668,-0.00103890261335411));
#49204=CARTESIAN_POINT('Ctrl Pts',(-0.0485379243677292,0.0028057609228668,
-0.00103890261335411));
#49205=CARTESIAN_POINT('Ctrl Pts',(-0.0482626321295759,0.00286788646427852,
-0.00129688101678008));
#49206=CARTESIAN_POINT('Ctrl Pts',(-0.0474954951077672,0.00298874310808213,
-0.00158006024895397));
#49207=CARTESIAN_POINT('Ctrl Pts',(-0.0467281321296702,0.00286638278580766,
-0.00129361981432716));
#49208=CARTESIAN_POINT('Ctrl Pts',(-0.0464522715406983,0.00280353121836822,
-0.00102962802751535));
#49209=CARTESIAN_POINT('',(-0.0489894472304209,0.00267652109012544,-1.8656167423741E-5));
#49210=CARTESIAN_POINT('Ctrl Pts',(-0.0489894472304209,0.00267652109012544,
-1.8656167423741E-5));
#49211=CARTESIAN_POINT('Ctrl Pts',(-0.0489840520567291,0.00267855735573614,
-0.000395630752060275));
#49212=CARTESIAN_POINT('Ctrl Pts',(-0.0488168919200026,0.00274251464423592,
-0.000775051359101422));
#49213=CARTESIAN_POINT('Ctrl Pts',(-0.0485409904223183,0.00280506900251836,
-0.0010360293907997));
#49214=CARTESIAN_POINT('Ctrl Pts',(-0.0485379243677292,0.0028057609228668,
-0.00103890261335411));
#49215=CARTESIAN_POINT('',(-0.0485484173841136,0.00280336755518862,0.0010289747883925));
#49216=CARTESIAN_POINT('Ctrl Pts',(-0.0485484173841136,0.00280336755518862,
0.0010289747883925));
#49217=CARTESIAN_POINT('Ctrl Pts',(-0.0488243561640007,0.00274048389401599,
0.000765098689612273));
#49218=CARTESIAN_POINT('Ctrl Pts',(-0.0489924898026455,0.00267538673953036,
0.000376229036000762));
#49219=CARTESIAN_POINT('Ctrl Pts',(-0.0489895325382811,0.00267648889292995,
-1.26954890466987E-5));
#49220=CARTESIAN_POINT('Ctrl Pts',(-0.0489894472304209,0.00267652109012544,
-1.8656167423741E-5));
#49221=CARTESIAN_POINT('Ctrl Pts',(-0.047521969610817,0.00292787381968359,
0.0014375057980809));
#49222=CARTESIAN_POINT('Ctrl Pts',(-0.0479007709531672,0.00292557966528534,
0.00143215706955921));
#49223=CARTESIAN_POINT('Ctrl Pts',(-0.0482777117231938,0.00286505864139897,
0.00128784653432999));
#49224=CARTESIAN_POINT('Ctrl Pts',(-0.0485484173841136,0.00280336755518862,
0.0010289747883925));
#49225=CARTESIAN_POINT('Ctrl Pts',(-0.0675219697530089,0.00292791234232007,
0.0014375007351075));
#49226=CARTESIAN_POINT('Ctrl Pts',(-0.0675217905822521,0.00272283848633946,
0.00149851530284684));
#49227=CARTESIAN_POINT('Ctrl Pts',(-0.0675249292449862,0.00279751942631426,
0.00169899223914141));
#49228=CARTESIAN_POINT('Ctrl Pts',(-0.0671359306861318,0.00292980295225596,
0.00144284563795754));
#49229=CARTESIAN_POINT('Ctrl Pts',(-0.0671283033320531,0.00272468023725727,
0.00150425289890677));
#49230=CARTESIAN_POINT('Ctrl Pts',(-0.0670869890419856,0.00279975471284072,
0.00170530652254623));
#49231=CARTESIAN_POINT('Ctrl Pts',(-0.0663597555989418,0.00281040271795959,
0.00116400921661836));
#49232=CARTESIAN_POINT('Ctrl Pts',(-0.0663911712050714,0.00262787967136621,
0.00125349479954789));
#49233=CARTESIAN_POINT('Ctrl Pts',(-0.0662058670420217,0.0026583834282292,
0.00137542120560276));
#49234=CARTESIAN_POINT('Ctrl Pts',(-0.065844810804675,0.00261243102946704,
2.73686784603625E-5));
#49235=CARTESIAN_POINT('Ctrl Pts',(-0.0658094820998151,0.00243981891809827,
3.02504277462119E-5));
#49236=CARTESIAN_POINT('Ctrl Pts',(-0.0656221070083461,0.00242419343546418,
3.23331464450973E-5));
#49237=CARTESIAN_POINT('Ctrl Pts',(-0.0663246614268507,0.00279922894991229,
-0.00113315917795546));
#49238=CARTESIAN_POINT('Ctrl Pts',(-0.0663534248332843,0.00261785874660285,
-0.00122287857653879));
#49239=CARTESIAN_POINT('Ctrl Pts',(-0.0661660653383145,0.00264516117224189,
-0.00133894667362545));
#49240=CARTESIAN_POINT('Ctrl Pts',(-0.067475667560966,0.00298937709191257,
-0.00158152248003427));
#49241=CARTESIAN_POINT('Ctrl Pts',(-0.0674776982153359,0.00277625525457778,
-0.00163733766341944));
#49242=CARTESIAN_POINT('Ctrl Pts',(-0.0674723735075983,0.00287024649410697,
-0.00186926883315253));
#49243=CARTESIAN_POINT('Ctrl Pts',(-0.0686390883124264,0.00281072577948571,
-0.00116572585728214));
#49244=CARTESIAN_POINT('Ctrl Pts',(-0.068607647449207,0.00262816948297615,
-0.0012553002294259));
#49245=CARTESIAN_POINT('Ctrl Pts',(-0.0687928212048197,0.00265876571215968,
-0.00137744992107544));
#49246=CARTESIAN_POINT('Ctrl Pts',(-0.0691553277660854,0.00261238743571347,
-2.56552014422452E-5));
#49247=CARTESIAN_POINT('Ctrl Pts',(-0.0691906502037132,0.00243978444592516,
-2.85609443699341E-5));
#49248=CARTESIAN_POINT('Ctrl Pts',(-0.0693780503329557,0.00242414178609795,
-3.03066921536361E-5));
#49249=CARTESIAN_POINT('Ctrl Pts',(-0.0686760035727276,0.00279905892909023,
0.00113193946402892));
#49250=CARTESIAN_POINT('Ctrl Pts',(-0.0686472257773982,0.00261770650436945,
0.00122160652879807));
#49251=CARTESIAN_POINT('Ctrl Pts',(-0.0688346894846698,0.00264495997721765,
0.00133750508047802));
#49252=CARTESIAN_POINT('Ctrl Pts',(-0.0679080088854605,0.00292602173206304,
0.00143215583134953));
#49253=CARTESIAN_POINT('Ctrl Pts',(-0.0679147483545036,0.00272099921368871,
0.0014927854273181));
#49254=CARTESIAN_POINT('Ctrl Pts',(-0.0679628751525174,0.00279528411067137,
0.00169267787348788));
#49255=CARTESIAN_POINT('Ctrl Pts',(-0.0675219697530089,0.00292791234232007,
0.0014375007351075));
#49256=CARTESIAN_POINT('Ctrl Pts',(-0.0675217905822521,0.00272283848633946,
0.00149851530284684));
#49257=CARTESIAN_POINT('Ctrl Pts',(-0.0675249292449862,0.00279751942631426,
0.00169899223914141));
#49258=CARTESIAN_POINT('',(-0.0675248989283422,0.00279679729590145,0.00169705696579711));
#49259=CARTESIAN_POINT('',(-0.067521969610817,0.00292787381968359,0.00143750579808091));
#49260=CARTESIAN_POINT('Ctrl Pts',(-0.067524898940367,0.0027968083975309,
0.00169705296016689));
#49261=CARTESIAN_POINT('Ctrl Pts',(-0.0675217930237306,0.00272496362417165,
0.00149792539327892));
#49262=CARTESIAN_POINT('Ctrl Pts',(-0.0675219697209349,0.00292787557066265,
0.00143751167942811));
#49263=CARTESIAN_POINT('',(-0.0675,0.002796875,0.00169723753033423));
#49264=CARTESIAN_POINT('Ctrl Pts',(-0.0675,0.002796875,0.00169723753033423));
#49265=CARTESIAN_POINT('Ctrl Pts',(-0.0670556118872741,0.00279685666170104,
0.00169708273941661));
#49266=CARTESIAN_POINT('Ctrl Pts',(-0.0661665719179776,0.00264539629297987,
0.00133451307288425));
#49267=CARTESIAN_POINT('Ctrl Pts',(-0.0656341151866447,0.00242721165967408,
2.0414311030091E-6));
#49268=CARTESIAN_POINT('Ctrl Pts',(-0.0661678030184114,0.00264575759329887,
-0.00133706644457988));
#49269=CARTESIAN_POINT('Ctrl Pts',(-0.0675004674124815,0.00287245605236691,
-0.00187753708326946));
#49270=CARTESIAN_POINT('Ctrl Pts',(-0.0688323000379284,0.00264566812967151,
-0.00133621021713016));
#49271=CARTESIAN_POINT('Ctrl Pts',(-0.0693659912919883,0.00242720638772113,
8.0357047990023E-8));
#49272=CARTESIAN_POINT('Ctrl Pts',(-0.0688362194957707,0.00264414723702811,
0.00132712816164593));
#49273=CARTESIAN_POINT('Ctrl Pts',(-0.0679609366490351,0.00279406634542389,
0.00169058598422322));
#49274=CARTESIAN_POINT('Ctrl Pts',(-0.0675248989283412,0.00279679729590146,
0.00169705696579713));
#49275=CARTESIAN_POINT('',(-0.0675,0.00292794117647059,0.00143766002569487));
#49276=CARTESIAN_POINT('Ctrl Pts',(-0.0674999999943631,0.00279686254156731,
0.00169724202650596));
#49277=CARTESIAN_POINT('Ctrl Pts',(-0.0674994195756651,0.00272498843318775,
0.00149808548501933));
#49278=CARTESIAN_POINT('Ctrl Pts',(-0.0675000000046904,0.00292793913822137,
0.00143765318065731));
#49279=CARTESIAN_POINT('',(-0.0664613877374912,0.002805595969907,0.00103824715833662));
#49280=CARTESIAN_POINT('Ctrl Pts',(-0.0664613877374912,0.002805595969907,
0.00103824715833662));
#49281=CARTESIAN_POINT('Ctrl Pts',(-0.0667365913194378,0.0028677273296308,
0.00129598001878069));
#49282=CARTESIAN_POINT('Ctrl Pts',(-0.0671182158646944,0.0029279629632896,
0.00143762672627058));
#49283=CARTESIAN_POINT('Ctrl Pts',(-0.0675,0.00292794117647059,0.00143766002569488));
#49284=CARTESIAN_POINT('',(-0.0660105501879809,0.00267652225571724,2.02991083315871E-5));
#49285=CARTESIAN_POINT('Ctrl Pts',(-0.0660105501879809,0.00267652225571724,
2.0299108331587E-5));
#49286=CARTESIAN_POINT('Ctrl Pts',(-0.0660158709169042,0.0026785745264265,
0.000396779691601394));
#49287=CARTESIAN_POINT('Ctrl Pts',(-0.0661825726657909,0.00274235049501098,
0.000774645398475571));
#49288=CARTESIAN_POINT('Ctrl Pts',(-0.0664582351392801,0.00280488422330787,
0.00103529469620283));
#49289=CARTESIAN_POINT('Ctrl Pts',(-0.0664613877374912,0.002805595969907,
0.00103824715833662));
#49290=CARTESIAN_POINT('',(-0.0664522715406983,0.00280353121836822,-0.00102962802751535));
#49291=CARTESIAN_POINT('Ctrl Pts',(-0.0664522715406983,0.00280353121836822,
-0.00102962802751535));
#49292=CARTESIAN_POINT('Ctrl Pts',(-0.0661764109517263,0.00274067965092877,
-0.000765636240703538));
#49293=CARTESIAN_POINT('Ctrl Pts',(-0.0660077424451038,0.00267543025507499,
-0.000375293469169463));
#49294=CARTESIAN_POINT('Ctrl Pts',(-0.0660104603923367,0.0026764876204308,
1.39454081196724E-5));
#49295=CARTESIAN_POINT('Ctrl Pts',(-0.0660105501879809,0.00267652225571724,
2.0299108331587E-5));
#49296=CARTESIAN_POINT('',(-0.0685379243677287,0.00280576092286691,-0.00103890261335452));
#49297=CARTESIAN_POINT('Ctrl Pts',(-0.0685379243677287,0.00280576092286691,
-0.00103890261335452));
#49298=CARTESIAN_POINT('Ctrl Pts',(-0.0682626321295755,0.00286788646427859,
-0.00129688101678024));
#49299=CARTESIAN_POINT('Ctrl Pts',(-0.067495495107767,0.0029887431080821,
-0.0015800602489539));
#49300=CARTESIAN_POINT('Ctrl Pts',(-0.0667281321296702,0.00286638278580766,
-0.00129361981432716));
#49301=CARTESIAN_POINT('Ctrl Pts',(-0.0664522715406983,0.00280353121836822,
-0.00102962802751535));
#49302=CARTESIAN_POINT('',(-0.0689894472304209,0.00267652109012544,-1.86561674233391E-5));
#49303=CARTESIAN_POINT('Ctrl Pts',(-0.0689894472304209,0.00267652109012544,
-1.86561674233391E-5));
#49304=CARTESIAN_POINT('Ctrl Pts',(-0.0689840520567293,0.0026785573557361,
-0.000395630752060009));
#49305=CARTESIAN_POINT('Ctrl Pts',(-0.0688168919200026,0.00274251464423593,
-0.000775051359101532));
#49306=CARTESIAN_POINT('Ctrl Pts',(-0.068540990422318,0.00280506900251843,
-0.00103602939079997));
#49307=CARTESIAN_POINT('Ctrl Pts',(-0.0685379243677287,0.00280576092286691,
-0.00103890261335452));
#49308=CARTESIAN_POINT('',(-0.0685484173841136,0.00280336755518862,0.0010289747883925));
#49309=CARTESIAN_POINT('Ctrl Pts',(-0.0685484173841136,0.00280336755518862,
0.00102897478839251));
#49310=CARTESIAN_POINT('Ctrl Pts',(-0.0688243561640007,0.00274048389401599,
0.00076509868961228));
#49311=CARTESIAN_POINT('Ctrl Pts',(-0.0689924898026455,0.00267538673953038,
0.000376229036000899));
#49312=CARTESIAN_POINT('Ctrl Pts',(-0.0689895325382811,0.00267648889292995,
-1.26954890464299E-5));
#49313=CARTESIAN_POINT('Ctrl Pts',(-0.0689894472304209,0.00267652109012544,
-1.86561674233391E-5));
#49314=CARTESIAN_POINT('Ctrl Pts',(-0.067521969610817,0.00292787381968359,
0.00143750579808091));
#49315=CARTESIAN_POINT('Ctrl Pts',(-0.0679007709531672,0.00292557966528535,
0.00143215706955923));
#49316=CARTESIAN_POINT('Ctrl Pts',(-0.0682777117231937,0.00286505864139897,
0.00128784653433001));
#49317=CARTESIAN_POINT('Ctrl Pts',(-0.0685484173841136,0.00280336755518862,
0.0010289747883925));
#49318=CARTESIAN_POINT('Ctrl Pts',(-0.087521969753009,0.00292791234232007,
0.0014375007351075));
#49319=CARTESIAN_POINT('Ctrl Pts',(-0.0875217905822522,0.00272283848633951,
0.00149851530284683));
#49320=CARTESIAN_POINT('Ctrl Pts',(-0.0875249292449862,0.00279751942631424,
0.00169899223914137));
#49321=CARTESIAN_POINT('Ctrl Pts',(-0.0871359306861318,0.00292980295225596,
0.00144284563795755));
#49322=CARTESIAN_POINT('Ctrl Pts',(-0.087128303332053,0.00272468023725732,
0.00150425289890676));
#49323=CARTESIAN_POINT('Ctrl Pts',(-0.0870869890419856,0.0027997547128407,
0.00170530652254619));
#49324=CARTESIAN_POINT('Ctrl Pts',(-0.0863597555989418,0.00281040271795959,
0.00116400921661838));
#49325=CARTESIAN_POINT('Ctrl Pts',(-0.0863911712050714,0.00262787967136625,
0.00125349479954789));
#49326=CARTESIAN_POINT('Ctrl Pts',(-0.0862058670420218,0.0026583834282292,
0.00137542120560275));
#49327=CARTESIAN_POINT('Ctrl Pts',(-0.0858448108046749,0.00261243102946704,
2.73686784603756E-5));
#49328=CARTESIAN_POINT('Ctrl Pts',(-0.0858094820998151,0.00243981891809831,
3.02504277462256E-5));
#49329=CARTESIAN_POINT('Ctrl Pts',(-0.0856221070083461,0.00242419343546418,
3.23331464451119E-5));
#49330=CARTESIAN_POINT('Ctrl Pts',(-0.0863246614268507,0.00279922894991229,
-0.00113315917795547));
#49331=CARTESIAN_POINT('Ctrl Pts',(-0.0863534248332843,0.00261785874660288,
-0.00122287857653878));
#49332=CARTESIAN_POINT('Ctrl Pts',(-0.0861660653383145,0.00264516117224188,
-0.00133894667362542));
#49333=CARTESIAN_POINT('Ctrl Pts',(-0.0874756675609659,0.00298937709191257,
-0.00158152248003427));
#49334=CARTESIAN_POINT('Ctrl Pts',(-0.0874776982153359,0.00277625525457783,
-0.00163733766341943));
#49335=CARTESIAN_POINT('Ctrl Pts',(-0.0874723735075982,0.00287024649410694,
-0.00186926883315248));
#49336=CARTESIAN_POINT('Ctrl Pts',(-0.0886390883124264,0.00281072577948571,
-0.00116572585728214));
#49337=CARTESIAN_POINT('Ctrl Pts',(-0.088607647449207,0.00262816948297619,
-0.00125530022942588));
#49338=CARTESIAN_POINT('Ctrl Pts',(-0.0887928212048197,0.00265876571215967,
-0.00137744992107541));
#49339=CARTESIAN_POINT('Ctrl Pts',(-0.0891553277660854,0.00261238743571347,
-2.56552014422575E-5));
#49340=CARTESIAN_POINT('Ctrl Pts',(-0.0891906502037131,0.00243978444592521,
-2.85609443699477E-5));
#49341=CARTESIAN_POINT('Ctrl Pts',(-0.0893780503329556,0.00242414178609795,
-3.030669215365E-5));
#49342=CARTESIAN_POINT('Ctrl Pts',(-0.0886760035727276,0.00279905892909023,
0.0011319394640289));
#49343=CARTESIAN_POINT('Ctrl Pts',(-0.0886472257773982,0.0026177065043695,
0.00122160652879803));
#49344=CARTESIAN_POINT('Ctrl Pts',(-0.0888346894846697,0.00264495997721763,
0.00133750508047797));
#49345=CARTESIAN_POINT('Ctrl Pts',(-0.0879080088854605,0.00292602173206304,
0.00143215583134954));
#49346=CARTESIAN_POINT('Ctrl Pts',(-0.0879147483545036,0.00272099921368876,
0.00149278542731808));
#49347=CARTESIAN_POINT('Ctrl Pts',(-0.0879628751525175,0.00279528411067136,
0.00169267787348782));
#49348=CARTESIAN_POINT('Ctrl Pts',(-0.087521969753009,0.00292791234232007,
0.0014375007351075));
#49349=CARTESIAN_POINT('Ctrl Pts',(-0.0875217905822522,0.00272283848633951,
0.00149851530284683));
#49350=CARTESIAN_POINT('Ctrl Pts',(-0.0875249292449862,0.00279751942631424,
0.00169899223914137));
#49351=CARTESIAN_POINT('',(-0.0875248989283422,0.00279679729590145,0.00169705696579711));
#49352=CARTESIAN_POINT('',(-0.087521969610817,0.00292787381968359,0.00143750579808091));
#49353=CARTESIAN_POINT('Ctrl Pts',(-0.087524898940367,0.00279680839753089,
0.00169705296016689));
#49354=CARTESIAN_POINT('Ctrl Pts',(-0.0875217930237306,0.00272496362417165,
0.00149792539327892));
#49355=CARTESIAN_POINT('Ctrl Pts',(-0.087521969720935,0.00292787557066265,
0.00143751167942811));
#49356=CARTESIAN_POINT('',(-0.0875,0.002796875,0.00169723753033423));
#49357=CARTESIAN_POINT('Ctrl Pts',(-0.0875,0.002796875,0.00169723753033423));
#49358=CARTESIAN_POINT('Ctrl Pts',(-0.0870556118872741,0.00279685666170104,
0.00169708273941661));
#49359=CARTESIAN_POINT('Ctrl Pts',(-0.0861665719179776,0.00264539629297987,
0.00133451307288424));
#49360=CARTESIAN_POINT('Ctrl Pts',(-0.0856341151866447,0.00242721165967408,
2.04143110301139E-6));
#49361=CARTESIAN_POINT('Ctrl Pts',(-0.0861678030184114,0.00264575759329887,
-0.00133706644457989));
#49362=CARTESIAN_POINT('Ctrl Pts',(-0.0875004674124815,0.00287245605236691,
-0.00187753708326946));
#49363=CARTESIAN_POINT('Ctrl Pts',(-0.0888323000379284,0.00264566812967151,
-0.00133621021713016));
#49364=CARTESIAN_POINT('Ctrl Pts',(-0.0893659912919883,0.00242720638772113,
8.03570479923811E-8));
#49365=CARTESIAN_POINT('Ctrl Pts',(-0.0888362194957707,0.00264414723702811,
0.00132712816164589));
#49366=CARTESIAN_POINT('Ctrl Pts',(-0.0879609366490351,0.00279406634542388,
0.00169058598422319));
#49367=CARTESIAN_POINT('Ctrl Pts',(-0.0875248989283412,0.00279679729590146,
0.00169705696579712));
#49368=CARTESIAN_POINT('',(-0.0875,0.00292794117647059,0.00143766002569487));
#49369=CARTESIAN_POINT('Ctrl Pts',(-0.0874999999943631,0.00279686254156731,
0.00169724202650596));
#49370=CARTESIAN_POINT('Ctrl Pts',(-0.0874994195756651,0.00272498843318775,
0.00149808548501933));
#49371=CARTESIAN_POINT('Ctrl Pts',(-0.0875000000046905,0.00292793913822137,
0.00143765318065731));
#49372=CARTESIAN_POINT('',(-0.0864613877374919,0.00280559596990716,0.00103824715833728));
#49373=CARTESIAN_POINT('Ctrl Pts',(-0.0864613877374919,0.00280559596990716,
0.00103824715833728));
#49374=CARTESIAN_POINT('Ctrl Pts',(-0.0867365913194384,0.0028677273296309,
0.00129598001878093));
#49375=CARTESIAN_POINT('Ctrl Pts',(-0.0871182158646947,0.0029279629632896,
0.00143762672627057));
#49376=CARTESIAN_POINT('Ctrl Pts',(-0.0875,0.00292794117647059,0.00143766002569487));
#49377=CARTESIAN_POINT('',(-0.0860105501879809,0.00267652225571725,2.02991083332626E-5));
#49378=CARTESIAN_POINT('Ctrl Pts',(-0.0860105501879809,0.00267652225571725,
2.02991083332626E-5));
#49379=CARTESIAN_POINT('Ctrl Pts',(-0.0860158709169047,0.00267857452642669,
0.000396779691602501));
#49380=CARTESIAN_POINT('Ctrl Pts',(-0.0861825726657915,0.00274235049501113,
0.000774645398476271));
#49381=CARTESIAN_POINT('Ctrl Pts',(-0.0864582351392805,0.00280488422330797,
0.00103529469620327));
#49382=CARTESIAN_POINT('Ctrl Pts',(-0.0864613877374919,0.00280559596990716,
0.00103824715833728));
#49383=CARTESIAN_POINT('',(-0.0864522715406982,0.00280353121836822,-0.00102962802751535));
#49384=CARTESIAN_POINT('Ctrl Pts',(-0.0864522715406982,0.00280353121836822,
-0.00102962802751535));
#49385=CARTESIAN_POINT('Ctrl Pts',(-0.0861764109517263,0.00274067965092877,
-0.000765636240703536));
#49386=CARTESIAN_POINT('Ctrl Pts',(-0.0860077424451036,0.00267543025507489,
-0.000375293469168902));
#49387=CARTESIAN_POINT('Ctrl Pts',(-0.0860104603923367,0.00267648762043081,
1.39454081207884E-5));
#49388=CARTESIAN_POINT('Ctrl Pts',(-0.0860105501879809,0.00267652225571725,
2.02991083332626E-5));
#49389=CARTESIAN_POINT('',(-0.0885379243677292,0.00280576092286681,-0.00103890261335415));
#49390=CARTESIAN_POINT('Ctrl Pts',(-0.0885379243677291,0.00280576092286681,
-0.00103890261335415));
#49391=CARTESIAN_POINT('Ctrl Pts',(-0.0882626321295759,0.00286788646427853,
-0.0012968810167801));
#49392=CARTESIAN_POINT('Ctrl Pts',(-0.0874954951077672,0.00298874310808213,
-0.00158006024895397));
#49393=CARTESIAN_POINT('Ctrl Pts',(-0.0867281321296702,0.00286638278580766,
-0.00129361981432716));
#49394=CARTESIAN_POINT('Ctrl Pts',(-0.0864522715406982,0.00280353121836822,
-0.00102962802751535));
#49395=CARTESIAN_POINT('',(-0.0889894472304209,0.00267652109012543,-1.86561674220561E-5));
#49396=CARTESIAN_POINT('Ctrl Pts',(-0.0889894472304209,0.00267652109012543,
-1.86561674220561E-5));
#49397=CARTESIAN_POINT('Ctrl Pts',(-0.0889840520567296,0.00267855735573596,
-0.000395630752059159));
#49398=CARTESIAN_POINT('Ctrl Pts',(-0.088816891920003,0.00274251464423583,
-0.000775051359101059));
#49399=CARTESIAN_POINT('Ctrl Pts',(-0.0885409904223183,0.00280506900251837,
-0.00103602939079972));
#49400=CARTESIAN_POINT('Ctrl Pts',(-0.0885379243677291,0.00280576092286681,
-0.00103890261335415));
#49401=CARTESIAN_POINT('',(-0.0885484173841136,0.00280336755518862,0.0010289747883925));
#49402=CARTESIAN_POINT('Ctrl Pts',(-0.0885484173841136,0.00280336755518862,
0.0010289747883925));
#49403=CARTESIAN_POINT('Ctrl Pts',(-0.0888243561640007,0.00274048389401599,
0.000765098689612275));
#49404=CARTESIAN_POINT('Ctrl Pts',(-0.0889924898026453,0.00267538673953045,
0.000376229036001328));
#49405=CARTESIAN_POINT('Ctrl Pts',(-0.0889895325382811,0.00267648889292995,
-1.26954890455724E-5));
#49406=CARTESIAN_POINT('Ctrl Pts',(-0.0889894472304209,0.00267652109012543,
-1.86561674220561E-5));
#49407=CARTESIAN_POINT('Ctrl Pts',(-0.087521969610817,0.00292787381968359,
0.00143750579808091));
#49408=CARTESIAN_POINT('Ctrl Pts',(-0.0879007709531672,0.00292557966528534,
0.00143215706955922));
#49409=CARTESIAN_POINT('Ctrl Pts',(-0.0882777117231937,0.00286505864139897,
0.00128784653433));
#49410=CARTESIAN_POINT('Ctrl Pts',(-0.0885484173841136,0.00280336755518862,
0.0010289747883925));
#49411=CARTESIAN_POINT('Ctrl Pts',(-0.107521969753009,0.00292791234232008,
0.0014375007351075));
#49412=CARTESIAN_POINT('Ctrl Pts',(-0.107521790582252,0.00272283848633961,
0.00149851530284679));
#49413=CARTESIAN_POINT('Ctrl Pts',(-0.107524929244986,0.00279751942631421,
0.00169899223914127));
#49414=CARTESIAN_POINT('Ctrl Pts',(-0.107135930686132,0.00292980295225595,
0.00144284563795752));
#49415=CARTESIAN_POINT('Ctrl Pts',(-0.107128303332053,0.00272468023725742,
0.00150425289890669));
#49416=CARTESIAN_POINT('Ctrl Pts',(-0.107086989041985,0.00279975471284066,
0.00170530652254606));
#49417=CARTESIAN_POINT('Ctrl Pts',(-0.106359755598941,0.00281040271795956,
0.00116400921661828));
#49418=CARTESIAN_POINT('Ctrl Pts',(-0.106391171205071,0.00262787967136631,
0.00125349479954775));
#49419=CARTESIAN_POINT('Ctrl Pts',(-0.106205867042022,0.00265838342822915,
0.00137542120560257));
#49420=CARTESIAN_POINT('Ctrl Pts',(-0.105844810804675,0.00261243102946704,
2.73686784602542E-5));
#49421=CARTESIAN_POINT('Ctrl Pts',(-0.105809482099816,0.00243981891809839,
3.02504277460862E-5));
#49422=CARTESIAN_POINT('Ctrl Pts',(-0.105622107008346,0.00242419343546419,
3.23331464449678E-5));
#49423=CARTESIAN_POINT('Ctrl Pts',(-0.106324661426851,0.00279922894991231,
-0.00113315917795554));
#49424=CARTESIAN_POINT('Ctrl Pts',(-0.106353424833284,0.002617858746603,
-0.00122287857653881));
#49425=CARTESIAN_POINT('Ctrl Pts',(-0.106166065338315,0.0026451611722419,
-0.00133894667362546));
#49426=CARTESIAN_POINT('Ctrl Pts',(-0.107475667560966,0.00298937709191257,
-0.00158152248003427));
#49427=CARTESIAN_POINT('Ctrl Pts',(-0.107477698215336,0.00277625525457795,
-0.00163733766341938));
#49428=CARTESIAN_POINT('Ctrl Pts',(-0.107472373507598,0.0028702464941069,
-0.00186926883315237));
#49429=CARTESIAN_POINT('Ctrl Pts',(-0.108639088312426,0.00281072577948568,
-0.00116572585728207));
#49430=CARTESIAN_POINT('Ctrl Pts',(-0.108607647449207,0.00262816948297624,
-0.00125530022942576));
#49431=CARTESIAN_POINT('Ctrl Pts',(-0.10879282120482,0.00265876571215962,
-0.00137744992107526));
#49432=CARTESIAN_POINT('Ctrl Pts',(-0.109155327766085,0.00261238743571347,
-2.5655201442127E-5));
#49433=CARTESIAN_POINT('Ctrl Pts',(-0.109190650203713,0.00243978444592529,
-2.85609443698138E-5));
#49434=CARTESIAN_POINT('Ctrl Pts',(-0.109378050332955,0.00242414178609796,
-3.0306692153495E-5));
#49435=CARTESIAN_POINT('Ctrl Pts',(-0.108676003572727,0.00279905892909026,
0.00113193946402899));
#49436=CARTESIAN_POINT('Ctrl Pts',(-0.108647225777398,0.0026177065043696,
0.00122160652879808));
#49437=CARTESIAN_POINT('Ctrl Pts',(-0.108834689484669,0.00264495997721766,
0.00133750508047803));
#49438=CARTESIAN_POINT('Ctrl Pts',(-0.107908008885461,0.00292602173206305,
0.00143215583134956));
#49439=CARTESIAN_POINT('Ctrl Pts',(-0.107914748354504,0.00272099921368888,
0.00149278542731809));
#49440=CARTESIAN_POINT('Ctrl Pts',(-0.107962875152517,0.00279528411067133,
0.00169267787348776));
#49441=CARTESIAN_POINT('Ctrl Pts',(-0.107521969753009,0.00292791234232008,
0.0014375007351075));
#49442=CARTESIAN_POINT('Ctrl Pts',(-0.107521790582252,0.00272283848633961,
0.00149851530284679));
#49443=CARTESIAN_POINT('Ctrl Pts',(-0.107524929244986,0.00279751942631421,
0.00169899223914127));
#49444=CARTESIAN_POINT('',(-0.107524898928342,0.00279679729590145,0.00169705696579711));
#49445=CARTESIAN_POINT('',(-0.107521969610817,0.00292787381968359,0.00143750579808091));
#49446=CARTESIAN_POINT('Ctrl Pts',(-0.107524898940367,0.0027968083975309,
0.00169705296016689));
#49447=CARTESIAN_POINT('Ctrl Pts',(-0.107521793023731,0.00272496362417165,
0.00149792539327893));
#49448=CARTESIAN_POINT('Ctrl Pts',(-0.107521969720935,0.00292787557066265,
0.00143751167942811));
#49449=CARTESIAN_POINT('',(-0.1075,0.002796875,0.00169723753033423));
#49450=CARTESIAN_POINT('Ctrl Pts',(-0.1075,0.002796875,0.00169723753033422));
#49451=CARTESIAN_POINT('Ctrl Pts',(-0.107055611887274,0.00279685666170103,
0.00169708273941661));
#49452=CARTESIAN_POINT('Ctrl Pts',(-0.106166571917978,0.00264539629297986,
0.00133451307288423));
#49453=CARTESIAN_POINT('Ctrl Pts',(-0.105634115186645,0.00242721165967408,
2.04143110301389E-6));
#49454=CARTESIAN_POINT('Ctrl Pts',(-0.106167803018411,0.00264575759329888,
-0.00133706644457991));
#49455=CARTESIAN_POINT('Ctrl Pts',(-0.107500467412482,0.00287245605236691,
-0.00187753708326945));
#49456=CARTESIAN_POINT('Ctrl Pts',(-0.108832300037928,0.00264566812967151,
-0.00133621021713017));
#49457=CARTESIAN_POINT('Ctrl Pts',(-0.109365991291988,0.00242720638772112,
8.03570480027352E-8));
#49458=CARTESIAN_POINT('Ctrl Pts',(-0.108836219495771,0.00264414723702813,
0.00132712816164603));
#49459=CARTESIAN_POINT('Ctrl Pts',(-0.107960936649035,0.00279406634542393,
0.00169058598422331));
#49460=CARTESIAN_POINT('Ctrl Pts',(-0.107524898928341,0.00279679729590146,
0.00169705696579713));
#49461=CARTESIAN_POINT('',(-0.1075,0.00292794117647059,0.00143766002569487));
#49462=CARTESIAN_POINT('Ctrl Pts',(-0.107499999994363,0.00279686254156731,
0.00169724202650596));
#49463=CARTESIAN_POINT('Ctrl Pts',(-0.107499419575665,0.00272498843318775,
0.00149808548501934));
#49464=CARTESIAN_POINT('Ctrl Pts',(-0.10750000000469,0.00292793913822137,
0.00143765318065731));
#49465=CARTESIAN_POINT('',(-0.106461387737498,0.0028055959699086,0.00103824715834326));
#49466=CARTESIAN_POINT('Ctrl Pts',(-0.106461387737498,0.0028055959699086,
0.00103824715834326));
#49467=CARTESIAN_POINT('Ctrl Pts',(-0.106736591319444,0.00286772732963183,
0.00129598001878312));
#49468=CARTESIAN_POINT('Ctrl Pts',(-0.107118215864697,0.0029279629632896,
0.00143762672627057));
#49469=CARTESIAN_POINT('Ctrl Pts',(-0.1075,0.00292794117647059,0.00143766002569487));
#49470=CARTESIAN_POINT('',(-0.106010550187981,0.00267652225571722,2.02991083284823E-5));
#49471=CARTESIAN_POINT('Ctrl Pts',(-0.106010550187981,0.00267652225571722,
2.02991083284823E-5));
#49472=CARTESIAN_POINT('Ctrl Pts',(-0.106015870916903,0.00267857452642615,
0.000396779691599338));
#49473=CARTESIAN_POINT('Ctrl Pts',(-0.106182572665792,0.00274235049501136,
0.000774645398478084));
#49474=CARTESIAN_POINT('Ctrl Pts',(-0.106458235139285,0.00280488422330894,
0.00103529469620727));
#49475=CARTESIAN_POINT('Ctrl Pts',(-0.106461387737498,0.0028055959699086,
0.00103824715834326));
#49476=CARTESIAN_POINT('',(-0.106452271540698,0.00280353121836822,-0.00102962802751534));
#49477=CARTESIAN_POINT('Ctrl Pts',(-0.106452271540698,0.00280353121836822,
-0.00102962802751534));
#49478=CARTESIAN_POINT('Ctrl Pts',(-0.106176410951726,0.00274067965092877,
-0.000765636240703531));
#49479=CARTESIAN_POINT('Ctrl Pts',(-0.106007742445104,0.00267543025507516,
-0.000375293469170498));
#49480=CARTESIAN_POINT('Ctrl Pts',(-0.106010460392337,0.0026764876204308,
1.39454081176005E-5));
#49481=CARTESIAN_POINT('Ctrl Pts',(-0.106010550187981,0.00267652225571722,
2.02991083284823E-5));
#49482=CARTESIAN_POINT('',(-0.108537924367725,0.00280576092286767,-0.0010389026133577));
#49483=CARTESIAN_POINT('Ctrl Pts',(-0.108537924367725,0.00280576092286767,
-0.0010389026133577));
#49484=CARTESIAN_POINT('Ctrl Pts',(-0.108262632129572,0.00286788646427908,
-0.0012968810167814));
#49485=CARTESIAN_POINT('Ctrl Pts',(-0.107495495107766,0.00298874310808185,
-0.00158006024895331));
#49486=CARTESIAN_POINT('Ctrl Pts',(-0.10672813212967,0.00286638278580766,
-0.00129361981432716));
#49487=CARTESIAN_POINT('Ctrl Pts',(-0.106452271540698,0.00280353121836822,
-0.00102962802751534));
#49488=CARTESIAN_POINT('',(-0.108989447230421,0.00267652109012545,-1.86561674248701E-5));
#49489=CARTESIAN_POINT('Ctrl Pts',(-0.108989447230421,0.00267652109012544,
-1.86561674248702E-5));
#49490=CARTESIAN_POINT('Ctrl Pts',(-0.108984052056729,0.00267855735573627,
-0.000395630752061024));
#49491=CARTESIAN_POINT('Ctrl Pts',(-0.108816891920001,0.00274251464423628,
-0.000775051359103429));
#49492=CARTESIAN_POINT('Ctrl Pts',(-0.108540990422316,0.00280506900251894,
-0.0010360293908021));
#49493=CARTESIAN_POINT('Ctrl Pts',(-0.108537924367725,0.00280576092286767,
-0.0010389026133577));
#49494=CARTESIAN_POINT('',(-0.108548417384113,0.00280336755518862,0.0010289747883925));
#49495=CARTESIAN_POINT('Ctrl Pts',(-0.108548417384113,0.00280336755518862,
0.0010289747883925));
#49496=CARTESIAN_POINT('Ctrl Pts',(-0.108824356164,0.00274048389401599,
0.000765098689612275));
#49497=CARTESIAN_POINT('Ctrl Pts',(-0.108992489802645,0.00267538673953029,
0.000376229036000389));
#49498=CARTESIAN_POINT('Ctrl Pts',(-0.108989532538281,0.00267648889292995,
-1.26954890474506E-5));
#49499=CARTESIAN_POINT('Ctrl Pts',(-0.108989447230421,0.00267652109012544,
-1.86561674248702E-5));
#49500=CARTESIAN_POINT('Ctrl Pts',(-0.107521969610817,0.00292787381968359,
0.0014375057980809));
#49501=CARTESIAN_POINT('Ctrl Pts',(-0.107900770953167,0.00292557966528534,
0.00143215706955921));
#49502=CARTESIAN_POINT('Ctrl Pts',(-0.108277711723193,0.00286505864139896,
0.00128784653432998));
#49503=CARTESIAN_POINT('Ctrl Pts',(-0.108548417384113,0.00280336755518862,
0.0010289747883925));
#49504=CARTESIAN_POINT('Ctrl Pts',(-0.127521969753009,0.00292791234232007,
0.0014375007351075));
#49505=CARTESIAN_POINT('Ctrl Pts',(-0.127521790582252,0.0027228384863398,
0.00149851530284674));
#49506=CARTESIAN_POINT('Ctrl Pts',(-0.127524929244986,0.00279751942631414,
0.0016989922391411));
#49507=CARTESIAN_POINT('Ctrl Pts',(-0.127135930686132,0.00292980295225595,
0.00144284563795753));
#49508=CARTESIAN_POINT('Ctrl Pts',(-0.127128303332053,0.00272468023725761,
0.00150425289890664));
#49509=CARTESIAN_POINT('Ctrl Pts',(-0.127086989041986,0.00279975471284059,
0.00170530652254589));
#49510=CARTESIAN_POINT('Ctrl Pts',(-0.126359755598941,0.00281040271795957,
0.00116400921661829));
#49511=CARTESIAN_POINT('Ctrl Pts',(-0.126391171205071,0.00262787967136648,
0.00125349479954768));
#49512=CARTESIAN_POINT('Ctrl Pts',(-0.126205867042022,0.00265838342822912,
0.00137542120560247));
#49513=CARTESIAN_POINT('Ctrl Pts',(-0.125844810804675,0.00261243102946704,
2.73686784602689E-5));
#49514=CARTESIAN_POINT('Ctrl Pts',(-0.125809482099816,0.00243981891809853,
3.02504277461029E-5));
#49515=CARTESIAN_POINT('Ctrl Pts',(-0.125622107008347,0.00242419343546421,
3.23331464449823E-5));
#49516=CARTESIAN_POINT('Ctrl Pts',(-0.126324661426851,0.00279922894991231,
-0.00113315917795553));
#49517=CARTESIAN_POINT('Ctrl Pts',(-0.126353424833284,0.00261785874660316,
-0.00122287857653872));
#49518=CARTESIAN_POINT('Ctrl Pts',(-0.126166065338315,0.00264516117224187,
-0.00133894667362534));
#49519=CARTESIAN_POINT('Ctrl Pts',(-0.127475667560966,0.00298937709191257,
-0.00158152248003426));
#49520=CARTESIAN_POINT('Ctrl Pts',(-0.127477698215336,0.00277625525457815,
-0.00163733766341933));
#49521=CARTESIAN_POINT('Ctrl Pts',(-0.127472373507598,0.00287024649410682,
-0.00186926883315216));
#49522=CARTESIAN_POINT('Ctrl Pts',(-0.128639088312426,0.00281072577948569,
-0.0011657258572821));
#49523=CARTESIAN_POINT('Ctrl Pts',(-0.128607647449207,0.00262816948297644,
-0.00125530022942571));
#49524=CARTESIAN_POINT('Ctrl Pts',(-0.12879282120482,0.00265876571215961,
-0.00137744992107518));
#49525=CARTESIAN_POINT('Ctrl Pts',(-0.129155327766085,0.00261238743571346,
-2.56552014421315E-5));
#49526=CARTESIAN_POINT('Ctrl Pts',(-0.129190650203713,0.00243978444592542,
-2.85609443698061E-5));
#49527=CARTESIAN_POINT('Ctrl Pts',(-0.129378050332955,0.00242414178609797,
-3.03066921534991E-5));
#49528=CARTESIAN_POINT('Ctrl Pts',(-0.128676003572727,0.00279905892909026,
0.00113193946402897));
#49529=CARTESIAN_POINT('Ctrl Pts',(-0.128647225777398,0.00261770650436977,
0.00122160652879797));
#49530=CARTESIAN_POINT('Ctrl Pts',(-0.12883468948467,0.00264495997721762,
0.00133750508047789));
#49531=CARTESIAN_POINT('Ctrl Pts',(-0.127908008885461,0.00292602173206305,
0.00143215583134956));
#49532=CARTESIAN_POINT('Ctrl Pts',(-0.127914748354504,0.00272099921368907,
0.00149278542731802));
#49533=CARTESIAN_POINT('Ctrl Pts',(-0.127962875152517,0.00279528411067127,
0.00169267787348758));
#49534=CARTESIAN_POINT('Ctrl Pts',(-0.127521969753009,0.00292791234232007,
0.0014375007351075));
#49535=CARTESIAN_POINT('Ctrl Pts',(-0.127521790582252,0.0027228384863398,
0.00149851530284674));
#49536=CARTESIAN_POINT('Ctrl Pts',(-0.127524929244986,0.00279751942631414,
0.0016989922391411));
#49537=CARTESIAN_POINT('',(-0.127524898928342,0.00279679729590145,0.00169705696579711));
#49538=CARTESIAN_POINT('',(-0.127521969610817,0.00292787381968359,0.0014375057980809));
#49539=CARTESIAN_POINT('Ctrl Pts',(-0.127524898940367,0.0027968083975309,
0.00169705296016689));
#49540=CARTESIAN_POINT('Ctrl Pts',(-0.127521793023731,0.00272496362417165,
0.00149792539327892));
#49541=CARTESIAN_POINT('Ctrl Pts',(-0.127521969720935,0.00292787557066265,
0.00143751167942811));
#49542=CARTESIAN_POINT('',(-0.1275,0.002796875,0.00169723753033423));
#49543=CARTESIAN_POINT('Ctrl Pts',(-0.1275,0.002796875,0.00169723753033422));
#49544=CARTESIAN_POINT('Ctrl Pts',(-0.127055611887274,0.00279685666170104,
0.00169708273941661));
#49545=CARTESIAN_POINT('Ctrl Pts',(-0.126166571917978,0.00264539629297987,
0.00133451307288423));
#49546=CARTESIAN_POINT('Ctrl Pts',(-0.125634115186645,0.00242721165967408,
2.04143110301003E-6));
#49547=CARTESIAN_POINT('Ctrl Pts',(-0.126167803018411,0.00264575759329888,
-0.0013370664445799));
#49548=CARTESIAN_POINT('Ctrl Pts',(-0.127500467412481,0.00287245605236691,
-0.00187753708326946));
#49549=CARTESIAN_POINT('Ctrl Pts',(-0.128832300037928,0.00264566812967151,
-0.00133621021713016));
#49550=CARTESIAN_POINT('Ctrl Pts',(-0.129365991291988,0.00242720638772113,
8.03570479970567E-8));
#49551=CARTESIAN_POINT('Ctrl Pts',(-0.128836219495771,0.00264414723702813,
0.00132712816164604));
#49552=CARTESIAN_POINT('Ctrl Pts',(-0.127960936649035,0.00279406634542393,
0.00169058598422331));
#49553=CARTESIAN_POINT('Ctrl Pts',(-0.127524898928341,0.00279679729590146,
0.00169705696579713));
#49554=CARTESIAN_POINT('',(-0.1275,0.00292794117647059,0.00143766002569487));
#49555=CARTESIAN_POINT('Ctrl Pts',(-0.127499999994363,0.00279686254156731,
0.00169724202650597));
#49556=CARTESIAN_POINT('Ctrl Pts',(-0.127499419575665,0.00272498843318775,
0.00149808548501933));
#49557=CARTESIAN_POINT('Ctrl Pts',(-0.12750000000469,0.00292793913822137,
0.00143765318065731));
#49558=CARTESIAN_POINT('',(-0.126461387737499,0.0028055959699088,0.00103824715834409));
#49559=CARTESIAN_POINT('Ctrl Pts',(-0.126461387737499,0.0028055959699088,
0.00103824715834409));
#49560=CARTESIAN_POINT('Ctrl Pts',(-0.126736591319445,0.00286772732963196,
0.00129598001878342));
#49561=CARTESIAN_POINT('Ctrl Pts',(-0.127118215864698,0.0029279629632896,
0.00143762672627057));
#49562=CARTESIAN_POINT('Ctrl Pts',(-0.1275,0.00292794117647059,0.00143766002569487));
#49563=CARTESIAN_POINT('',(-0.126010550187981,0.00267652225571722,2.02991083269042E-5));
#49564=CARTESIAN_POINT('Ctrl Pts',(-0.126010550187981,0.00267652225571722,
2.02991083269042E-5));
#49565=CARTESIAN_POINT('Ctrl Pts',(-0.126015870916903,0.00267857452642598,
0.000396779691598294));
#49566=CARTESIAN_POINT('Ctrl Pts',(-0.126182572665792,0.00274235049501134,
0.000774645398478129));
#49567=CARTESIAN_POINT('Ctrl Pts',(-0.126458235139285,0.00280488422330907,
0.00103529469620783));
#49568=CARTESIAN_POINT('Ctrl Pts',(-0.126461387737499,0.0028055959699088,
0.00103824715834409));
#49569=CARTESIAN_POINT('',(-0.126452271540698,0.00280353121836822,-0.00102962802751534));
#49570=CARTESIAN_POINT('Ctrl Pts',(-0.126452271540698,0.00280353121836822,
-0.00102962802751534));
#49571=CARTESIAN_POINT('Ctrl Pts',(-0.126176410951726,0.00274067965092877,
-0.000765636240703523));
#49572=CARTESIAN_POINT('Ctrl Pts',(-0.126007742445104,0.00267543025507525,
-0.000375293469171025));
#49573=CARTESIAN_POINT('Ctrl Pts',(-0.126010460392337,0.00267648762043079,
1.39454081165485E-5));
#49574=CARTESIAN_POINT('Ctrl Pts',(-0.126010550187981,0.00267652225571722,
2.02991083269042E-5));
#49575=CARTESIAN_POINT('',(-0.128537924367724,0.00280576092286786,-0.00103890261335849));
#49576=CARTESIAN_POINT('Ctrl Pts',(-0.128537924367724,0.00280576092286786,
-0.00103890261335849));
#49577=CARTESIAN_POINT('Ctrl Pts',(-0.128262632129572,0.0028678864642792,
-0.00129688101678168));
#49578=CARTESIAN_POINT('Ctrl Pts',(-0.127495495107765,0.00298874310808179,
-0.00158006024895316));
#49579=CARTESIAN_POINT('Ctrl Pts',(-0.12672813212967,0.00286638278580766,
-0.00129361981432715));
#49580=CARTESIAN_POINT('Ctrl Pts',(-0.126452271540698,0.00280353121836822,
-0.00102962802751534));
#49581=CARTESIAN_POINT('',(-0.128989447230421,0.00267652109012544,-1.86561674238163E-5));
#49582=CARTESIAN_POINT('Ctrl Pts',(-0.128989447230421,0.00267652109012544,
-1.86561674238163E-5));
#49583=CARTESIAN_POINT('Ctrl Pts',(-0.128984052056729,0.00267855735573615,
-0.000395630752060325));
#49584=CARTESIAN_POINT('Ctrl Pts',(-0.128816891920002,0.00274251464423628,
-0.000775051359103574));
#49585=CARTESIAN_POINT('Ctrl Pts',(-0.128540990422315,0.00280506900251906,
-0.00103602939080263));
#49586=CARTESIAN_POINT('Ctrl Pts',(-0.128537924367724,0.00280576092286786,
-0.00103890261335849));
#49587=CARTESIAN_POINT('',(-0.128548417384113,0.00280336755518862,0.0010289747883925));
#49588=CARTESIAN_POINT('Ctrl Pts',(-0.128548417384113,0.00280336755518862,
0.0010289747883925));
#49589=CARTESIAN_POINT('Ctrl Pts',(-0.128824356164,0.00274048389401599,
0.00076509868961228));
#49590=CARTESIAN_POINT('Ctrl Pts',(-0.128992489802645,0.00267538673953035,
0.00037622903600074));
#49591=CARTESIAN_POINT('Ctrl Pts',(-0.128989532538281,0.00267648889292995,
-1.26954890467481E-5));
#49592=CARTESIAN_POINT('Ctrl Pts',(-0.128989447230421,0.00267652109012544,
-1.86561674238163E-5));
#49593=CARTESIAN_POINT('Ctrl Pts',(-0.127521969610817,0.00292787381968359,
0.0014375057980809));
#49594=CARTESIAN_POINT('Ctrl Pts',(-0.127900770953167,0.00292557966528534,
0.00143215706955922));
#49595=CARTESIAN_POINT('Ctrl Pts',(-0.128277711723193,0.00286505864139897,
0.00128784653432999));
#49596=CARTESIAN_POINT('Ctrl Pts',(-0.128548417384113,0.00280336755518862,
0.0010289747883925));
#49597=CARTESIAN_POINT('Origin',(0.0125,0.013,-4.59242549680257E-18));
#49598=CARTESIAN_POINT('',(0.00634842519685039,0.0128,-0.0108815498639327));
#49599=CARTESIAN_POINT('',(0.00595472440944882,0.0132,-0.0106493834302149));
#49600=CARTESIAN_POINT('Ctrl Pts',(0.00634842519685039,0.0128,-0.0108815498639327));
#49601=CARTESIAN_POINT('Ctrl Pts',(0.00634842519685039,0.0130276434464512,
-0.0108815498639327));
#49602=CARTESIAN_POINT('Ctrl Pts',(0.00614779345682715,0.0132,-0.0107680466496751));
#49603=CARTESIAN_POINT('Ctrl Pts',(0.00595472440944882,0.0132,-0.0106493834302149));
#49604=CARTESIAN_POINT('',(0.00634842519685039,0.0012,-0.0108815498639328));
#49605=CARTESIAN_POINT('',(0.00634842519685039,0.013,-0.0108815498639327));
#49606=CARTESIAN_POINT('',(0.0063484251968504,0.0012,0.0108815498639327));
#49607=CARTESIAN_POINT('Origin',(0.0125,0.0012,-4.59242549680257E-18));
#49608=CARTESIAN_POINT('',(0.0063484251968504,0.0132,0.0108815498639327));
#49609=CARTESIAN_POINT('',(0.0063484251968504,0.013,0.0108815498639327));
#49610=CARTESIAN_POINT('',(0.0125,0.0132,-0.0125));
#49611=CARTESIAN_POINT('Origin',(0.0125,0.0132,-4.59242549680257E-18));
#49612=CARTESIAN_POINT('Origin',(0.0125,0.0132,-4.59242549680257E-18));
#49613=CARTESIAN_POINT('Origin',(-0.00501982557395217,0.0101715728752538,
-2.16840434497101E-19));
#49614=CARTESIAN_POINT('',(-0.00501982557395217,0.013,-0.001));
#49615=CARTESIAN_POINT('Origin',(-0.00501982557395217,0.013,-2.16840434497101E-19));
#49616=CARTESIAN_POINT('',(-0.00501982557395217,0.0132,-0.001));
#49617=CARTESIAN_POINT('',(-0.00501982557395217,0.0101715728752538,-0.001));
#49618=CARTESIAN_POINT('Origin',(-0.00501982557395217,0.0132,-2.16840434497101E-19));
#49619=CARTESIAN_POINT('Origin',(0.00396253460616978,-0.0267643850402721,
0.));
#49620=CARTESIAN_POINT('',(-0.00847413551306003,0.0128,0.00451935750764788));
#49621=CARTESIAN_POINT('',(-0.000426041560703258,0.0128,0.0124834192096569));
#49622=CARTESIAN_POINT('Origin',(0.00396253460616978,0.0128,0.));
#49623=CARTESIAN_POINT('',(-0.000426041560703258,0.0012,0.0124834192096569));
#49624=CARTESIAN_POINT('',(-0.000426041560703259,-0.0267643850402721,0.0124834192096569));
#49625=CARTESIAN_POINT('',(-0.00847413551306003,0.0012,0.00451935750764788));
#49626=CARTESIAN_POINT('Origin',(0.00396253460616978,0.0012,0.));
#49627=CARTESIAN_POINT('',(-0.00847413551306003,-0.0267643850402721,0.00451935750764788));
#49628=CARTESIAN_POINT('Origin',(0.00396253460616978,-0.0267643850402721,
0.));
#49629=CARTESIAN_POINT('',(-0.00918425288415922,0.001,-0.00150244288430738));
#49630=CARTESIAN_POINT('',(-0.00918425288415922,0.0128,-0.00150244288430738));
#49631=CARTESIAN_POINT('',(-0.00918425288415922,0.007,-0.00150244288430738));
#49632=CARTESIAN_POINT('',(-0.00918425288415922,0.0128,0.00150244288430738));
#49633=CARTESIAN_POINT('Origin',(0.00396253460616978,0.0128,0.));
#49634=CARTESIAN_POINT('',(-0.00918425288415922,0.001,0.00150244288430738));
#49635=CARTESIAN_POINT('',(-0.00918425288415922,0.007,0.00150244288430738));
#49636=CARTESIAN_POINT('Origin',(0.00396253460616978,0.001,0.));
#49637=CARTESIAN_POINT('Origin',(0.00625,0.013,-2.29621274840129E-18));
#49638=CARTESIAN_POINT('',(-0.000359710594690624,0.013,-0.0122947390492059));
#49639=CARTESIAN_POINT('',(0.00585,0.013,-0.0108197735650983));
#49640=CARTESIAN_POINT('Origin',(0.,0.013,0.));
#49641=CARTESIAN_POINT('',(0.0060484,0.013,0.0109392347739684));
#49642=CARTESIAN_POINT('Origin',(0.0125,0.013,-4.59242549680257E-18));
#49643=CARTESIAN_POINT('',(0.000266151447280837,0.013,0.0124971662150709));
#49644=CARTESIAN_POINT('Origin',(0.,0.013,0.));
#49645=CARTESIAN_POINT('',(-0.00828616193994173,0.013,0.00445104985208033));
#49646=CARTESIAN_POINT('Origin',(0.00396253460616978,0.013,0.));
#49647=CARTESIAN_POINT('',(-0.00880510120094866,0.013,0.00421409688951767));
#49648=CARTESIAN_POINT('Origin',(-0.00866210908617835,0.013,0.00458766516321543));
#49649=CARTESIAN_POINT('',(-0.00895326315945259,0.013,0.00173913195070769));
#49650=CARTESIAN_POINT('Origin',(-0.00926982557395217,0.013,0.003));
#49651=CARTESIAN_POINT('',(-0.00895326315945259,0.013,-0.00173913195070769));
#49652=CARTESIAN_POINT('Origin',(0.00396253460616978,0.013,0.));
#49653=CARTESIAN_POINT('',(-0.00880510120094866,0.013,-0.00421409688951767));
#49654=CARTESIAN_POINT('Origin',(-0.00926982557395217,0.013,-0.003));
#49655=CARTESIAN_POINT('',(-0.00828616193994173,0.013,-0.00445104985208033));
#49656=CARTESIAN_POINT('Origin',(-0.00866210908617835,0.013,-0.00458766516321543));
#49657=CARTESIAN_POINT('Origin',(0.00396253460616978,0.013,0.));
#49658=CARTESIAN_POINT('',(0.,0.013,0.0115));
#49659=CARTESIAN_POINT('Origin',(0.,0.013,0.011));
#49660=CARTESIAN_POINT('',(0.,0.013,-0.0105));
#49661=CARTESIAN_POINT('Origin',(0.,0.013,-0.011));
#49662=CARTESIAN_POINT('',(-0.00926982557395217,0.013,-0.0025));
#49663=CARTESIAN_POINT('Origin',(-0.00926982557395217,0.013,-0.003));
#49664=CARTESIAN_POINT('',(-0.00926982557395217,0.013,0.0035));
#49665=CARTESIAN_POINT('Origin',(-0.00926982557395217,0.013,0.003));
#49666=CARTESIAN_POINT('Origin',(0.,0.013,0.));
#49667=CARTESIAN_POINT('',(0.00615157480314961,0.0130279409847639,0.0108815498639327));
#49668=CARTESIAN_POINT('Ctrl Pts',(0.00604840000000001,0.013,0.0109392347739684));
#49669=CARTESIAN_POINT('Ctrl Pts',(0.00605844545062544,0.013,0.0109336805551571));
#49670=CARTESIAN_POINT('Ctrl Pts',(0.00606848366139432,0.0130007331928852,
0.0109281121725045));
#49671=CARTESIAN_POINT('Ctrl Pts',(0.0061039365412421,0.0130059660120152,
0.0109083825874413));
#49672=CARTESIAN_POINT('Ctrl Pts',(0.00612881666876444,0.0130145598482818,
0.0108944155280892));
#49673=CARTESIAN_POINT('Ctrl Pts',(0.00615157480314961,0.013027940984764,
0.0108815498639328));
#49674=CARTESIAN_POINT('',(0.00615157480314961,0.0012,0.0108815498639327));
#49675=CARTESIAN_POINT('',(0.00615157480314961,0.013,0.0108815498639327));
#49676=CARTESIAN_POINT('',(-0.000365559547449821,0.0012,0.0124946535052905));
#49677=CARTESIAN_POINT('Origin',(0.,0.0012,0.));
#49678=CARTESIAN_POINT('',(-0.000365559547449821,0.0128603449921863,0.0124946535052905));
#49679=CARTESIAN_POINT('',(-0.000365559547449821,0.013,0.0124946535052905));
#49680=CARTESIAN_POINT('Ctrl Pts',(-0.000365559547449479,0.0128603449921859,
0.0124946535052905));
#49681=CARTESIAN_POINT('Ctrl Pts',(-0.000355817464249198,0.0128695697559461,
0.0124949385321241));
#49682=CARTESIAN_POINT('Ctrl Pts',(-0.00034473067538757,0.0128777448000062,
0.0124952504075834));
#49683=CARTESIAN_POINT('Ctrl Pts',(-0.000293723387019724,0.012910410477147,
0.0124966125421717));
#49684=CARTESIAN_POINT('Ctrl Pts',(-0.000243928646755985,0.0129282527769246,
0.012497667010507));
#49685=CARTESIAN_POINT('Ctrl Pts',(-0.000103079663471278,0.0129721021830651,
0.012500028589373));
#49686=CARTESIAN_POINT('Ctrl Pts',(3.8406604879568E-5,0.0129933569155071,
0.0125008701719831));
#49687=CARTESIAN_POINT('Ctrl Pts',(0.000215988889848001,0.0129995665030976,
0.0124981591951788));
#49688=CARTESIAN_POINT('Ctrl Pts',(0.000241141730008187,0.013,0.0124976988456156));
#49689=CARTESIAN_POINT('Ctrl Pts',(0.000266151447280838,0.013,0.0124971662150709));
#49690=CARTESIAN_POINT('Origin',(0.,0.013,0.));
#49691=CARTESIAN_POINT('',(-0.000365559547449821,0.0012,-0.0124946535052905));
#49692=CARTESIAN_POINT('',(0.0061515748031496,0.0012,-0.0108815498639327));
#49693=CARTESIAN_POINT('Origin',(0.,0.0012,0.));
#49694=CARTESIAN_POINT('',(0.0061515748031496,0.0128,-0.0108815498639327));
#49695=CARTESIAN_POINT('',(0.0061515748031496,0.013,-0.0108815498639328));
#49696=CARTESIAN_POINT('',(-0.00036555954744982,0.0128,-0.0124946535052905));
#49697=CARTESIAN_POINT('Origin',(0.,0.0128,0.));
#49698=CARTESIAN_POINT('',(-0.00036555954744982,0.013,-0.0124946535052905));
#49699=CARTESIAN_POINT('Origin',(-0.14,0.0075,0.));
#49700=CARTESIAN_POINT('',(-0.0399999969037804,0.00997686116634681,-0.00434340405242746));
#49701=CARTESIAN_POINT('',(-0.0399999963113939,0.00997613772986841,0.00434381651807744));
#49702=CARTESIAN_POINT('Ctrl Pts',(-0.04,0.00997615395078692,0.0043438072715076));
#49703=CARTESIAN_POINT('Ctrl Pts',(-0.04,0.0107382262196358,0.00390939383155763));
#49704=CARTESIAN_POINT('Ctrl Pts',(-0.04,0.0113831176353465,0.00327045662389616));
#49705=CARTESIAN_POINT('Ctrl Pts',(-0.04,0.0118237356861523,0.00251236616753416));
#49706=CARTESIAN_POINT('Ctrl Pts',(-0.04,0.0122643368146118,0.00175430482634162));
#49707=CARTESIAN_POINT('Ctrl Pts',(-0.04,0.012500474596807,0.000877315234985374));
#49708=CARTESIAN_POINT('Ctrl Pts',(-0.04,0.0125005474735341,4.15581768158591E-7));
#49709=CARTESIAN_POINT('Ctrl Pts',(-0.04,0.0125006203502613,-0.000876484072272305));
#49710=CARTESIAN_POINT('Ctrl Pts',(-0.04,0.0122646283392576,-0.00175351290185706));
#49711=CARTESIAN_POINT('Ctrl Pts',(-0.04,0.0118241532168882,-0.00251164746737131));
#49712=CARTESIAN_POINT('Ctrl Pts',(-0.04,0.0113836611778392,-0.00326981114944385));
#49713=CARTESIAN_POINT('Ctrl Pts',(-0.04,0.0107388759723705,-0.00390885553816552));
#49714=CARTESIAN_POINT('Ctrl Pts',(-0.04,0.00997687591821936,-0.00434339564002003));
#49715=CARTESIAN_POINT('',(-0.04,0.0075,-0.005));
#49716=CARTESIAN_POINT('Origin',(-0.04,0.00750000000000001,7.7715611723761E-18));
#49717=CARTESIAN_POINT('',(-0.0399999990786921,0.00503252942117453,-0.00434874567463202));
#49718=CARTESIAN_POINT('Origin',(-0.04,0.00750000000000002,-4.9960036108132E-18));
#49719=CARTESIAN_POINT('',(-0.0399999989166323,0.00503323066735753,0.00434914348573771));
#49720=CARTESIAN_POINT('Ctrl Pts',(-0.04,0.00503252942117453,-0.00434874567463202));
#49721=CARTESIAN_POINT('Ctrl Pts',(-0.04,0.00426802397510403,-0.00391496664116614));
#49722=CARTESIAN_POINT('Ctrl Pts',(-0.04,0.00362078375203728,-0.00327557207983672));
#49723=CARTESIAN_POINT('Ctrl Pts',(-0.04,0.00317856541491556,-0.00251633280931734));
#49724=CARTESIAN_POINT('Ctrl Pts',(-0.04,0.00273636410682584,-0.00175712277573535));
#49725=CARTESIAN_POINT('Ctrl Pts',(-0.04,0.00249937673440971,-0.000878295009110667));
#49726=CARTESIAN_POINT('Ctrl Pts',(-0.04,0.00249944757726906,4.03157137211354E-7));
#49727=CARTESIAN_POINT('Ctrl Pts',(-0.04,0.00249951842012842,0.000879101323554153));
#49728=CARTESIAN_POINT('Ctrl Pts',(-0.04,0.00273664749617628,0.00175789086588404));
#49729=CARTESIAN_POINT('Ctrl Pts',(-0.04,0.00317897121753076,0.00251702958693044));
#49730=CARTESIAN_POINT('Ctrl Pts',(-0.04,0.00362131197246112,0.00327619754187586));
#49731=CARTESIAN_POINT('Ctrl Pts',(-0.04,0.0042686552861704,0.00391548773053193));
#49732=CARTESIAN_POINT('Ctrl Pts',(-0.04,0.00503323066735754,0.0043491434857377));
#49733=CARTESIAN_POINT('',(-0.04,0.0075,0.005));
#49734=CARTESIAN_POINT('Origin',(-0.04,0.0075,0.));
#49735=CARTESIAN_POINT('',(-0.139,0.0075,0.005));
#49736=CARTESIAN_POINT('',(-0.14,0.0075,0.005));
#49737=CARTESIAN_POINT('',(-0.139,0.0075,-0.005));
#49738=CARTESIAN_POINT('Origin',(-0.139,0.0075,0.));
#49739=CARTESIAN_POINT('Origin',(-0.139,0.0075,0.));
#49740=CARTESIAN_POINT('Origin',(-0.04,0.0075,0.));
#49741=CARTESIAN_POINT('Ctrl Pts',(-0.127524898928341,0.00279679729590146,
0.00169705696579713));
#49742=CARTESIAN_POINT('Ctrl Pts',(-0.127516599909907,0.00279684927353385,
0.00169718012669082));
#49743=CARTESIAN_POINT('Ctrl Pts',(-0.127508299977955,0.00279687534251024,
0.00169724042141337));
#49744=CARTESIAN_POINT('Ctrl Pts',(-0.1275,0.002796875,0.00169723753033422));
#49745=CARTESIAN_POINT('Ctrl Pts',(-0.107524898928341,0.00279679729590146,
0.00169705696579713));
#49746=CARTESIAN_POINT('Ctrl Pts',(-0.107516599909907,0.00279684927353385,
0.00169718012669082));
#49747=CARTESIAN_POINT('Ctrl Pts',(-0.107508299977955,0.00279687534251023,
0.00169724042141337));
#49748=CARTESIAN_POINT('Ctrl Pts',(-0.1075,0.002796875,0.00169723753033422));
#49749=CARTESIAN_POINT('Ctrl Pts',(-0.0875248989283412,0.00279679729590146,
0.00169705696579712));
#49750=CARTESIAN_POINT('Ctrl Pts',(-0.0875165999099073,0.00279684927353385,
0.00169718012669082));
#49751=CARTESIAN_POINT('Ctrl Pts',(-0.0875082999779549,0.00279687534251024,
0.00169724042141337));
#49752=CARTESIAN_POINT('Ctrl Pts',(-0.0875,0.002796875,0.00169723753033423));
#49753=CARTESIAN_POINT('Ctrl Pts',(-0.0675248989283412,0.00279679729590146,
0.00169705696579713));
#49754=CARTESIAN_POINT('Ctrl Pts',(-0.0675165999099073,0.00279684927353385,
0.00169718012669082));
#49755=CARTESIAN_POINT('Ctrl Pts',(-0.0675082999779549,0.00279687534251024,
0.00169724042141337));
#49756=CARTESIAN_POINT('Ctrl Pts',(-0.0675,0.002796875,0.00169723753033423));
#49757=CARTESIAN_POINT('Ctrl Pts',(-0.0475248989283412,0.00279679729590146,
0.00169705696579713));
#49758=CARTESIAN_POINT('Ctrl Pts',(-0.0475165999099073,0.00279684927353385,
0.00169718012669083));
#49759=CARTESIAN_POINT('Ctrl Pts',(-0.0475082999779549,0.00279687534251024,
0.00169724042141337));
#49760=CARTESIAN_POINT('Ctrl Pts',(-0.0475,0.002796875,0.00169723753033423));
#49761=CARTESIAN_POINT('Origin',(0.,0.015,0.));
#49762=CARTESIAN_POINT('',(-5.65991084816151E-17,0.0148,-0.0165));
#49763=CARTESIAN_POINT('',(-5.65991084816151E-17,0.0002,-0.0165));
#49764=CARTESIAN_POINT('',(-5.65991084816151E-17,0.015,-0.0165));
#49765=CARTESIAN_POINT('',(-0.00839639405880103,0.0002,-0.0142038926639612));
#49766=CARTESIAN_POINT('Origin',(0.,0.0002,0.));
#49767=CARTESIAN_POINT('',(-0.00839639405880103,0.0148,-0.0142038926639612));
#49768=CARTESIAN_POINT('',(-0.00839639405880103,0.015,-0.0142038926639612));
#49769=CARTESIAN_POINT('Origin',(0.,0.0148,0.));
#49770=CARTESIAN_POINT('Origin',(-5.76094420909117E-17,0.015,-0.0165));
#49771=CARTESIAN_POINT('',(0.0125,0.0148,-0.0165));
#49772=CARTESIAN_POINT('',(0.0125,0.0002,-0.0165));
#49773=CARTESIAN_POINT('',(0.0125,0.015,-0.0165));
#49774=CARTESIAN_POINT('',(-5.73013858584659E-17,0.0002,-0.0165));
#49775=CARTESIAN_POINT('',(-5.76094420909117E-17,0.0148,-0.0165));
#49776=CARTESIAN_POINT('Origin',(0.,0.015,0.));
#49777=CARTESIAN_POINT('',(-0.00839639405880104,0.0148,0.0142038926639612));
#49778=CARTESIAN_POINT('',(-0.00839639405880104,0.0002,0.0142038926639612));
#49779=CARTESIAN_POINT('',(-0.00839639405880104,0.015,0.0142038926639612));
#49780=CARTESIAN_POINT('',(0.,0.0002,0.0165));
#49781=CARTESIAN_POINT('Origin',(0.,0.0002,0.));
#49782=CARTESIAN_POINT('',(0.,0.0148,0.0165));
#49783=CARTESIAN_POINT('',(0.,0.015,0.0165));
#49784=CARTESIAN_POINT('Origin',(0.,0.0148,0.));
#49785=CARTESIAN_POINT('Origin',(1.72828326272735E-16,0.015,0.0165));
#49786=CARTESIAN_POINT('',(0.0125000000000002,0.0002,0.0165));
#49787=CARTESIAN_POINT('',(1.72828326272735E-16,0.0002,0.0165));
#49788=CARTESIAN_POINT('',(0.0125000000000002,0.0148,0.0165));
#49789=CARTESIAN_POINT('',(0.0125000000000002,0.015,0.0165));
#49790=CARTESIAN_POINT('',(5.55111512312575E-20,0.0148,0.0165));
#49791=CARTESIAN_POINT('Origin',(0.0125,0.015,-4.59242549680257E-18));
#49792=CARTESIAN_POINT('Origin',(0.0125,0.0002,-4.59242549680257E-18));
#49793=CARTESIAN_POINT('Origin',(0.0125,0.0148,-4.59242549680257E-18));
#49794=CARTESIAN_POINT('Origin',(0.0125,0.015,-4.59242549680257E-18));
#49795=CARTESIAN_POINT('',(-0.0166089107357434,0.015,-0.00911686983553521));
#49796=CARTESIAN_POINT('',(-0.00376723863546634,0.015,-0.00239186662703728));
#49797=CARTESIAN_POINT('',(-0.00376723863546634,0.015,-0.00239186662703728));
#49798=CARTESIAN_POINT('',(-0.00376723863546634,0.015,0.00239186662703728));
#49799=CARTESIAN_POINT('Origin',(-0.00501982557395217,0.015,-2.16840434497101E-19));
#49800=CARTESIAN_POINT('',(-0.0166089107357433,0.015,0.00911686983553521));
#49801=CARTESIAN_POINT('',(-0.0169270413562866,0.015,0.00928347037066553));
#49802=CARTESIAN_POINT('',(-0.00829461958536103,0.015,0.0140317242680344));
#49803=CARTESIAN_POINT('',(-0.00829461958536103,0.015,0.0140317242680344));
#49804=CARTESIAN_POINT('',(-5.55111512312578E-20,0.015,0.0163));
#49805=CARTESIAN_POINT('Origin',(0.,0.015,0.));
#49806=CARTESIAN_POINT('',(0.0125000000000002,0.015,0.0163));
#49807=CARTESIAN_POINT('',(0.0125000000000002,0.015,0.0163));
#49808=CARTESIAN_POINT('',(0.0125,0.015,-0.0163));
#49809=CARTESIAN_POINT('Origin',(0.0125,0.015,-4.59242549680257E-18));
#49810=CARTESIAN_POINT('',(-5.5913058681838E-17,0.015,-0.0163));
#49811=CARTESIAN_POINT('',(0.0125,0.015,-0.0163));
#49812=CARTESIAN_POINT('',(-0.00829461958536102,0.015,-0.0140317242680344));
#49813=CARTESIAN_POINT('Origin',(0.,0.015,0.));
#49814=CARTESIAN_POINT('',(-0.0169180511005122,0.015,-0.00893412666903227));
#49815=CARTESIAN_POINT('',(0.,0.015,0.0115));
#49816=CARTESIAN_POINT('Origin',(0.,0.015,0.011));
#49817=CARTESIAN_POINT('',(0.,0.015,-0.0105));
#49818=CARTESIAN_POINT('Origin',(0.,0.015,-0.011));
#49819=CARTESIAN_POINT('',(0.0125,0.015,-0.0092));
#49820=CARTESIAN_POINT('Origin',(0.0125,0.015,-4.59242549680257E-18));
#49821=CARTESIAN_POINT('Origin',(0.0125,0.,-4.59242549680257E-18));
#49822=CARTESIAN_POINT('',(-0.0306415078475588,-1.19605085394936E-7,-0.000938136006279154));
#49823=CARTESIAN_POINT('',(-0.0206310823726759,0.,-0.00685120104972884));
#49824=CARTESIAN_POINT('Ctrl Pts',(-0.03064150786828,6.06630742267791E-51,
-0.000938136151692983));
#49825=CARTESIAN_POINT('Ctrl Pts',(-0.0289673468934464,7.16790888657192E-28,
-0.00191390121462454));
#49826=CARTESIAN_POINT('Ctrl Pts',(-0.0272875529435704,-1.0309211203299E-17,
-0.00288012983552212));
#49827=CARTESIAN_POINT('Ctrl Pts',(-0.0256190528013343,1.02955830966733E-17,
-0.00386547850042675));
#49828=CARTESIAN_POINT('Ctrl Pts',(-0.0239505526590982,3.09003774046027E-17,
-0.00485082716533138));
#49829=CARTESIAN_POINT('Ctrl Pts',(-0.022293347014245,1.90239552262182E-25,
-0.00585529628600419));
#49830=CARTESIAN_POINT('Ctrl Pts',(-0.0206310823726766,-1.73472347597923E-20,
-0.0068512010497298));
#49831=CARTESIAN_POINT('',(-0.018277353250021,3.08514507815582E-8,-0.00813059850575379));
#49832=CARTESIAN_POINT('Ctrl Pts',(-0.0206310823726745,0.,-0.00685120104972968));
#49833=CARTESIAN_POINT('Ctrl Pts',(-0.0198643807345651,1.57511708648874E-27,
-0.0073105513809931));
#49834=CARTESIAN_POINT('Ctrl Pts',(-0.0190726109028725,0.,-0.0077237863538248));
#49835=CARTESIAN_POINT('Ctrl Pts',(-0.0182773531828187,0.,-0.00813059853874281));
#49836=CARTESIAN_POINT('',(-0.00829461958536102,0.,-0.0140317242680344));
#49837=CARTESIAN_POINT('',(0.00096849183839154,0.,-0.0195074579675537));
#49838=CARTESIAN_POINT('',(-5.5913058681838E-17,0.,-0.0163));
#49839=CARTESIAN_POINT('Origin',(0.,0.,0.));
#49840=CARTESIAN_POINT('',(0.0125,0.,-0.0163));
#49841=CARTESIAN_POINT('',(0.0125,0.,-0.0163));
#49842=CARTESIAN_POINT('',(0.0125000000000002,0.,0.0163));
#49843=CARTESIAN_POINT('Origin',(0.0125,0.,-4.59242549680257E-18));
#49844=CARTESIAN_POINT('',(0.,0.,0.0163));
#49845=CARTESIAN_POINT('',(0.0125,0.,0.0163));
#49846=CARTESIAN_POINT('',(-0.00829461958536103,0.,0.0140317242680344));
#49847=CARTESIAN_POINT('Origin',(0.,0.,0.));
#49848=CARTESIAN_POINT('',(-0.0183185438988578,2.99066327258402E-17,0.00810624909661309));
#49849=CARTESIAN_POINT('',(0.000968491838391539,0.,0.0195074579675537));
#49850=CARTESIAN_POINT('',(-0.0206729454446971,0.,0.0068262100906602));
#49851=CARTESIAN_POINT('Ctrl Pts',(-0.0183185440091374,0.,0.00810624927278113));
#49852=CARTESIAN_POINT('Ctrl Pts',(-0.0191139452258369,0.,0.00769907071789008));
#49853=CARTESIAN_POINT('Ctrl Pts',(-0.0199059893503628,2.20596951890412E-24,
0.00728571135373499));
#49854=CARTESIAN_POINT('Ctrl Pts',(-0.0206729454446971,6.6121838851786E-30,
0.00682621009066024));
#49855=CARTESIAN_POINT('',(-0.0306415862453137,-8.66279905141487E-8,0.000938073089450988));
#49856=CARTESIAN_POINT('Ctrl Pts',(-0.0206729454446971,-2.71050543121376E-20,
0.00682621009066024));
#49857=CARTESIAN_POINT('Ctrl Pts',(-0.0223282407769415,-2.71050543121376E-20,
0.00583448409485697));
#49858=CARTESIAN_POINT('Ctrl Pts',(-0.0239784617686096,-6.77626357803436E-21,
0.00483419474493695));
#49859=CARTESIAN_POINT('Ctrl Pts',(-0.0256400041972464,2.42311502295287E-35,
0.00385301122208682));
#49860=CARTESIAN_POINT('Ctrl Pts',(-0.0273015466258831,6.77626357803439E-21,
0.00287182769923668));
#49861=CARTESIAN_POINT('Ctrl Pts',(-0.0289744104914885,0.,0.00190975000345643));
#49862=CARTESIAN_POINT('Ctrl Pts',(-0.0306415862989849,0.,0.000938073256321053));
#49863=CARTESIAN_POINT('Ctrl Pts',(-0.0306415862453137,-8.66279905141357E-8,
0.000938073089450988));
#49864=CARTESIAN_POINT('Ctrl Pts',(-0.0308898601383488,2.57926462655969E-8,
0.000793373576933981));
#49865=CARTESIAN_POINT('Ctrl Pts',(-0.0310667270502054,1.08407425174632E-7,
0.000550378915350664));
#49866=CARTESIAN_POINT('Ctrl Pts',(-0.0311372956334381,1.45622331613657E-7,
0.00028264191180899));
#49867=CARTESIAN_POINT('Ctrl Pts',(-0.0311615868604397,1.5843250433844E-7,
0.000190481065837118));
#49868=CARTESIAN_POINT('Ctrl Pts',(-0.0311737818075073,1.66200756503995E-7,
9.53821800403144E-5));
#49869=CARTESIAN_POINT('Ctrl Pts',(-0.0311737532392636,1.64882298400146E-7,
1.60473702184294E-7));
#49870=CARTESIAN_POINT('Ctrl Pts',(-0.0311736711029301,1.61091609846496E-7,
-0.000273610707362422));
#49871=CARTESIAN_POINT('Ctrl Pts',(-0.0310696664268064,9.52873903898754E-8,
-0.000547409293633988));
#49872=CARTESIAN_POINT('Ctrl Pts',(-0.030877772516319,-5.72693113770487E-10,
-0.000750518444677997));
#49873=CARTESIAN_POINT('Ctrl Pts',(-0.0308090257338665,-3.49149621819306E-8,
-0.000823283133174159));
#49874=CARTESIAN_POINT('Ctrl Pts',(-0.0307294370403642,-7.72395171728875E-8,
-0.000886888142082073));
#49875=CARTESIAN_POINT('Ctrl Pts',(-0.0306415078475588,-1.19605085394879E-7,
-0.000938136006279154));
#49876=CARTESIAN_POINT('',(0.00625,0.,-0.0121912878729033));
#49877=CARTESIAN_POINT('',(0.00625,0.,0.0121912878729033));
#49878=CARTESIAN_POINT('Origin',(0.,0.,0.));
#49879=CARTESIAN_POINT('Origin',(0.0125,0.,-4.59242549680257E-18));
#49880=CARTESIAN_POINT('Origin',(0.,0.001,0.));
#49881=CARTESIAN_POINT('',(0.00625,0.001,0.0119660979437743));
#49882=CARTESIAN_POINT('',(0.00625,0.0002,0.0119660979437743));
#49883=CARTESIAN_POINT('',(0.00625,0.001,0.0119660979437743));
#49884=CARTESIAN_POINT('',(0.00625,0.0002,-0.0119660979437743));
#49885=CARTESIAN_POINT('Origin',(0.,0.0002,0.));
#49886=CARTESIAN_POINT('',(0.00625,0.001,-0.0119660979437743));
#49887=CARTESIAN_POINT('',(0.00625,0.001,-0.0119660979437743));
#49888=CARTESIAN_POINT('Origin',(0.,0.001,0.));
#49889=CARTESIAN_POINT('Origin',(0.0125,0.001,-4.59242549680257E-18));
#49890=CARTESIAN_POINT('Origin',(0.0125,0.0002,-4.59242549680257E-18));
#49891=CARTESIAN_POINT('Origin',(0.0125,0.001,-4.59242549680257E-18));
#49892=CARTESIAN_POINT('Origin',(0.00625,0.001,-2.29621274840129E-18));
#49893=CARTESIAN_POINT('',(-0.000371408500209017,0.001,0.0126945679613751));
#49894=CARTESIAN_POINT('',(0.00625,0.001,0.0110556546617557));
#49895=CARTESIAN_POINT('Origin',(0.,0.001,0.));
#49896=CARTESIAN_POINT('',(0.00625,0.001,-0.0110556546617557));
#49897=CARTESIAN_POINT('Origin',(0.0125,0.001,-4.59242549680257E-18));
#49898=CARTESIAN_POINT('',(-0.000371408500209017,0.001,-0.0126945679613751));
#49899=CARTESIAN_POINT('Origin',(0.,0.001,0.));
#49900=CARTESIAN_POINT('',(-0.000492372526715892,0.001,-0.0126720993701079));
#49901=CARTESIAN_POINT('Origin',(-0.000359710594690623,0.001,-0.0122947390492059));
#49902=CARTESIAN_POINT('',(-0.00872901544041542,0.001,-0.00439918826870923));
#49903=CARTESIAN_POINT('Origin',(0.00396253460616978,0.001,0.));
#49904=CARTESIAN_POINT('',(-0.0087336051435635,0.001,-0.00440088102636655));
#49905=CARTESIAN_POINT('Origin',(-0.00866210908617835,0.001,-0.00458766516321543));
#49906=CARTESIAN_POINT('Origin',(-0.00926982557395217,0.001,-0.003));
#49907=CARTESIAN_POINT('',(-0.0087336051435635,0.001,0.00440088102636655));
#49908=CARTESIAN_POINT('Origin',(-0.00926982557395217,0.001,0.003));
#49909=CARTESIAN_POINT('',(-0.00872901544041542,0.001,0.00439918826870923));
#49910=CARTESIAN_POINT('Origin',(-0.00866210908617835,0.001,0.00458766516321543));
#49911=CARTESIAN_POINT('',(-0.000492372526715893,0.001,0.0126720993701079));
#49912=CARTESIAN_POINT('Origin',(0.00396253460616978,0.001,0.));
#49913=CARTESIAN_POINT('Origin',(-0.000359710594690623,0.001,0.0122947390492058));
#49914=CARTESIAN_POINT('Origin',(0.0125,0.0134,-4.59242549680257E-18));
#49915=CARTESIAN_POINT('',(0.0125,0.0134,-0.0123));
#49916=CARTESIAN_POINT('Origin',(0.0125,0.0134,-4.59242549680257E-18));
#49917=CARTESIAN_POINT('',(0.0125,0.0134,-0.0092));
#49918=CARTESIAN_POINT('Origin',(0.0125,0.0134,-4.59242549680257E-18));
#49919=CARTESIAN_POINT('Origin',(0.0125,0.015,-4.59242549680257E-18));
#49920=CARTESIAN_POINT('',(0.0125,0.0148,0.00899999999999999));
#49921=CARTESIAN_POINT('',(0.0125,0.0148,-0.009));
#49922=CARTESIAN_POINT('Origin',(0.0125,0.0148,-4.59242549680257E-18));
#49923=CARTESIAN_POINT('Origin',(0.0125,0.0148,-4.59242549680257E-18));
#49924=CARTESIAN_POINT('',(0.0125,0.0136,0.00899999999999999));
#49925=CARTESIAN_POINT('',(0.0125,0.015,0.00899999999999999));
#49926=CARTESIAN_POINT('',(0.0125,0.0136,-0.009));
#49927=CARTESIAN_POINT('Origin',(0.0125,0.0136,-4.59242549680257E-18));
#49928=CARTESIAN_POINT('Origin',(0.0125,0.0136,-4.59242549680257E-18));
#49929=CARTESIAN_POINT('Origin',(-0.00839639405880103,0.015,0.0142038926639612));
#49930=CARTESIAN_POINT('',(-0.0171157106796651,0.0132,0.00904961418521835));
#49931=CARTESIAN_POINT('',(-0.0175612941370424,0.0132,0.00878621496200997));
#49932=CARTESIAN_POINT('',(-0.0215570023002331,0.0132,0.00642421877717253));
#49933=CARTESIAN_POINT('',(-0.0150672706217452,0.0114767391344914,0.010260629200748));
#49934=CARTESIAN_POINT('Ctrl Pts',(-0.0175612941370424,0.0132,0.00878621496200996));
#49935=CARTESIAN_POINT('Ctrl Pts',(-0.0173229778501341,0.013111161537897,
0.00892709165707185));
#49936=CARTESIAN_POINT('Ctrl Pts',(-0.0170864812350933,0.0130160222101977,
0.00906689268348295));
#49937=CARTESIAN_POINT('Ctrl Pts',(-0.0168527050452293,0.0129128930140674,
0.0092050855759598));
#49938=CARTESIAN_POINT('Ctrl Pts',(-0.0166189288553652,0.012809763817937,
0.00934327846843666));
#49939=CARTESIAN_POINT('Ctrl Pts',(-0.0163878730912532,0.0126986447513118,
0.00947986322663923));
#49940=CARTESIAN_POINT('Ctrl Pts',(-0.0161611109731713,0.0125744273552869,
0.00961390986766));
#49941=CARTESIAN_POINT('Ctrl Pts',(-0.0159343488550895,0.0124502099592619,
0.00974795650868077));
#49942=CARTESIAN_POINT('Ctrl Pts',(-0.0157118803918583,0.0123128942200067,
0.00987946502730567));
#49943=CARTESIAN_POINT('Ctrl Pts',(-0.0155076135681626,0.0121472852270145,
0.0100002139505386));
#49944=CARTESIAN_POINT('Ctrl Pts',(-0.0154054801563147,0.0120644807305183,
0.010060588412155));
#49945=CARTESIAN_POINT('Ctrl Pts',(-0.0153078971638308,0.0119746028996598,
0.0101182729693195));
#49946=CARTESIAN_POINT('Ctrl Pts',(-0.0152234095810172,0.0118644951654366,
0.0101682163936442));
#49947=CARTESIAN_POINT('Ctrl Pts',(-0.0151389219982035,0.0117543874312135,
0.0102181598179688));
#49948=CARTESIAN_POINT('Ctrl Pts',(-0.0150675299392406,0.0116240498354857,
0.0102603620419579));
#49949=CARTESIAN_POINT('Ctrl Pts',(-0.0150672200690482,0.0114767391349546,
0.0102605452165499));
#49950=CARTESIAN_POINT('',(-0.0150696760858911,0.00250000000230064,0.0102591396094456));
#49951=CARTESIAN_POINT('Ctrl Pts',(-0.0150672705003522,0.0114767391348364,
0.0102606292735785));
#49952=CARTESIAN_POINT('Ctrl Pts',(-0.0150659075926703,0.0108260833645536,
0.0102614460562153));
#49953=CARTESIAN_POINT('Ctrl Pts',(-0.0150649244414608,0.0101240231335967,
0.0102620375058781));
#49954=CARTESIAN_POINT('Ctrl Pts',(-0.0150643215473666,0.00937866249945708,
0.0102624001187059));
#49955=CARTESIAN_POINT('Ctrl Pts',(-0.0150640201003195,0.00900598218238727,
0.0102625814251198));
#49956=CARTESIAN_POINT('Ctrl Pts',(-0.0150638137327322,0.00862247676452173,
0.0102627055478026));
#49957=CARTESIAN_POINT('Ctrl Pts',(-0.0150637004162104,0.00822004218836817,
0.0102627735152981));
#49958=CARTESIAN_POINT('Ctrl Pts',(-0.0150635870996886,0.00781760761221461,
0.0102628414827935));
#49959=CARTESIAN_POINT('Ctrl Pts',(-0.015063566834431,0.00739624387777302,
0.0102628532955054));
#49960=CARTESIAN_POINT('Ctrl Pts',(-0.0150636473733159,0.00698836721501205,
0.0102628042599833));
#49961=CARTESIAN_POINT('Ctrl Pts',(-0.0150638084510857,0.00617261388949012,
0.010262706188939));
#49962=CARTESIAN_POINT('Ctrl Pts',(-0.0150643726537689,0.00541080885069056,
0.0102623645778269));
#49963=CARTESIAN_POINT('Ctrl Pts',(-0.0150653755701918,0.00466676809321675,
0.010261759642764));
#49964=CARTESIAN_POINT('Ctrl Pts',(-0.0150663784866148,0.00392272733574294,
0.0102611547077011));
#49965=CARTESIAN_POINT('Ctrl Pts',(-0.015067820129422,0.00319645085959551,
0.0102602864595939));
#49966=CARTESIAN_POINT('Ctrl Pts',(-0.0150696910491641,0.0024999999999077,
0.0102591654099954));
#49967=CARTESIAN_POINT('',(-0.0150726550660005,0.00138682640630969,0.0102573320455256));
#49968=CARTESIAN_POINT('',(-0.015069656672316,0.00249999999999522,0.0102591080098914));
#49969=CARTESIAN_POINT('',(-0.0167335787825944,0.0002,0.00927550507767659));
#49970=CARTESIAN_POINT('Ctrl Pts',(-0.0150726552252303,0.00138682640630866,
0.0102573323146958));
#49971=CARTESIAN_POINT('Ctrl Pts',(-0.0150731971649166,0.00118574953270313,
0.0102570119560962));
#49972=CARTESIAN_POINT('Ctrl Pts',(-0.0152081064597958,0.00103259595613278,
0.0101772625783165));
#49973=CARTESIAN_POINT('Ctrl Pts',(-0.0153485028614304,0.000910488615915601,
0.0100942695889684));
#49974=CARTESIAN_POINT('Ctrl Pts',(-0.0154888992630651,0.000788381275698425,
0.0100112765996203));
#49975=CARTESIAN_POINT('Ctrl Pts',(-0.0156347825636464,0.000697320245644121,
0.00992504012154639));
#49976=CARTESIAN_POINT('Ctrl Pts',(-0.0157861198041517,0.000614449925209533,
0.00983557963792288));
#49977=CARTESIAN_POINT('Ctrl Pts',(-0.0159374570446571,0.000531579604774943,
0.00974611915429937));
#49978=CARTESIAN_POINT('Ctrl Pts',(-0.0160942482158647,0.000456899963464771,
0.0096534346705775));
#49979=CARTESIAN_POINT('Ctrl Pts',(-0.0162528722771886,0.000388514508127937,
0.00955966670445773));
#49980=CARTESIAN_POINT('Ctrl Pts',(-0.0164114963385125,0.000320129052791105,
0.00946589873833796));
#49981=CARTESIAN_POINT('Ctrl Pts',(-0.0165719532869742,0.000258037776486399,
0.00937104729158102));
#49982=CARTESIAN_POINT('Ctrl Pts',(-0.01673357878255,0.000200000000015906,
0.00927550507770282));
#49983=CARTESIAN_POINT('',(-0.00839639405880103,0.0002,0.0142038926639612));
#49984=CARTESIAN_POINT('',(-0.0167106852091834,0.0148,0.009289038231462));
#49985=CARTESIAN_POINT('',(-0.0170198255739522,0.0148,0.00910629506495906));
#49986=CARTESIAN_POINT('',(-0.0167106852091834,0.0136,0.009289038231462));
#49987=CARTESIAN_POINT('',(-0.0167106852091834,0.015,0.009289038231462));
#49988=CARTESIAN_POINT('Origin',(-0.0171157106796651,0.0136,0.00904961418521835));
#49989=CARTESIAN_POINT('Origin',(-0.00839639405880103,0.015,-0.0142038926639612));
#49990=CARTESIAN_POINT('',(-0.0166926437830517,0.0002,-0.00929970311937464));
#49991=CARTESIAN_POINT('',(-0.00839639405880103,0.0002,-0.0142038926639612));
#49992=CARTESIAN_POINT('',(-0.01504752612516,0.00139784887637815,-0.0102721865570626));
#49993=CARTESIAN_POINT('Ctrl Pts',(-0.0166926437830517,0.000199999999999716,
-0.00929970311937462));
#49994=CARTESIAN_POINT('Ctrl Pts',(-0.0165313761725789,0.000258323117271339,
-0.00939503377544802));
#49995=CARTESIAN_POINT('Ctrl Pts',(-0.0163717374471408,0.00032059129430158,
-0.00948940154332222));
#49996=CARTESIAN_POINT('Ctrl Pts',(-0.0162138266410766,0.000389342010301485,
-0.00958274788050075));
#49997=CARTESIAN_POINT('Ctrl Pts',(-0.0160559158350124,0.000458092726301389,
-0.00967609421767928));
#49998=CARTESIAN_POINT('Ctrl Pts',(-0.015899732950897,0.000533325987099894,
-0.00976841912264));
#49999=CARTESIAN_POINT('Ctrl Pts',(-0.0157484005065699,0.000617287381555205,
-0.00985787677108282));
#50000=CARTESIAN_POINT('Ctrl Pts',(-0.0155970680622428,0.000701248776010517,
-0.00994733441952563));
#50001=CARTESIAN_POINT('Ctrl Pts',(-0.0154505860660156,0.000793938331462511,
-0.0100339248065372));
#50002=CARTESIAN_POINT('Ctrl Pts',(-0.0153122611083508,0.000918161762487361,
-0.0101156932963588));
#50003=CARTESIAN_POINT('Ctrl Pts',(-0.015173936150686,0.00104238519351221,
-0.0101974617861805));
#50004=CARTESIAN_POINT('Ctrl Pts',(-0.015043768415608,0.00119814242791505,
-0.0102744082700292));
#50005=CARTESIAN_POINT('Ctrl Pts',(-0.0150475263029645,0.00139784887637434,
-0.0102721868576446));
#50006=CARTESIAN_POINT('',(-0.0150682948691039,0.00250188254723652,-0.0102598985791645));
#50007=CARTESIAN_POINT('',(-0.0150475257696179,0.00139784887638291,-0.0102721859558591));
#50008=CARTESIAN_POINT('',(-0.0151696828310441,0.00750413531507349,-0.0101999796192979));
#50009=CARTESIAN_POINT('Ctrl Pts',(-0.0150682998181951,0.00250188254704829,
-0.0102599069408648));
#50010=CARTESIAN_POINT('Ctrl Pts',(-0.0150967279280264,0.00401291028492777,
-0.0102431021382563));
#50011=CARTESIAN_POINT('Ctrl Pts',(-0.0151305217455447,0.00568032787429946,
-0.0102231254871123));
#50012=CARTESIAN_POINT('Ctrl Pts',(-0.0151696812707501,0.00750413531516336,
-0.0101999769874327));
#50013=CARTESIAN_POINT('',(-0.0152584725567155,0.0114711480137007,-0.0101474887966015));
#50014=CARTESIAN_POINT('Ctrl Pts',(-0.01516968127075,0.00750413531516336,
-0.0101999769874327));
#50015=CARTESIAN_POINT('Ctrl Pts',(-0.0152015623713677,0.00898895812500316,
-0.0101811310069577));
#50016=CARTESIAN_POINT('Ctrl Pts',(-0.0152311595696551,0.0103112956911785,
-0.0101636351172226));
#50017=CARTESIAN_POINT('Ctrl Pts',(-0.0152584728656123,0.0114711480136893,
-0.0101474893182275));
#50018=CARTESIAN_POINT('',(-0.0177200739051674,0.0132,-0.00869235495241383));
#50019=CARTESIAN_POINT('Ctrl Pts',(-0.0152584728656124,0.0114711480136919,
-0.0101474893182275));
#50020=CARTESIAN_POINT('Ctrl Pts',(-0.0152619549961719,0.0116190061218255,
-0.0101454309148705));
#50021=CARTESIAN_POINT('Ctrl Pts',(-0.0153327035891074,0.0117490011390277,
-0.0101036090650828));
#50022=CARTESIAN_POINT('Ctrl Pts',(-0.0154162085456889,0.0118593137698746,
-0.0100542465038534));
#50023=CARTESIAN_POINT('Ctrl Pts',(-0.0154997135022704,0.0119696264007216,
-0.0100048839426239));
#50024=CARTESIAN_POINT('Ctrl Pts',(-0.0155959746753244,0.0120602565912413,
-0.00994798075695177));
#50025=CARTESIAN_POINT('Ctrl Pts',(-0.0156967904973433,0.0121437216331223,
-0.00988838516656967));
#50026=CARTESIAN_POINT('Ctrl Pts',(-0.0158984221413811,0.0123106517168843,
-0.00976919398580547));
#50027=CARTESIAN_POINT('Ctrl Pts',(-0.0161182723237525,0.0124489213294069,
-0.00963923322020681));
#50028=CARTESIAN_POINT('Ctrl Pts',(-0.0163414673925833,0.0125735141295264,
-0.0095072951808101));
#50029=CARTESIAN_POINT('Ctrl Pts',(-0.0165646624614141,0.0126981069296459,
-0.0093753571414134));
#50030=CARTESIAN_POINT('Ctrl Pts',(-0.0167912024035204,0.0128090229374379,
-0.00924144183601202));
#50031=CARTESIAN_POINT('Ctrl Pts',(-0.017021176870325,0.012912202521094,
-0.00910549626866394));
#50032=CARTESIAN_POINT('Ctrl Pts',(-0.0172511513371295,0.0130153821047501,
-0.00896955070131585));
#50033=CARTESIAN_POINT('Ctrl Pts',(-0.0174845603276081,0.0131108252678533,
-0.00883157487262645));
#50034=CARTESIAN_POINT('Ctrl Pts',(-0.017720073905168,0.0132,-0.00869235495241341));
#50035=CARTESIAN_POINT('',(-0.0171157106796651,0.0132,-0.00904961418521835));
#50036=CARTESIAN_POINT('',(-0.0170198255739522,0.0132,-0.00910629506495906));
#50037=CARTESIAN_POINT('',(-0.0167106852091834,0.0136,-0.00928903823146201));
#50038=CARTESIAN_POINT('Origin',(-0.0171157106796651,0.0136,-0.00904961418521834));
#50039=CARTESIAN_POINT('',(-0.0167106852091834,0.0148,-0.00928903823146201));
#50040=CARTESIAN_POINT('',(-0.0167106852091834,0.015,-0.00928903823146201));
#50041=CARTESIAN_POINT('',(-0.00839639405880103,0.0148,-0.0142038926639612));
#50042=CARTESIAN_POINT('Ctrl Pts',(-0.04,0.00503323066735754,0.0043491434857377));
#50043=CARTESIAN_POINT('Ctrl Pts',(-0.0373335531119965,0.00503323066735754,
0.0043491434857377));
#50044=CARTESIAN_POINT('Ctrl Pts',(-0.0349552522444544,0.00493945518810382,
0.0044470975219459));
#50045=CARTESIAN_POINT('Ctrl Pts',(-0.0327211769482695,0.00477742014678961,
0.00468135238095731));
#50046=CARTESIAN_POINT('Ctrl Pts',(-0.04,0.00426866982654043,0.00391549597761299));
#50047=CARTESIAN_POINT('Ctrl Pts',(-0.037357541268117,0.00426866982654043,
0.00391549597761299));
#50048=CARTESIAN_POINT('Ctrl Pts',(-0.0349933516210969,0.00420319701705448,
0.00397919554166179));
#50049=CARTESIAN_POINT('Ctrl Pts',(-0.032766245054209,0.00409006624844954,
0.00414731897802562));
#50050=CARTESIAN_POINT('Ctrl Pts',(-0.04,0.00297384830823641,0.00263671750932495));
#50051=CARTESIAN_POINT('Ctrl Pts',(-0.0374055174496866,0.00297384830823641,
0.00263671750932495));
#50052=CARTESIAN_POINT('Ctrl Pts',(-0.0350694792794186,0.00295630750671264,
0.00265761922721007));
#50053=CARTESIAN_POINT('Ctrl Pts',(-0.0328562262229028,0.00292599858475061,
0.00273220367477735));
#50054=CARTESIAN_POINT('Ctrl Pts',(-0.04,0.00226235348654652,4.2227252587527E-7));
#50055=CARTESIAN_POINT('Ctrl Pts',(-0.0374076766156412,0.00226235348654652,
4.2227252587527E-7));
#50056=CARTESIAN_POINT('Ctrl Pts',(-0.0350724447670342,0.00227115110622434,
-5.69710842301547E-7));
#50057=CARTESIAN_POINT('Ctrl Pts',(-0.0328592699289883,0.00228635233847694,
-1.75243967904944E-6));
#50058=CARTESIAN_POINT('Ctrl Pts',(-0.04,0.00297342320919197,-0.00263598765508364));
#50059=CARTESIAN_POINT('Ctrl Pts',(-0.0374055078715638,0.00297342320919197,
-0.00263598765508364));
#50060=CARTESIAN_POINT('Ctrl Pts',(-0.0350685208298449,0.00295589853021904,
-0.00265886669139246));
#50061=CARTESIAN_POINT('Ctrl Pts',(-0.0328541484702436,0.00292561725632549,
-0.0027358064165028));
#50062=CARTESIAN_POINT('Ctrl Pts',(-0.04,0.00426803851384994,-0.00391497489042477));
#50063=CARTESIAN_POINT('Ctrl Pts',(-0.0373575346994387,0.00426803851384994,
-0.00391497489042477));
#50064=CARTESIAN_POINT('Ctrl Pts',(-0.034991910923473,0.00420258965996815,
-0.00398063923938531));
#50065=CARTESIAN_POINT('Ctrl Pts',(-0.03276310942731,0.00408949996568061,
-0.00415109891161779));
#50066=CARTESIAN_POINT('Ctrl Pts',(-0.04,0.00503252942117453,-0.00434874567463202));
#50067=CARTESIAN_POINT('Ctrl Pts',(-0.037333548178702,0.00503252942117453,
-0.00434874567463202));
#50068=CARTESIAN_POINT('Ctrl Pts',(-0.034953641512335,0.00493878055701564,
-0.00444865672873833));
#50069=CARTESIAN_POINT('Ctrl Pts',(-0.032717667415586,0.00477679114689861,
-0.00468523614631841));
#50070=CARTESIAN_POINT('',(-0.0327968762032639,0.00420554807594454,-0.00417120478069329));
#50071=CARTESIAN_POINT('Ctrl Pts',(-0.0327968795935294,0.00420555000362145,
-0.00417120625622339));
#50072=CARTESIAN_POINT('Ctrl Pts',(-0.0336175849861136,0.00434997248243195,
-0.00420475803964206));
#50073=CARTESIAN_POINT('Ctrl Pts',(-0.0344378865182222,0.0044959788927343,
-0.00423892428362857));
#50074=CARTESIAN_POINT('Ctrl Pts',(-0.0352615686182026,0.00462509266287838,
-0.00426736268617292));
#50075=CARTESIAN_POINT('Ctrl Pts',(-0.0360317364760486,0.00474581797155349,
-0.00429395345895852));
#50076=CARTESIAN_POINT('Ctrl Pts',(-0.0368048362410686,0.00485177839771797,
-0.00431592424605144));
#50077=CARTESIAN_POINT('Ctrl Pts',(-0.0375815336438874,0.00492019429147787,
-0.0043277496851657));
#50078=CARTESIAN_POINT('Ctrl Pts',(-0.0383853608252005,0.00499099992934722,
-0.00433998818288245));
#50079=CARTESIAN_POINT('Ctrl Pts',(-0.0391930521783087,0.00502105452742686,
-0.00434223485095487));
#50080=CARTESIAN_POINT('Ctrl Pts',(-0.0399999990786921,0.00503252942117453,
-0.00434874567463202));
#50081=CARTESIAN_POINT('',(-0.0364391610694964,0.00340557668880199,-0.00293086975220478));
#50082=CARTESIAN_POINT('Ctrl Pts',(-0.0327968763819142,0.00420554873112458,
-0.00417120302188662));
#50083=CARTESIAN_POINT('Ctrl Pts',(-0.0328215632400491,0.00420048893979486,
-0.00416276786668299));
#50084=CARTESIAN_POINT('Ctrl Pts',(-0.0328462592609637,0.00419541111203618,
-0.00415433766263343));
#50085=CARTESIAN_POINT('Ctrl Pts',(-0.0328709631528736,0.00419031601120015,
-0.00414591186122784));
#50086=CARTESIAN_POINT('Ctrl Pts',(-0.0330092657588975,0.00416179152905996,
-0.00409874073950808));
#50087=CARTESIAN_POINT('Ctrl Pts',(-0.0331477652015767,0.00413273014284505,
-0.00405173072279408));
#50088=CARTESIAN_POINT('Ctrl Pts',(-0.0332860718111478,0.00410328863811645,
-0.00400491481922219));
#50089=CARTESIAN_POINT('Ctrl Pts',(-0.0334147601364774,0.00407589458984604,
-0.00396135464340599));
#50090=CARTESIAN_POINT('Ctrl Pts',(-0.0335432958668976,0.00404817007233707,
-0.00391795487705723));
#50091=CARTESIAN_POINT('Ctrl Pts',(-0.0336714989161663,0.00402023339740768,
-0.00387471114131506));
#50092=CARTESIAN_POINT('Ctrl Pts',(-0.0336837720381774,0.00401755896632395,
-0.00387057133615437));
#50093=CARTESIAN_POINT('Ctrl Pts',(-0.0336960424060585,0.00401488256503795,
-0.00386643283303635));
#50094=CARTESIAN_POINT('Ctrl Pts',(-0.0337083098547249,0.00401220430028142,
-0.00386229565129054));
#50095=CARTESIAN_POINT('Ctrl Pts',(-0.0338164503700708,0.00398859475123179,
-0.00382582539751267));
#50096=CARTESIAN_POINT('Ctrl Pts',(-0.0339242916194723,0.00396485019215915,
-0.00378947774226141));
#50097=CARTESIAN_POINT('Ctrl Pts',(-0.0340330956396721,0.00394073017346232,
-0.00375277414638576));
#50098=CARTESIAN_POINT('Ctrl Pts',(-0.0340765868380846,0.00393108890729467,
-0.00373810296633425));
#50099=CARTESIAN_POINT('Ctrl Pts',(-0.0341202308469956,0.00392138799822184,
-0.00372337504059853));
#50100=CARTESIAN_POINT('Ctrl Pts',(-0.0341640923441276,0.00391161467659147,
-0.00370856653712364));
#50101=CARTESIAN_POINT('Ctrl Pts',(-0.0343176842555536,0.00387739096676982,
-0.00365671088916841));
#50102=CARTESIAN_POINT('Ctrl Pts',(-0.0344740450561803,0.00384224880621381,
-0.00360383719676782));
#50103=CARTESIAN_POINT('Ctrl Pts',(-0.0346199413654582,0.00380932113143792,
-0.00355433783745459));
#50104=CARTESIAN_POINT('Ctrl Pts',(-0.0346472426152604,0.00380315944935759,
-0.00354507513313842));
#50105=CARTESIAN_POINT('Ctrl Pts',(-0.0346741609330305,0.00379707968931115,
-0.0035359367135654));
#50106=CARTESIAN_POINT('Ctrl Pts',(-0.0347008875072039,0.00379104028287026,
-0.00352685777939867));
#50107=CARTESIAN_POINT('Ctrl Pts',(-0.0348169862087886,0.00376480544852224,
-0.00348741941136502));
#50108=CARTESIAN_POINT('Ctrl Pts',(-0.0349296502264305,0.00373928845294353,
-0.00344904799014247));
#50109=CARTESIAN_POINT('Ctrl Pts',(-0.0350527857045229,0.00371144178408232,
-0.00340701244398427));
#50110=CARTESIAN_POINT('Ctrl Pts',(-0.0351285266834232,0.00369431321974542,
-0.00338115626131496));
#50111=CARTESIAN_POINT('Ctrl Pts',(-0.0352082756719269,0.00367630004581376,
-0.00335389864567627));
#50112=CARTESIAN_POINT('Ctrl Pts',(-0.0352855219259208,0.00365889457268727,
-0.00332745545077473));
#50113=CARTESIAN_POINT('Ctrl Pts',(-0.0352950361946265,0.00365675077490146,
-0.00332419849462838));
#50114=CARTESIAN_POINT('Ctrl Pts',(-0.0353045108873918,0.00365461653476455,
-0.00332095448530997));
#50115=CARTESIAN_POINT('Ctrl Pts',(-0.0353140452347724,0.00365246957958181,
-0.00331768947106946));
#50116=CARTESIAN_POINT('Ctrl Pts',(-0.0353432155236711,0.003645900980764,
-0.00330770017606563));
#50117=CARTESIAN_POINT('Ctrl Pts',(-0.035372952324594,0.00363921098688231,
-0.00329751177977544));
#50118=CARTESIAN_POINT('Ctrl Pts',(-0.0354060246459562,0.00363178204943183,
-0.00328617448683469));
#50119=CARTESIAN_POINT('Ctrl Pts',(-0.0354499066991535,0.00362192495398237,
-0.00327113158475073));
#50120=CARTESIAN_POINT('Ctrl Pts',(-0.0354996695841126,0.003610770528947,
-0.00325405419777999));
#50121=CARTESIAN_POINT('Ctrl Pts',(-0.0355293049097754,0.00360413703833009,
-0.00324387808159859));
#50122=CARTESIAN_POINT('Ctrl Pts',(-0.0355589402354383,0.00359750354771319,
-0.00323370196541719));
#50123=CARTESIAN_POINT('Ctrl Pts',(-0.035568441838183,0.00359537779213524,
-0.00323043241565654));
#50124=CARTESIAN_POINT('Ctrl Pts',(-0.0355865697128671,0.00359132226877824,
-0.00322419580591136));
#50125=CARTESIAN_POINT('Ctrl Pts',(-0.0356046975875512,0.00358726674542124,
-0.00321795919616619));
#50126=CARTESIAN_POINT('Ctrl Pts',(-0.0356314515535437,0.00358128594405739,
-0.00320875208760797));
#50127=CARTESIAN_POINT('Ctrl Pts',(-0.0356598137894403,0.00357495996564327,
-0.00319898802663048));
#50128=CARTESIAN_POINT('Ctrl Pts',(-0.0357165382612333,0.00356230800881504,
-0.0031794599046755));
#50129=CARTESIAN_POINT('Ctrl Pts',(-0.0357796961244657,0.00354826678936026,
-0.00315771038066871));
#50130=CARTESIAN_POINT('Ctrl Pts',(-0.0358544927611633,0.00353177085984188,
-0.00313195953803351));
#50131=CARTESIAN_POINT('Ctrl Pts',(-0.0358658119065493,0.00352927449325723,
-0.00312806260436819));
#50132=CARTESIAN_POINT('Ctrl Pts',(-0.0358773984533578,0.00352672229526407,
-0.00312407426270795));
#50133=CARTESIAN_POINT('Ctrl Pts',(-0.0358892505658731,0.00352411502968923,
-0.0031199950177777));
#50134=CARTESIAN_POINT('Ctrl Pts',(-0.0360340353943418,0.00349226480058136,
-0.00307016316065143));
#50135=CARTESIAN_POINT('Ctrl Pts',(-0.0362183141856735,0.00345212494100749,
-0.00300676298061814));
#50136=CARTESIAN_POINT('Ctrl Pts',(-0.0364391610694963,0.00340557668880201,
-0.0029308697522048));
#50137=CARTESIAN_POINT('',(-0.0364455123647,0.00340591076454288,0.00292997690155914));
#50138=CARTESIAN_POINT('Ctrl Pts',(-0.0364391610694963,0.00340557668880199,
-0.00293086975220478));
#50139=CARTESIAN_POINT('Ctrl Pts',(-0.0366322171547545,0.00336488594745255,
-0.00286452673010944));
#50140=CARTESIAN_POINT('Ctrl Pts',(-0.0368202498946822,0.00332281518765035,
-0.00279459104114316));
#50141=CARTESIAN_POINT('Ctrl Pts',(-0.0369926649570915,0.00328301199041162,
-0.00272634783401865));
#50142=CARTESIAN_POINT('Ctrl Pts',(-0.0371650800195008,0.00324320879317288,
-0.00265810462689414));
#50143=CARTESIAN_POINT('Ctrl Pts',(-0.0373212896723696,0.00320527811107744,
-0.00259151629192671));
#50144=CARTESIAN_POINT('Ctrl Pts',(-0.0374934455541359,0.00316088800823521,
-0.00250972996224946));
#50145=CARTESIAN_POINT('Ctrl Pts',(-0.0376508819930815,0.0031202932888204,
-0.00243493641835938));
#50146=CARTESIAN_POINT('Ctrl Pts',(-0.0378208106088136,0.00307439159668025,
-0.00234670930103131));
#50147=CARTESIAN_POINT('Ctrl Pts',(-0.0379716858037714,0.00303194552412074,
-0.0022594496374276));
#50148=CARTESIAN_POINT('Ctrl Pts',(-0.037985791806296,0.00302797704933699,
-0.00225129133787787));
#50149=CARTESIAN_POINT('Ctrl Pts',(-0.0379997479104133,0.00302403681227977,
-0.00224314220566623));
#50150=CARTESIAN_POINT('Ctrl Pts',(-0.0380135368744372,0.00302013075314561,
-0.0022350151484838));
#50151=CARTESIAN_POINT('Ctrl Pts',(-0.0381748100482325,0.00297444620769995,
-0.00213996259028189));
#50152=CARTESIAN_POINT('Ctrl Pts',(-0.038312309636301,0.00293311953030676,
-0.00204871414221153));
#50153=CARTESIAN_POINT('Ctrl Pts',(-0.0384600371843599,0.00288577414216096,
-0.00193316908477411));
#50154=CARTESIAN_POINT('Ctrl Pts',(-0.0386051400137966,0.00283926995339588,
-0.00181967695022035));
#50155=CARTESIAN_POINT('Ctrl Pts',(-0.0387586492955602,0.00278795635858161,
-0.00168181136542702));
#50156=CARTESIAN_POINT('Ctrl Pts',(-0.0388855191400815,0.00274380193022642,
-0.00154395937952611));
#50157=CARTESIAN_POINT('Ctrl Pts',(-0.0388878140480774,0.00274300323490941,
-0.00154146581909104));
#50158=CARTESIAN_POINT('Ctrl Pts',(-0.0388901012423995,0.00274220668911971,
-0.0015389723937722));
#50159=CARTESIAN_POINT('Ctrl Pts',(-0.0388923806047438,0.00274141234102353,
-0.00153647927517296));
#50160=CARTESIAN_POINT('Ctrl Pts',(-0.0390206703983249,0.00269670389282599,
-0.00139615859676874));
#50161=CARTESIAN_POINT('Ctrl Pts',(-0.0391239336719105,0.00265838818924466,
-0.00125737015421032));
#50162=CARTESIAN_POINT('Ctrl Pts',(-0.0392167430625687,0.00262253089827314,
-0.00109809991377156));
#50163=CARTESIAN_POINT('Ctrl Pts',(-0.0392749718618309,0.00260003396145177,
-0.000998173443042866));
#50164=CARTESIAN_POINT('Ctrl Pts',(-0.039328684790478,0.00257880129105425,
-0.000889923640323347));
#50165=CARTESIAN_POINT('Ctrl Pts',(-0.0393735992297108,0.00256086087193436,
-0.000777199960031099));
#50166=CARTESIAN_POINT('Ctrl Pts',(-0.0394002727639511,0.00255020651685718,
-0.00071025625557167));
#50167=CARTESIAN_POINT('Ctrl Pts',(-0.0394238946703283,0.00254070596688381,
-0.000641752316417933));
#50168=CARTESIAN_POINT('Ctrl Pts',(-0.0394439206157009,0.00253260235611844,
-0.000572334592845821));
#50169=CARTESIAN_POINT('Ctrl Pts',(-0.0394976674058036,0.00251085341699091,
-0.000386027292550317));
#50170=CARTESIAN_POINT('Ctrl Pts',(-0.0395245481484425,0.00249939378462001,
-0.000193588585587571));
#50171=CARTESIAN_POINT('Ctrl Pts',(-0.0395245044804478,0.00249944756631425,
-5.83969798006665E-7));
#50172=CARTESIAN_POINT('Ctrl Pts',(-0.0395244608124532,0.00249950134800849,
0.000192420645991558));
#50173=CARTESIAN_POINT('Ctrl Pts',(-0.0394974499353326,0.00251105592430073,
0.000385956457755352));
#50174=CARTESIAN_POINT('Ctrl Pts',(-0.0394437750762487,0.00253280713317883,
0.000572917666467489));
#50175=CARTESIAN_POINT('Ctrl Pts',(-0.0394235786421328,0.00254099153951996,
0.000643266239307942));
#50176=CARTESIAN_POINT('Ctrl Pts',(-0.039399665844055,0.0025505954007062,
0.00071267267253678));
#50177=CARTESIAN_POINT('Ctrl Pts',(-0.0393726489689033,0.00256137149458157,
0.000780388259510024));
#50178=CARTESIAN_POINT('Ctrl Pts',(-0.0393278647053818,0.00257923438305918,
0.000892636351656218));
#50179=CARTESIAN_POINT('Ctrl Pts',(-0.0392744071551819,0.0026003385220159,
0.00100020014102538));
#50180=CARTESIAN_POINT('Ctrl Pts',(-0.0392166403478267,0.00262273376753246,
0.00109956726159259));
#50181=CARTESIAN_POINT('Ctrl Pts',(-0.0391240247230632,0.00265863932905144,
0.00125887930208133));
#50182=CARTESIAN_POINT('Ctrl Pts',(-0.0390206909807072,0.00269703396732437,
0.00139746286942015));
#50183=CARTESIAN_POINT('Ctrl Pts',(-0.0388923702372792,0.00274183860381698,
0.00153769715301582));
#50184=CARTESIAN_POINT('Ctrl Pts',(-0.0388899378618459,0.00274268789516454,
0.00154035535477821));
#50185=CARTESIAN_POINT('Ctrl Pts',(-0.0388874965753729,0.0027435396942637,
0.00154301394633622));
#50186=CARTESIAN_POINT('Ctrl Pts',(-0.0388850465184323,0.00274439394252674,
0.00154567272298213));
#50187=CARTESIAN_POINT('Ctrl Pts',(-0.0387582430383768,0.00278860583441763,
0.00168327855809584));
#50188=CARTESIAN_POINT('Ctrl Pts',(-0.0386049180378238,0.00283996495012589,
0.00182099137683305));
#50189=CARTESIAN_POINT('Ctrl Pts',(-0.0384601201429457,0.00288638007257898,
0.00193416251744746));
#50190=CARTESIAN_POINT('Ctrl Pts',(-0.0383125245087059,0.00293369201342276,
0.00204952031522948));
#50191=CARTESIAN_POINT('Ctrl Pts',(-0.038175769856324,0.00297489082212998,
0.00214047070895444));
#50192=CARTESIAN_POINT('Ctrl Pts',(-0.0380152841178011,0.00302046341891065,
0.00223527013525858));
#50193=CARTESIAN_POINT('Ctrl Pts',(-0.0380013638600284,0.00302441630781155,
0.00224349287494253));
#50194=CARTESIAN_POINT('Ctrl Pts',(-0.0379872712832568,0.00302840453802309,
0.00225173873899062));
#50195=CARTESIAN_POINT('Ctrl Pts',(-0.037973024859638,0.00303242184803372,
0.00225999405200227));
#50196=CARTESIAN_POINT('Ctrl Pts',(-0.0378230252000953,0.0030747198415511,
0.00234691370105252));
#50197=CARTESIAN_POINT('Ctrl Pts',(-0.0376540512084115,0.00312046819384517,
0.00243479635430532));
#50198=CARTESIAN_POINT('Ctrl Pts',(-0.0374974436182988,0.00316102158131972,
0.00250941439811513));
#50199=CARTESIAN_POINT('Ctrl Pts',(-0.0373259620072885,0.00320542658245059,
0.00259111939308842));
#50200=CARTESIAN_POINT('Ctrl Pts',(-0.0371698572482878,0.00324337705647934,
0.00265761331386267));
#50201=CARTESIAN_POINT('Ctrl Pts',(-0.0369977736313312,0.00328321943549953,
0.00272576538045062));
#50202=CARTESIAN_POINT('Ctrl Pts',(-0.0368256900143745,0.00332306181451972,
0.00279391744703857));
#50203=CARTESIAN_POINT('Ctrl Pts',(-0.0366381245804503,0.00336517498387712,
0.00286373576666462));
#50204=CARTESIAN_POINT('Ctrl Pts',(-0.0364455123647003,0.00340591076454282,
0.00292997690155905));
#50205=CARTESIAN_POINT('',(-0.0328029016201836,0.0042087665877202,0.00416971706663987));
#50206=CARTESIAN_POINT('Ctrl Pts',(-0.0364455123647,0.00340591076454287,
0.00292997690155913));
#50207=CARTESIAN_POINT('Ctrl Pts',(-0.0362270644193021,0.00345211057323863,
0.00300510318396827));
#50208=CARTESIAN_POINT('Ctrl Pts',(-0.0360444782753564,0.00349201166437273,
0.00306795737029401));
#50209=CARTESIAN_POINT('Ctrl Pts',(-0.035900556669434,0.00352377780582171,
0.00311751449050552));
#50210=CARTESIAN_POINT('Ctrl Pts',(-0.0358866082105257,0.00352685648685669,
0.00312231742089569));
#50211=CARTESIAN_POINT('Ctrl Pts',(-0.0358730242130647,0.00352985940275686,
0.00312699546607101));
#50212=CARTESIAN_POINT('Ctrl Pts',(-0.035859807632643,0.00353278531481164,
0.00313154782206464));
#50213=CARTESIAN_POINT('Ctrl Pts',(-0.0357850143374938,0.0035493431986902,
0.0031573098342184));
#50214=CARTESIAN_POINT('Ctrl Pts',(-0.0357219488060029,0.00356341802743243,
0.00317903667032381));
#50215=CARTESIAN_POINT('Ctrl Pts',(-0.0356653693009525,0.00357608634117101,
0.00319852211497317));
#50216=CARTESIAN_POINT('Ctrl Pts',(-0.0356370795484272,0.0035824204980403,
0.00320826483729785));
#50217=CARTESIAN_POINT('Ctrl Pts',(-0.0356104112237838,0.0035884052174244,
0.00321744556903178));
#50218=CARTESIAN_POINT('Ctrl Pts',(-0.0355924301039697,0.00359244353562749,
0.00322363379433966));
#50219=CARTESIAN_POINT('Ctrl Pts',(-0.0355744489841556,0.00359648185383058,
0.00322982201964753));
#50220=CARTESIAN_POINT('Ctrl Pts',(-0.0355651552515481,0.00359856917227115,
0.00323302126335804));
#50221=CARTESIAN_POINT('Ctrl Pts',(-0.035535592160163,0.0036052117695187,
0.0032431750763029));
#50222=CARTESIAN_POINT('Ctrl Pts',(-0.0355060290687778,0.00361185436676625,
0.00325332888924775));
#50223=CARTESIAN_POINT('Ctrl Pts',(-0.0354562026487998,0.00362306570783562,
0.00327043166439547));
#50224=CARTESIAN_POINT('Ctrl Pts',(-0.0354122937915675,0.00363296676100046,
0.00328548603247098));
#50225=CARTESIAN_POINT('Ctrl Pts',(-0.0353831565381878,0.00363953695009156,
0.00329547588337435));
#50226=CARTESIAN_POINT('Ctrl Pts',(-0.0353566195302761,0.00364552894526491,
0.00330456953780217));
#50227=CARTESIAN_POINT('Ctrl Pts',(-0.0353307849961087,0.00365136731128944,
0.00331341831473545));
#50228=CARTESIAN_POINT('Ctrl Pts',(-0.0353176877594042,0.0036543271657732,
0.00331790434592494));
#50229=CARTESIAN_POINT('Ctrl Pts',(-0.0353047699888091,0.00365724785862674,
0.00332232776947711));
#50230=CARTESIAN_POINT('Ctrl Pts',(-0.035291777825036,0.0036601865624281,
0.00332677547357952));
#50231=CARTESIAN_POINT('Ctrl Pts',(-0.0352145389456363,0.0036776572618796,
0.00335321723391829));
#50232=CARTESIAN_POINT('Ctrl Pts',(-0.0351347725914307,0.00369574357075716,
0.00338047939885123));
#50233=CARTESIAN_POINT('Ctrl Pts',(-0.0350590289584748,0.00371293866348363,
0.00340633288155524));
#50234=CARTESIAN_POINT('Ctrl Pts',(-0.0349417405437824,0.00373956512814698,
0.00344636679440428));
#50235=CARTESIAN_POINT('Ctrl Pts',(-0.034833966823461,0.00376406627577167,
0.00348306531417552));
#50236=CARTESIAN_POINT('Ctrl Pts',(-0.0347236872682142,0.00378908587494196,
0.00352051902312663));
#50237=CARTESIAN_POINT('Ctrl Pts',(-0.0346915320539729,0.003796381067326,
0.00353143974213713));
#50238=CARTESIAN_POINT('Ctrl Pts',(-0.0346591514393833,0.00380372333820802,
0.00354242837528044));
#50239=CARTESIAN_POINT('Ctrl Pts',(-0.0346262097476452,0.00381118597583179,
0.00355359860795237));
#50240=CARTESIAN_POINT('Ctrl Pts',(-0.0344802911966427,0.00384424248298917,
0.00360307828188067));
#50241=CARTESIAN_POINT('Ctrl Pts',(-0.03432383153918,0.00387953556415316,
0.00365594651514581));
#50242=CARTESIAN_POINT('Ctrl Pts',(-0.0341701782162089,0.00391389558342509,
0.00370777216502179));
#50243=CARTESIAN_POINT('Ctrl Pts',(-0.0341342598584151,0.00392192766136619,
0.00371988704935457));
#50244=CARTESIAN_POINT('Ctrl Pts',(-0.0340984902611279,0.00392991018127384,
0.00373194625001173));
#50245=CARTESIAN_POINT('Ctrl Pts',(-0.034062832762441,0.00393785044789938,
0.00374396324604674));
#50246=CARTESIAN_POINT('Ctrl Pts',(-0.0339459528541134,0.00396387744557068,
0.00378335314849828));
#50247=CARTESIAN_POINT('Ctrl Pts',(-0.0338302896252035,0.00398944666719792,
0.00382228737361244));
#50248=CARTESIAN_POINT('Ctrl Pts',(-0.0337142953371807,0.00401485474041696,
0.00386135192035288));
#50249=CARTESIAN_POINT('Ctrl Pts',(-0.0335847662876927,0.00404322754764296,
0.00390497470294179));
#50250=CARTESIAN_POINT('Ctrl Pts',(-0.0334549040645208,0.00407138715560721,
0.00394874177972471));
#50251=CARTESIAN_POINT('Ctrl Pts',(-0.0333248665632899,0.0040992144746389,
0.00399266634821324));
#50252=CARTESIAN_POINT('Ctrl Pts',(-0.0331886125518466,0.00412837209309429,
0.00403869075348735));
#50253=CARTESIAN_POINT('Ctrl Pts',(-0.0330521528209864,0.00415716609479881,
0.00408489535755997));
#50254=CARTESIAN_POINT('Ctrl Pts',(-0.0329158597169497,0.00418544311210461,
0.00413124843967162));
#50255=CARTESIAN_POINT('Ctrl Pts',(-0.0328781890819101,0.00419325871808455,
0.00414406016665905));
#50256=CARTESIAN_POINT('Ctrl Pts',(-0.0328405345546385,0.00420103452583491,
0.00415688169838706));
#50257=CARTESIAN_POINT('Ctrl Pts',(-0.0328029014491621,0.00420876770681893,
0.00416971455610656));
#50258=CARTESIAN_POINT('Ctrl Pts',(-0.0399999989166323,0.00503323066735753,
0.00434914348573771));
#50259=CARTESIAN_POINT('Ctrl Pts',(-0.039711581140538,0.00502913112529287,
0.00434681829103734));
#50260=CARTESIAN_POINT('Ctrl Pts',(-0.0394894177154315,0.00502523749458704,
0.00434631164359477));
#50261=CARTESIAN_POINT('Ctrl Pts',(-0.0393406143928409,0.00502250803880602,
0.00434618840248981));
#50262=CARTESIAN_POINT('Ctrl Pts',(-0.0392662127315455,0.00502114331091552,
0.00434612678193733));
#50263=CARTESIAN_POINT('Ctrl Pts',(-0.0392101513869168,0.00502006695100079,
0.00434616560492587));
#50264=CARTESIAN_POINT('Ctrl Pts',(-0.0391653212214987,0.00501908324652545,
0.00434615465470367));
#50265=CARTESIAN_POINT('Ctrl Pts',(-0.0391429061387897,0.00501859139428778,
0.00434614917959258));
#50266=CARTESIAN_POINT('Ctrl Pts',(-0.0391232988904322,0.00501812092527449,
0.00434613436931875));
#50267=CARTESIAN_POINT('Ctrl Pts',(-0.0391162722622056,0.00501801715431804,
0.00434616679069379));
#50268=CARTESIAN_POINT('Ctrl Pts',(-0.0391127589480922,0.00501796526883981,
0.00434618300138131));
#50269=CARTESIAN_POINT('Ctrl Pts',(-0.0391123907856138,0.00501800519558459,
0.00434621078025896));
#50270=CARTESIAN_POINT('Ctrl Pts',(-0.0391101702857959,0.00501796303220673,
0.00434621586351736));
#50271=CARTESIAN_POINT('Ctrl Pts',(-0.0391079497859779,0.00501792086882887,
0.00434622094677576));
#50272=CARTESIAN_POINT('Ctrl Pts',(-0.0391038769436897,0.00501779685223246,
0.00434620292056547));
#50273=CARTESIAN_POINT('Ctrl Pts',(-0.039092954313039,0.00501741517263418,
0.0043461308499061));
#50274=CARTESIAN_POINT('Ctrl Pts',(-0.0390711090517377,0.00501665181343761,
0.00434598670858736));
#50275=CARTESIAN_POINT('Ctrl Pts',(-0.0390218648173137,0.00501485005279275,
0.0043456399058556));
#50276=CARTESIAN_POINT('Ctrl Pts',(-0.0389797747097396,0.00501320906924717,
0.00434533586273387));
#50277=CARTESIAN_POINT('Ctrl Pts',(-0.0389376846021655,0.0050115680857016,
0.00434503181961215));
#50278=CARTESIAN_POINT('Ctrl Pts',(-0.0389027483307743,0.00501009839743316,
0.00434475226826703));
#50279=CARTESIAN_POINT('Ctrl Pts',(-0.038866578037483,0.00500850610247983,
0.00434444753378693));
#50280=CARTESIAN_POINT('Ctrl Pts',(-0.0387942374509004,0.00500532151257317,
0.00434383806482675));
#50281=CARTESIAN_POINT('Ctrl Pts',(-0.0387169611433133,0.00500163550461192,
0.00434314683154966));
#50282=CARTESIAN_POINT('Ctrl Pts',(-0.0386401339110594,0.00499761879150246,
0.00434239304998539));
#50283=CARTESIAN_POINT('Ctrl Pts',(-0.0384864794465515,0.00498958536528355,
0.00434088548685686));
#50284=CARTESIAN_POINT('Ctrl Pts',(-0.0383346207956242,0.00498023760043779,
0.00433911356543341));
#50285=CARTESIAN_POINT('Ctrl Pts',(-0.0381870450731536,0.00496998227270427,
0.00433717084775423));
#50286=CARTESIAN_POINT('Ctrl Pts',(-0.0380394693506831,0.00495972694497075,
0.00433522813007506));
#50287=CARTESIAN_POINT('Ctrl Pts',(-0.0378961762638081,0.00494857311330899,
0.00433309893900448));
#50288=CARTESIAN_POINT('Ctrl Pts',(-0.0377495136538368,0.00493598755792319,
0.00433066417381591));
#50289=CARTESIAN_POINT('Ctrl Pts',(-0.0376028510438655,0.00492340200253738,
0.00432822940862735));
#50290=CARTESIAN_POINT('Ctrl Pts',(-0.0374528194588452,0.00490937444928368,
0.00432550627190693));
#50291=CARTESIAN_POINT('Ctrl Pts',(-0.0373028914612309,0.00489425572424894,
0.0043225615854874));
#50292=CARTESIAN_POINT('Ctrl Pts',(-0.0371529634636166,0.0048791369992142,
0.00431961689906786));
#50293=CARTESIAN_POINT('Ctrl Pts',(-0.0370031385604832,0.00486293516907937,
0.00431643738830799));
#50294=CARTESIAN_POINT('Ctrl Pts',(-0.0368471831474604,0.00484485748918042,
0.00431280949290434));
#50295=CARTESIAN_POINT('Ctrl Pts',(-0.0366912277344377,0.00482677980928146,
0.0043091815975007));
#50296=CARTESIAN_POINT('Ctrl Pts',(-0.0365291435108589,0.0048068043540339,
0.00430513969283296));
#50297=CARTESIAN_POINT('Ctrl Pts',(-0.0363823923887819,0.00478786232742212,
0.0043012714753759));
#50298=CARTESIAN_POINT('Ctrl Pts',(-0.0362356412667049,0.00476892030081034,
0.00429740325791884));
#50299=CARTESIAN_POINT('Ctrl Pts',(-0.0361042200002657,0.00475104735615687,
0.00429365574570242));
#50300=CARTESIAN_POINT('Ctrl Pts',(-0.0359631726729839,0.0047311683590897,
0.00428942794780173));
#50301=CARTESIAN_POINT('Ctrl Pts',(-0.0358221253457021,0.00471128936202254,
0.00428520014990104));
#50302=CARTESIAN_POINT('Ctrl Pts',(-0.0356714544382095,0.00468938023788155,
0.00428052580056473));
#50303=CARTESIAN_POINT('Ctrl Pts',(-0.0355174660492713,0.00466619058057617,
0.00427549612867958));
#50304=CARTESIAN_POINT('Ctrl Pts',(-0.0354404718548022,0.00465459575192348,
0.004272981292737));
#50305=CARTESIAN_POINT('Ctrl Pts',(-0.035362648125467,0.00464268212391236,
0.00427037596598903));
#50306=CARTESIAN_POINT('Ctrl Pts',(-0.0352846830820956,0.0046305817879156,
0.00426771571664521));
#50307=CARTESIAN_POINT('Ctrl Pts',(-0.0352067180387242,0.00461848145191885,
0.00426505546730138));
#50308=CARTESIAN_POINT('Ctrl Pts',(-0.0351286115346058,0.00460619582423831,
0.00426233832436842));
#50309=CARTESIAN_POINT('Ctrl Pts',(-0.0350452817127376,0.00459288652142108,
0.00425936094303203));
#50310=CARTESIAN_POINT('Ctrl Pts',(-0.0350036168018035,0.00458623187001247,
0.00425787225236383));
#50311=CARTESIAN_POINT('Ctrl Pts',(-0.0349606463711649,0.00457931863118851,
0.00425632189955588));
#50312=CARTESIAN_POINT('Ctrl Pts',(-0.0349380016209598,0.00457566243006404,
0.00425549928983568));
#50313=CARTESIAN_POINT('Ctrl Pts',(-0.0349153568707547,0.00457200622893958,
0.00425467668011547));
#50314=CARTESIAN_POINT('Ctrl Pts',(-0.0349130374120522,0.00457161034223773,
0.00425457772917389));
#50315=CARTESIAN_POINT('Ctrl Pts',(-0.0349053710842191,0.00457033836329817,
0.00425427430389109));
#50316=CARTESIAN_POINT('Ctrl Pts',(-0.0348900384285529,0.00456779440541904,
0.00425366745332548));
#50317=CARTESIAN_POINT('Ctrl Pts',(-0.0348533188437881,0.0045617414677081,
0.00425224845367909));
#50318=CARTESIAN_POINT('Ctrl Pts',(-0.034813518170537,0.00455512497361659,
0.00425068480677904));
#50319=CARTESIAN_POINT('Ctrl Pts',(-0.0347339168240347,0.00454189198543359,
0.00424755751297895));
#50320=CARTESIAN_POINT('Ctrl Pts',(-0.0346419899576794,0.00452641460551389,
0.00424383939069223));
#50321=CARTESIAN_POINT('Ctrl Pts',(-0.0345234582519701,0.00450632423353793,
0.00423905828357747));
#50322=CARTESIAN_POINT('Ctrl Pts',(-0.0344049265462607,0.00448623386156196,
0.0042342771764627));
#50323=CARTESIAN_POINT('Ctrl Pts',(-0.0342597908811681,0.00446152376856126,
0.00422844041257158));
#50324=CARTESIAN_POINT('Ctrl Pts',(-0.0340916301155351,0.00443270371878135,
0.00422171509726581));
#50325=CARTESIAN_POINT('Ctrl Pts',(-0.033755308584269,0.00437506361922152,
0.00420826446665425));
#50326=CARTESIAN_POINT('Ctrl Pts',(-0.0333269077952901,0.00430084306725824,
0.00419133495359302));
#50327=CARTESIAN_POINT('Ctrl Pts',(-0.0328029052223737,0.0042087689636135,
0.00416971896312806));
#50328=CARTESIAN_POINT('Ctrl Pts',(-0.04,0.00997687591821936,-0.00434339564002003));
#50329=CARTESIAN_POINT('Ctrl Pts',(-0.0366885717327396,0.00997687591821936,
-0.00434339564002003));
#50330=CARTESIAN_POINT('Ctrl Pts',(-0.0338250628738108,0.0101232964422964,
-0.00449314468513572));
#50331=CARTESIAN_POINT('Ctrl Pts',(-0.0311299933513177,0.0103662543728445,
-0.00486696278424518));
#50332=CARTESIAN_POINT('Ctrl Pts',(-0.04,0.0107388615197248,-0.00390886377996825));
#50333=CARTESIAN_POINT('Ctrl Pts',(-0.0367159969968672,0.0107388615197248,
-0.00390886377996825));
#50334=CARTESIAN_POINT('Ctrl Pts',(-0.0338649863625956,0.0108410632031505,
-0.00400561616999478));
#50335=CARTESIAN_POINT('Ctrl Pts',(-0.0311724810188551,0.011010647908647,
-0.00427784708467796));
#50336=CARTESIAN_POINT('Ctrl Pts',(-0.04,0.0120285654953516,-0.00263057838182841));
#50337=CARTESIAN_POINT('Ctrl Pts',(-0.0367708476877013,0.0120285654953516,
-0.00263057838182841));
#50338=CARTESIAN_POINT('Ctrl Pts',(-0.0339449440082147,0.0120559242133456,
-0.00266140852833637));
#50339=CARTESIAN_POINT('Ctrl Pts',(-0.0312576750393058,0.0121013205007559,
-0.00278583369248179));
#50340=CARTESIAN_POINT('Ctrl Pts',(-0.04,0.0127366477880115,4.35202123928724E-7));
#50341=CARTESIAN_POINT('Ctrl Pts',(-0.0367665215704158,0.0127366477880115,
4.35202123928724E-7));
#50342=CARTESIAN_POINT('Ctrl Pts',(-0.033936097062896,0.0127229154815913,
2.59498982767992E-6));
#50343=CARTESIAN_POINT('Ctrl Pts',(-0.0312436761854233,0.0127001287639775,
7.2219948256526E-6));
#50344=CARTESIAN_POINT('Ctrl Pts',(-0.04,0.0120281281938075,0.00263133105653345));
#50345=CARTESIAN_POINT('Ctrl Pts',(-0.0367570493854284,0.0120281281938075,
0.00263133105653345));
#50346=CARTESIAN_POINT('Ctrl Pts',(-0.0339195876897249,0.0120555116847181,
0.00266649147709405));
#50347=CARTESIAN_POINT('Ctrl Pts',(-0.0312212323834849,0.0121009494899832,
0.00280018576913209));
#50348=CARTESIAN_POINT('Ctrl Pts',(-0.04,0.0107382117670507,0.00390940207014268));
#50349=CARTESIAN_POINT('Ctrl Pts',(-0.0366933059897235,0.0107382117670507,
0.00390940207014268));
#50350=CARTESIAN_POINT('Ctrl Pts',(-0.0338229608340258,0.0108404502398202,
0.00401050490853467));
#50351=CARTESIAN_POINT('Ctrl Pts',(-0.0311118088133509,0.0110100966150892,
0.00429203315759127));
#50352=CARTESIAN_POINT('Ctrl Pts',(-0.04,0.00997615395078692,0.0043438072715076));
#50353=CARTESIAN_POINT('Ctrl Pts',(-0.036661434210569,0.00997615395078692,
0.0043438072715076));
#50354=CARTESIAN_POINT('Ctrl Pts',(-0.0337745920634133,0.0101226153439546,
0.00449791927069512));
#50355=CARTESIAN_POINT('Ctrl Pts',(-0.0310569876683288,0.010365641789481,
0.00488105194237219));
#50356=CARTESIAN_POINT('',(-0.0347727610542622,0.012000956525018,-0.00227981334747213));
#50357=CARTESIAN_POINT('',(-0.0312271855506422,0.0110770582020895,-0.00409339326150648));
#50358=CARTESIAN_POINT('Ctrl Pts',(-0.0347727610542622,0.012000956525018,
-0.00227981334747212));
#50359=CARTESIAN_POINT('Ctrl Pts',(-0.0347662162249802,0.0119994708798832,
-0.00228333575096989));
#50360=CARTESIAN_POINT('Ctrl Pts',(-0.0346907936442485,0.0119827318232676,
-0.00232385956332954));
#50361=CARTESIAN_POINT('Ctrl Pts',(-0.0345418896085024,0.0119471677082457,
-0.00240444031058215));
#50362=CARTESIAN_POINT('Ctrl Pts',(-0.0344738490314361,0.0119309169538802,
-0.00244126107582215));
#50363=CARTESIAN_POINT('Ctrl Pts',(-0.0343905139349971,0.0119106560343659,
-0.0024864354481445));
#50364=CARTESIAN_POINT('Ctrl Pts',(-0.0342965588584313,0.011887132404934,
-0.00253740875700026));
#50365=CARTESIAN_POINT('Ctrl Pts',(-0.034236301287015,0.0118720456546244,
-0.00257010020818064));
#50366=CARTESIAN_POINT('Ctrl Pts',(-0.0341731823267349,0.0118560350353544,
-0.00260435876863534));
#50367=CARTESIAN_POINT('Ctrl Pts',(-0.0340949388892498,0.0118357864876751,
-0.00264679134155758));
#50368=CARTESIAN_POINT('Ctrl Pts',(-0.0340646226447708,0.0118279409744727,
-0.00266323228914288));
#50369=CARTESIAN_POINT('Ctrl Pts',(-0.0340320390897621,0.0118194510631183,
-0.00268089710286973));
#50370=CARTESIAN_POINT('Ctrl Pts',(-0.0340002251881336,0.0118111051586246,
-0.00269813252557422));
#50371=CARTESIAN_POINT('Ctrl Pts',(-0.033961994181482,0.0118010758219548,
-0.00271884446363681));
#50372=CARTESIAN_POINT('Ctrl Pts',(-0.0339248656177919,0.0117912519918997,
-0.00273893933469951));
#50373=CARTESIAN_POINT('Ctrl Pts',(-0.0338943260618987,0.0117831360576042,
-0.00275544446672193));
#50374=CARTESIAN_POINT('Ctrl Pts',(-0.0338383730389783,0.0117682664550715,
-0.00278568433116486));
#50375=CARTESIAN_POINT('Ctrl Pts',(-0.0338044172619026,0.0117591280377497,
-0.00280401656801114));
#50376=CARTESIAN_POINT('Ctrl Pts',(-0.0337658113104114,0.0117487234303718,
-0.00282481271370906));
#50377=CARTESIAN_POINT('Ctrl Pts',(-0.0337272053589202,0.0117383188229939,
-0.00284560885940698));
#50378=CARTESIAN_POINT('Ctrl Pts',(-0.0336839476070479,0.0117266082277593,
-0.002868845618102));
#50379=CARTESIAN_POINT('Ctrl Pts',(-0.0336427042610508,0.0117153823389272,
-0.00289094862413562));
#50380=CARTESIAN_POINT('Ctrl Pts',(-0.0336265071504343,0.0117109737013934,
-0.00289962892940737));
#50381=CARTESIAN_POINT('Ctrl Pts',(-0.0336106180654591,0.0117066401691773,
-0.00290813652225827));
#50382=CARTESIAN_POINT('Ctrl Pts',(-0.0335949886689743,0.0117023701389523,
-0.00291649748682474));
#50383=CARTESIAN_POINT('Ctrl Pts',(-0.0335310225595433,0.0116848942741027,
-0.00295071623448586));
#50384=CARTESIAN_POINT('Ctrl Pts',(-0.0334714329877785,0.0116684952021746,
-0.00298246811210692));
#50385=CARTESIAN_POINT('Ctrl Pts',(-0.0334126721852774,0.0116522695073128,
-0.00301364109545719));
#50386=CARTESIAN_POINT('Ctrl Pts',(-0.0333395538442574,0.0116320792471445,
-0.00305243084525968));
#50387=CARTESIAN_POINT('Ctrl Pts',(-0.0332677431191887,0.0116121490182614,
-0.00309030074696719));
#50388=CARTESIAN_POINT('Ctrl Pts',(-0.0332040782600887,0.011594446505781,
-0.00312370844975335));
#50389=CARTESIAN_POINT('Ctrl Pts',(-0.0331902389087889,0.0115905983658092,
-0.00313097055543473));
#50390=CARTESIAN_POINT('Ctrl Pts',(-0.0331767719966812,0.0115868537675826,
-0.00313802634461842));
#50391=CARTESIAN_POINT('Ctrl Pts',(-0.0331634772545252,0.011583157686754,
-0.00314498140164933));
#50392=CARTESIAN_POINT('Ctrl Pts',(-0.0331156124908776,0.0115698507693872,
-0.00317002153834643));
#50393=CARTESIAN_POINT('Ctrl Pts',(-0.0330700704267301,0.0115571966523754,
-0.00319372493591726));
#50394=CARTESIAN_POINT('Ctrl Pts',(-0.0330167657676819,0.0115424264317148,
-0.00322127745264625));
#50395=CARTESIAN_POINT('Ctrl Pts',(-0.032948655400974,0.0115235536884403,
-0.00325648285591949));
#50396=CARTESIAN_POINT('Ctrl Pts',(-0.0328679304816266,0.0115012287484612,
-0.00329790419386068));
#50397=CARTESIAN_POINT('Ctrl Pts',(-0.0327909578303375,0.0114800362569381,
-0.00333705744501196));
#50398=CARTESIAN_POINT('Ctrl Pts',(-0.0327573110869359,0.0114707724689254,
-0.00335417234715916));
#50399=CARTESIAN_POINT('Ctrl Pts',(-0.0327243697723556,0.011461725602602,
-0.00337086051058516));
#50400=CARTESIAN_POINT('Ctrl Pts',(-0.0326918474558674,0.0114528169513001,
-0.00338727608029467));
#50401=CARTESIAN_POINT('Ctrl Pts',(-0.0326499694389777,0.0114413455467393,
-0.00340841391977791));
#50402=CARTESIAN_POINT('Ctrl Pts',(-0.0326087884759492,0.0114301038343232,
-0.00342909906358724));
#50403=CARTESIAN_POINT('Ctrl Pts',(-0.0325676120192666,0.0114189070941222,
-0.00344969210741507));
#50404=CARTESIAN_POINT('Ctrl Pts',(-0.0324324977420077,0.0113821666948313,
-0.00351726504733077));
#50405=CARTESIAN_POINT('Ctrl Pts',(-0.032297606118495,0.0113459495619924,
-0.00358378257787548));
#50406=CARTESIAN_POINT('Ctrl Pts',(-0.0321620057256791,0.0113102703660507,
-0.00364974238539242));
#50407=CARTESIAN_POINT('Ctrl Pts',(-0.0321507718423466,0.0113073145049629,
-0.0036552068591074));
#50408=CARTESIAN_POINT('Ctrl Pts',(-0.0321395333106712,0.0113043623100987,
-0.00366066739946016));
#50409=CARTESIAN_POINT('Ctrl Pts',(-0.0321282891655846,0.0113014137098195,
-0.00366612453785849));
#50410=CARTESIAN_POINT('Ctrl Pts',(-0.0320417758799519,0.0112787269607416,
-0.00370811216513983));
#50411=CARTESIAN_POINT('Ctrl Pts',(-0.0319549400458757,0.0112562481925477,
-0.00374990739672547));
#50412=CARTESIAN_POINT('Ctrl Pts',(-0.031867579817233,0.0112339722338532,
-0.00379165633688003));
#50413=CARTESIAN_POINT('Ctrl Pts',(-0.0317617277771904,0.0112069810536747,
-0.00384224240509021));
#50414=CARTESIAN_POINT('Ctrl Pts',(-0.031655096866317,0.011180287153048,
-0.003892766024649));
#50415=CARTESIAN_POINT('Ctrl Pts',(-0.031547327846147,0.0111538702353446,
-0.00394349975127678));
#50416=CARTESIAN_POINT('Ctrl Pts',(-0.0314418503941371,0.0111280150390655,
-0.0039931546911401));
#50417=CARTESIAN_POINT('Ctrl Pts',(-0.0313352791840738,0.0111024246360599,
-0.00404301369035159));
#50418=CARTESIAN_POINT('Ctrl Pts',(-0.0312271883190323,0.0110770591286335,
-0.0040933922183782));
#50419=CARTESIAN_POINT('Ctrl Pts',(-0.0399999969232478,0.00997687592866901,
-0.00434339563406105));
#50420=CARTESIAN_POINT('Ctrl Pts',(-0.0395738517935777,0.00998089464425918,
-0.00434110392960138));
#50421=CARTESIAN_POINT('Ctrl Pts',(-0.0391781870153202,0.00999130333547632,
-0.00433902484280308));
#50422=CARTESIAN_POINT('Ctrl Pts',(-0.0388078014104782,0.010007542172654,
-0.0043362037413784));
#50423=CARTESIAN_POINT('Ctrl Pts',(-0.0386226084475415,0.0100156615982803,
-0.00433479318944348));
#50424=CARTESIAN_POINT('Ctrl Pts',(-0.0384437358201049,0.0100252444432719,
-0.00433320817237369));
#50425=CARTESIAN_POINT('Ctrl Pts',(-0.0382763937035359,0.0100357889612725,
-0.00433138882420424));
#50426=CARTESIAN_POINT('Ctrl Pts',(-0.0381090515869669,0.0100463334792731,
-0.0043295694760348));
#50427=CARTESIAN_POINT('Ctrl Pts',(-0.037953239061578,0.0100578130509366,
-0.00432747007831575));
#50428=CARTESIAN_POINT('Ctrl Pts',(-0.037788101735501,0.010071778232986,
-0.0043247184724149));
#50429=CARTESIAN_POINT('Ctrl Pts',(-0.0374578270833469,0.0100997085970848,
-0.0043192152606132));
#50430=CARTESIAN_POINT('Ctrl Pts',(-0.0370902617756126,0.0101377503212127,
-0.0043113870511226));
#50431=CARTESIAN_POINT('Ctrl Pts',(-0.036719991551943,0.010182450920575,
-0.0043020261361203));
#50432=CARTESIAN_POINT('Ctrl Pts',(-0.0365348564401082,0.0102048012202561,
-0.00429734567861916));
#50433=CARTESIAN_POINT('Ctrl Pts',(-0.0363490431730722,0.0102287930336494,
-0.00429224677147734));
#50434=CARTESIAN_POINT('Ctrl Pts',(-0.0361629038294802,0.0102541382250016,
-0.00428678656364088));
#50435=CARTESIAN_POINT('Ctrl Pts',(-0.0360698341576842,0.0102668108206777,
-0.00428405645972265));
#50436=CARTESIAN_POINT('Ctrl Pts',(-0.0359766828489092,0.0102798199653733,
-0.00428123305530202));
#50437=CARTESIAN_POINT('Ctrl Pts',(-0.0358785913924785,0.0102939117478491,
-0.0042781242773886));
#50438=CARTESIAN_POINT('Ctrl Pts',(-0.0357804999360477,0.010308003530325,
-0.00427501549947518));
#50439=CARTESIAN_POINT('Ctrl Pts',(-0.0356774693366876,0.0103231880445341,
-0.00427163559790304));
#50440=CARTESIAN_POINT('Ctrl Pts',(-0.0355904281524484,0.0103362437577912,
-0.00426871175137701));
#50441=CARTESIAN_POINT('Ctrl Pts',(-0.0355033869682092,0.0103492994710482,
-0.00426578790485099));
#50442=CARTESIAN_POINT('Ctrl Pts',(-0.0354323335052546,0.0103602105430234,
-0.00426329869026004));
#50443=CARTESIAN_POINT('Ctrl Pts',(-0.0353541216407747,0.0103723925303275,
-0.00426049197487973));
#50444=CARTESIAN_POINT('Ctrl Pts',(-0.0352759097762947,0.0103845745176317,
-0.00425768525949942));
#50445=CARTESIAN_POINT('Ctrl Pts',(-0.0351905405864586,0.0103980370683696,
-0.00425457369612543));
#50446=CARTESIAN_POINT('Ctrl Pts',(-0.0351042461552928,0.010411833918664,
-0.00425136745846616));
#50447=CARTESIAN_POINT('Ctrl Pts',(-0.0349316572929612,0.0104394276192529,
-0.00424495498314762));
#50448=CARTESIAN_POINT('Ctrl Pts',(-0.0347553659619536,0.0104683456523605,
-0.00423814780461085));
#50449=CARTESIAN_POINT('Ctrl Pts',(-0.0345637802517622,0.0105004831389811,
-0.0042304709836301));
#50450=CARTESIAN_POINT('Ctrl Pts',(-0.0343721945415708,0.0105326206256018,
-0.00422279416264936));
#50451=CARTESIAN_POINT('Ctrl Pts',(-0.0341653165318991,0.0105679934601369,
-0.00421426474276195));
#50452=CARTESIAN_POINT('Ctrl Pts',(-0.03396901109119,0.0106019602844291,
-0.00420601505060714));
#50453=CARTESIAN_POINT('Ctrl Pts',(-0.0337727056504808,0.0106359271087213,
-0.00419776535845234));
#50454=CARTESIAN_POINT('Ctrl Pts',(-0.0335869704556112,0.0106684707640346,
-0.00418977769754576));
#50455=CARTESIAN_POINT('Ctrl Pts',(-0.0334035706353302,0.0107005985088829,
-0.00418196081844651));
#50456=CARTESIAN_POINT('Ctrl Pts',(-0.0332201708150493,0.0107327262537313,
-0.00417414393934726));
#50457=CARTESIAN_POINT('Ctrl Pts',(-0.033039107416087,0.0107644457777805,
-0.0041665051414215));
#50458=CARTESIAN_POINT('Ctrl Pts',(-0.0328575587521421,0.0107963002655774,
-0.0041587950627355));
#50459=CARTESIAN_POINT('Ctrl Pts',(-0.0326760100881971,0.0108281547533742,
-0.0041510849840495));
#50460=CARTESIAN_POINT('Ctrl Pts',(-0.032493976134264,0.0108601443570704,
-0.00414330399826378));
#50461=CARTESIAN_POINT('Ctrl Pts',(-0.0323160004717604,0.0108915520131664,
-0.0041354509857575));
#50462=CARTESIAN_POINT('Ctrl Pts',(-0.0322270126405086,0.0109072558412144,
-0.00413152447950437));
#50463=CARTESIAN_POINT('Ctrl Pts',(-0.0321390390296874,0.0109228115832411,
-0.00412757802328178));
#50464=CARTESIAN_POINT('Ctrl Pts',(-0.032058751349319,0.0109368485082703,
-0.00412412547505019));
#50465=CARTESIAN_POINT('Ctrl Pts',(-0.0319784636689506,0.0109508854332996,
-0.00412067292681859));
#50466=CARTESIAN_POINT('Ctrl Pts',(-0.0319058625544242,0.0109634080368383,
-0.00411771731119518));
#50467=CARTESIAN_POINT('Ctrl Pts',(-0.0318233652299006,0.0109774606394118,
-0.00411453809373492));
#50468=CARTESIAN_POINT('Ctrl Pts',(-0.0316583705808533,0.0110055658445589,
-0.00410817965881439));
#50469=CARTESIAN_POINT('Ctrl Pts',(-0.0314537906056737,0.0110397887429251,
-0.00410092050257926));
#50470=CARTESIAN_POINT('Ctrl Pts',(-0.0312272002437396,0.0110770530880674,
-0.00409339712395557));
#50471=CARTESIAN_POINT('',(-0.0311805491196909,0.0110755203513828,0.00410667728630412));
#50472=CARTESIAN_POINT('Ctrl Pts',(-0.0311805648084427,0.0110755143676243,
0.00410668200447306));
#50473=CARTESIAN_POINT('Ctrl Pts',(-0.0313371568854333,0.0110497540541028,
0.00411147974496858));
#50474=CARTESIAN_POINT('Ctrl Pts',(-0.0315032409861522,0.0110220279747615,
0.00411696689026756));
#50475=CARTESIAN_POINT('Ctrl Pts',(-0.0316901958519466,0.010990269889629,
0.00412364605205666));
#50476=CARTESIAN_POINT('Ctrl Pts',(-0.031877150717741,0.0109585118044965,
0.00413032521384576));
#50477=CARTESIAN_POINT('Ctrl Pts',(-0.0320849742587853,0.0109227073742163,
0.0041381857078831));
#50478=CARTESIAN_POINT('Ctrl Pts',(-0.03227706278129,0.0108894139580456,
0.00414560009689503));
#50479=CARTESIAN_POINT('Ctrl Pts',(-0.0324691513037948,0.0108561205418749,
0.00415301448590696));
#50480=CARTESIAN_POINT('Ctrl Pts',(-0.0326455063356221,0.0108253481113506,
0.00415998828010131));
#50481=CARTESIAN_POINT('Ctrl Pts',(-0.0328258638881128,0.0107939394614203,
0.00416708628235608));
#50482=CARTESIAN_POINT('Ctrl Pts',(-0.0330062214406034,0.01076253081149,
0.00417418428461086));
#50483=CARTESIAN_POINT('Ctrl Pts',(-0.0331905823077373,0.0107304917967662,
0.00418141299511146));
#50484=CARTESIAN_POINT('Ctrl Pts',(-0.0333738417105198,0.0106983687695328,
0.00418895670506269));
#50485=CARTESIAN_POINT('Ctrl Pts',(-0.0337403605160849,0.0106341227150661,
0.00420404412496513));
#50486=CARTESIAN_POINT('Ctrl Pts',(-0.0341024613721,0.0105694464301792,
0.00422028417680778));
#50487=CARTESIAN_POINT('Ctrl Pts',(-0.0344647676792294,0.0105081464292615,
0.0042345923946209));
#50488=CARTESIAN_POINT('Ctrl Pts',(-0.0348270739863588,0.0104468464283438,
0.00424890061243402));
#50489=CARTESIAN_POINT('Ctrl Pts',(-0.0351895922052,0.0103889807025132,
0.00426136261367898));
#50490=CARTESIAN_POINT('Ctrl Pts',(-0.0355611770151797,0.0103340570263314,
0.00427288930827505));
#50491=CARTESIAN_POINT('Ctrl Pts',(-0.0359327618251594,0.0102791333501495,
0.00428441600287112));
#50492=CARTESIAN_POINT('Ctrl Pts',(-0.0363134177233673,0.0102271929237579,
0.00429506336753169));
#50493=CARTESIAN_POINT('Ctrl Pts',(-0.0366843211943214,0.0101825886185625,
0.00430403705182438));
#50494=CARTESIAN_POINT('Ctrl Pts',(-0.0370552246652755,0.0101379843133672,
0.00431301073611707));
#50495=CARTESIAN_POINT('Ctrl Pts',(-0.0374163694815425,0.0101006527765711,
0.00432021620435609));
#50496=CARTESIAN_POINT('Ctrl Pts',(-0.037785030861159,0.0100697780674643,
0.00432610688485246));
#50497=CARTESIAN_POINT('Ctrl Pts',(-0.0378771962060632,0.0100620593901876,
0.00432757955497655));
#50498=CARTESIAN_POINT('Ctrl Pts',(-0.0379698317952406,0.0100547517233659,
0.0043289821701388));
#50499=CARTESIAN_POINT('Ctrl Pts',(-0.0380529341974252,0.0100486088393398,
0.0043301407721085));
#50500=CARTESIAN_POINT('Ctrl Pts',(-0.0381360365996097,0.0100424659553138,
0.00433129937407819));
#50501=CARTESIAN_POINT('Ctrl Pts',(-0.0382096052190389,0.0100374751681415,
0.00433219261129474));
#50502=CARTESIAN_POINT('Ctrl Pts',(-0.0382877151654865,0.0100326093935622,
0.00433301336685188));
#50503=CARTESIAN_POINT('Ctrl Pts',(-0.0384439350583817,0.0100228778444037,
0.00433465487796617));
#50504=CARTESIAN_POINT('Ctrl Pts',(-0.0386183217531855,0.0100136844537418,
0.00433607137582392));
#50505=CARTESIAN_POINT('Ctrl Pts',(-0.0388006428457909,0.0100058927764429,
0.00433731100066326));
#50506=CARTESIAN_POINT('Ctrl Pts',(-0.0391652846248559,0.00999030943920216,
0.00433979024758051));
#50507=CARTESIAN_POINT('Ctrl Pts',(-0.0395616602579697,0.00998027460548254,
0.00434145834687895));
#50508=CARTESIAN_POINT('Ctrl Pts',(-0.0399999963064522,0.00997615396455589,
0.0043438072636588));
#50509=CARTESIAN_POINT('',(-0.034761114924408,0.0120023525649548,0.00228080342275957));
#50510=CARTESIAN_POINT('Ctrl Pts',(-0.0311805519738734,0.0110755212028574,
0.00410667612600569));
#50511=CARTESIAN_POINT('Ctrl Pts',(-0.0312918893531326,0.0111015040086574,
0.00405492486269926));
#50512=CARTESIAN_POINT('Ctrl Pts',(-0.0314017335980751,0.0111277460894534,
0.00400366400621591));
#50513=CARTESIAN_POINT('Ctrl Pts',(-0.0315104679833535,0.0111542739003986,
0.00395259289717512));
#50514=CARTESIAN_POINT('Ctrl Pts',(-0.0316184123909562,0.0111806089813405,
0.00390189283024682));
#50515=CARTESIAN_POINT('Ctrl Pts',(-0.0317252674010335,0.0112072263396688,
0.00385137641012631));
#50516=CARTESIAN_POINT('Ctrl Pts',(-0.0318313013275745,0.01123412287288,
0.0038008189377741));
#50517=CARTESIAN_POINT('Ctrl Pts',(-0.0319182047370657,0.0112561667650172,
0.00375938298547096));
#50518=CARTESIAN_POINT('Ctrl Pts',(-0.0320045596728881,0.0112783978373286,
0.00371791719079459));
#50519=CARTESIAN_POINT('Ctrl Pts',(-0.0320905660624497,0.0113008209554723,
0.00367628081283267));
#50520=CARTESIAN_POINT('Ctrl Pts',(-0.0321026129250342,0.0113039617479688,
0.00367044883073946));
#50521=CARTESIAN_POINT('Ctrl Pts',(-0.0321146523625482,0.0113071063118642,
0.00366461350737955));
#50522=CARTESIAN_POINT('Ctrl Pts',(-0.0321266856106329,0.0113102547460609,
0.00365877417887169));
#50523=CARTESIAN_POINT('Ctrl Pts',(-0.0322628118099773,0.0113458714289443,
0.00359271673611796));
#50524=CARTESIAN_POINT('Ctrl Pts',(-0.0323981143072709,0.0113819863572385,
0.00352616264000121));
#50525=CARTESIAN_POINT('Ctrl Pts',(-0.0325337400951053,0.0114186401173113,
0.0034585154464424));
#50526=CARTESIAN_POINT('Ctrl Pts',(-0.0325752451621761,0.0114298571343293,
0.0034378136215856));
#50527=CARTESIAN_POINT('Ctrl Pts',(-0.0326167633897675,0.0114411208131778,
0.00341701578897169));
#50528=CARTESIAN_POINT('Ctrl Pts',(-0.0326590147018697,0.0114526223625216,
0.00339574828950089));
#50529=CARTESIAN_POINT('Ctrl Pts',(-0.0326918978185774,0.0114615737245165,
0.00337919633803755));
#50530=CARTESIAN_POINT('Ctrl Pts',(-0.0327252236306174,0.0114706688758631,
0.00336236029861347));
#50531=CARTESIAN_POINT('Ctrl Pts',(-0.032759291126813,0.0114799895158526,
0.00334507974729073));
#50532=CARTESIAN_POINT('Ctrl Pts',(-0.0328371317369472,0.0115012861881837,
0.00330559552307026));
#50533=CARTESIAN_POINT('Ctrl Pts',(-0.0329189086742722,0.0115237573151514,
0.00326375361780902));
#50534=CARTESIAN_POINT('Ctrl Pts',(-0.0329874853269181,0.011542635819523,
0.00322841091201546));
#50535=CARTESIAN_POINT('Ctrl Pts',(-0.0330410365704526,0.0115573779707679,
0.00320081192938659));
#50536=CARTESIAN_POINT('Ctrl Pts',(-0.0330865025860455,0.0115699282316569,
0.0031772185812425));
#50537=CARTESIAN_POINT('Ctrl Pts',(-0.0331343405503289,0.0115831402852154,
0.00315226931100933));
#50538=CARTESIAN_POINT('Ctrl Pts',(-0.0331477629274199,0.0115868473234991,
0.00314526904420802));
#50539=CARTESIAN_POINT('Ctrl Pts',(-0.0331613648801142,0.0115906045911974,
0.00313816443928055));
#50540=CARTESIAN_POINT('Ctrl Pts',(-0.0331753611862401,0.0115944707197936,
0.00313084263796009));
#50541=CARTESIAN_POINT('Ctrl Pts',(-0.0332392409659126,0.0116121159070799,
0.00309742560271175));
#50542=CARTESIAN_POINT('Ctrl Pts',(-0.0333116000603191,0.0116320643618833,
0.00305938956895168));
#50543=CARTESIAN_POINT('Ctrl Pts',(-0.0333856189510863,0.011652363846843,
0.003020250876743));
#50544=CARTESIAN_POINT('Ctrl Pts',(-0.0334451841017341,0.0116686994318155,
0.00298875483467318));
#50545=CARTESIAN_POINT('Ctrl Pts',(-0.0335058104640706,0.0116852674860886,
0.00295655835990366));
#50546=CARTESIAN_POINT('Ctrl Pts',(-0.0335705269574241,0.0117028231560492,
0.00292205539953335));
#50547=CARTESIAN_POINT('Ctrl Pts',(-0.0335862306930179,0.011707083114909,
0.0029136831077298));
#50548=CARTESIAN_POINT('Ctrl Pts',(-0.0336021740916453,0.011711400593777,
0.00290517547569836));
#50549=CARTESIAN_POINT('Ctrl Pts',(-0.0336183971299517,0.0117157849409566,
0.00289651104597295));
#50550=CARTESIAN_POINT('Ctrl Pts',(-0.0336599369421521,0.0117270112572004,
0.00287432538772449));
#50551=CARTESIAN_POINT('Ctrl Pts',(-0.0337033263306569,0.0117386749950227,
0.00285109918914621));
#50552=CARTESIAN_POINT('Ctrl Pts',(-0.0337432769783829,0.0117493627271154,
0.00282965588400019));
#50553=CARTESIAN_POINT('Ctrl Pts',(-0.033783227626109,0.0117600504592081,
0.00280821257885418));
#50554=CARTESIAN_POINT('Ctrl Pts',(-0.0338197408500964,0.0117697936031173,
0.002788570552052));
#50555=CARTESIAN_POINT('Ctrl Pts',(-0.0338738318307421,0.0117840620682984,
0.00275943958532525));
#50556=CARTESIAN_POINT('Ctrl Pts',(-0.0339053976158736,0.0117923886931939,
0.00274243967470438));
#50557=CARTESIAN_POINT('Ctrl Pts',(-0.0339429792784883,0.0118022560787779,
0.00272217110902682));
#50558=CARTESIAN_POINT('Ctrl Pts',(-0.0339811690594926,0.0118121985860684,
0.00270155561106871));
#50559=CARTESIAN_POINT('Ctrl Pts',(-0.0340084211072455,0.0118192935124163,
0.00268684448887767));
#50560=CARTESIAN_POINT('Ctrl Pts',(-0.0340359888280535,0.0118264291801899,
0.00267195442002909));
#50561=CARTESIAN_POINT('Ctrl Pts',(-0.0340619844400523,0.0118331194661837,
0.00265790946211028));
#50562=CARTESIAN_POINT('Ctrl Pts',(-0.0341587801244567,0.0118580310093955,
0.00260561250852268));
#50563=CARTESIAN_POINT('Ctrl Pts',(-0.0342355350435881,0.011877303956768,
0.00256410000912341));
#50564=CARTESIAN_POINT('Ctrl Pts',(-0.0343090494548926,0.0118954720904133,
0.00252436942052295));
#50565=CARTESIAN_POINT('Ctrl Pts',(-0.034377765982074,0.0119124544892019,
0.00248723183044974));
#50566=CARTESIAN_POINT('Ctrl Pts',(-0.034440217823129,0.0119275695818341,
0.00245350394200026));
#50567=CARTESIAN_POINT('Ctrl Pts',(-0.0344945167249313,0.0119405224469314,
0.00242421468177289));
#50568=CARTESIAN_POINT('Ctrl Pts',(-0.0346443687635191,0.0119762692700891,
0.00234338329829906));
#50569=CARTESIAN_POINT('Ctrl Pts',(-0.0347320363953884,0.0119958065028771,
0.00229639230335554));
#50570=CARTESIAN_POINT('Ctrl Pts',(-0.034761114924408,0.0120023525649548,
0.00228080342275955));
#50571=CARTESIAN_POINT('Ctrl Pts',(-0.0347611149244081,0.0120023525649548,
0.00228080342275953));
#50572=CARTESIAN_POINT('Ctrl Pts',(-0.0350057465916318,0.0120574232361325,
0.00214965738323656));
#50573=CARTESIAN_POINT('Ctrl Pts',(-0.0352219305060277,0.0121119430756711,
0.00201136019321215));
#50574=CARTESIAN_POINT('Ctrl Pts',(-0.0354113877997593,0.0121652746629532,
0.00186094727113069));
#50575=CARTESIAN_POINT('Ctrl Pts',(-0.035506116446625,0.0121919404565942,
0.00178574081008997));
#50576=CARTESIAN_POINT('Ctrl Pts',(-0.0355941613778847,0.0122182229392589,
0.00170746180636983));
#50577=CARTESIAN_POINT('Ctrl Pts',(-0.0356727119988853,0.0122425351472171,
0.00163017986048025));
#50578=CARTESIAN_POINT('Ctrl Pts',(-0.035751262619886,0.0122668473551753,
0.00155289791459067));
#50579=CARTESIAN_POINT('Ctrl Pts',(-0.0358203219212352,0.0122894914949874,
0.00147671829736536));
#50580=CARTESIAN_POINT('Ctrl Pts',(-0.0358906376015656,0.0123143053868271,
0.00138469040033681));
#50581=CARTESIAN_POINT('Ctrl Pts',(-0.0359459581526986,0.0123338276067057,
0.00131228785855225));
#50582=CARTESIAN_POINT('Ctrl Pts',(-0.0360023350087833,0.0123544331983604,
0.0012299870285152));
#50583=CARTESIAN_POINT('Ctrl Pts',(-0.0360519439610623,0.0123733252959181,
0.00114522311741257));
#50584=CARTESIAN_POINT('Ctrl Pts',(-0.0360653909104063,0.0123784461675993,
0.00112224710267254));
#50585=CARTESIAN_POINT('Ctrl Pts',(-0.0360783784191254,0.0123834476159398,
0.00109909132918738));
#50586=CARTESIAN_POINT('Ctrl Pts',(-0.0360908073487765,0.0123882936272754,
0.00107590835554495));
#50587=CARTESIAN_POINT('Ctrl Pts',(-0.0361490895171189,0.0124110177118409,
0.000967197950833359));
#50588=CARTESIAN_POINT('Ctrl Pts',(-0.0361957250440342,0.012430415454159,
0.000858097457749819));
#50589=CARTESIAN_POINT('Ctrl Pts',(-0.0362335563872392,0.0124469446125988,
0.000743163630492097));
#50590=CARTESIAN_POINT('Ctrl Pts',(-0.0362517959565832,0.0124549137912221,
0.000687750754959665));
#50591=CARTESIAN_POINT('Ctrl Pts',(-0.0362680632461128,0.0124621879064148,
0.000630954362927607));
#50592=CARTESIAN_POINT('Ctrl Pts',(-0.0362821925945658,0.0124686133356257,
0.00057313845736941));
#50593=CARTESIAN_POINT('Ctrl Pts',(-0.0363266756201778,0.0124888423315418,
0.000391118287346746));
#50594=CARTESIAN_POINT('Ctrl Pts',(-0.036349052138052,0.0125003225965748,
0.000198997572025257));
#50595=CARTESIAN_POINT('Ctrl Pts',(-0.0363499678593351,0.0125005306980164,
7.1125461161381E-6));
#50596=CARTESIAN_POINT('Ctrl Pts',(-0.0363509068618171,0.0125007440902066,
-0.000189650943952258));
#50597=CARTESIAN_POINT('Ctrl Pts',(-0.0363293598144398,0.0124891685314849,
-0.000386265257023896));
#50598=CARTESIAN_POINT('Ctrl Pts',(-0.03628465461844,0.0124684484641288,
-0.000572491284554948));
#50599=CARTESIAN_POINT('Ctrl Pts',(-0.0362719151674783,0.0124625439540131,
-0.00062555932938664));
#50600=CARTESIAN_POINT('Ctrl Pts',(-0.0362573645944939,0.0124559208607803,
-0.000677787987754251));
#50601=CARTESIAN_POINT('Ctrl Pts',(-0.0362410960019726,0.0124486802760739,
-0.000728972235372414));
#50602=CARTESIAN_POINT('Ctrl Pts',(-0.0362044168877487,0.0124323556780397,
-0.00084437206866398));
#50603=CARTESIAN_POINT('Ctrl Pts',(-0.036158683752071,0.0124130217471169,
-0.000954369431566533));
#50604=CARTESIAN_POINT('Ctrl Pts',(-0.0361014308319117,0.0123903467940526,
-0.00106374449995132));
#50605=CARTESIAN_POINT('Ctrl Pts',(-0.0360874771524456,0.012384820455377,
-0.00109040138734813));
#50606=CARTESIAN_POINT('Ctrl Pts',(-0.0360727920550754,0.0123790911585592,
-0.00111700811362443));
#50607=CARTESIAN_POINT('Ctrl Pts',(-0.0360575232042416,0.0123732120918076,
-0.00114334700138639));
#50608=CARTESIAN_POINT('Ctrl Pts',(-0.0360101428950575,0.0123549689375955,
-0.00122507840732604));
#50609=CARTESIAN_POINT('Ctrl Pts',(-0.0359567194207932,0.0123352136600716,
-0.00130421953635196));
#50610=CARTESIAN_POINT('Ctrl Pts',(-0.03590398794558,0.0123163797963791,
-0.00137439251461595));
#50611=CARTESIAN_POINT('Ctrl Pts',(-0.035834263144592,0.0122914765029953,
-0.00146717954407812));
#50612=CARTESIAN_POINT('Ctrl Pts',(-0.0357652787954704,0.0122685831489911,
-0.00154443052208826));
#50613=CARTESIAN_POINT('Ctrl Pts',(-0.0356867706045274,0.0122440124521361,
-0.0016226400606878));
#50614=CARTESIAN_POINT('Ctrl Pts',(-0.0356082624135844,0.0122194417552811,
-0.00170084959928734));
#50615=CARTESIAN_POINT('Ctrl Pts',(-0.0355202275951528,0.012192895300252,
-0.00177991418021254));
#50616=CARTESIAN_POINT('Ctrl Pts',(-0.0354253661890923,0.0121659334521712,
-0.00185587673631822));
#50617=CARTESIAN_POINT('Ctrl Pts',(-0.0352356433769715,0.0121120097560096,
-0.00200780184852956));
#50618=CARTESIAN_POINT('Ctrl Pts',(-0.0350186221148744,0.0120567658180567,
-0.00214749180977129));
#50619=CARTESIAN_POINT('Ctrl Pts',(-0.0347727610542622,0.012000956525018,
-0.00227981334747214));
#50620=CARTESIAN_POINT('Ctrl Pts',(-0.04,0.00410701437367704,-0.00382361007903213));
#50621=CARTESIAN_POINT('Ctrl Pts',(-0.0301131479141235,0.00410701437367704,
-0.00382361007903213));
#50622=CARTESIAN_POINT('Ctrl Pts',(-0.0242064812039311,0.00227260406699975,
-0.00565754282198516));
#50623=CARTESIAN_POINT('Ctrl Pts',(-0.0150880182599324,0.00043817569586083,
-0.0102482507131694));
#50624=CARTESIAN_POINT('Ctrl Pts',(-0.04,0.00441551938950954,-0.00399865527756543));
#50625=CARTESIAN_POINT('Ctrl Pts',(-0.03014220946428,0.00441551938950954,
-0.00399865527756543));
#50626=CARTESIAN_POINT('Ctrl Pts',(-0.0242279866368223,0.00277049415159215,
-0.00567110613607142));
#50627=CARTESIAN_POINT('Ctrl Pts',(-0.0151029086749286,0.00112545046390722,
-0.0102394484928933));
#50628=CARTESIAN_POINT('Ctrl Pts',(-0.04,0.00472402440534204,-0.00417370047609873));
#50629=CARTESIAN_POINT('Ctrl Pts',(-0.0301712710144365,0.00472402440534204,
-0.00417370047609873));
#50630=CARTESIAN_POINT('Ctrl Pts',(-0.0242494920697135,0.00326838423618455,
-0.00568466945015768));
#50631=CARTESIAN_POINT('Ctrl Pts',(-0.0151177990899248,0.00181272523195361,
-0.0102306462726171));
#50632=CARTESIAN_POINT('Ctrl Pts',(-0.04,0.00503252942117453,-0.00434874567463202));
#50633=CARTESIAN_POINT('Ctrl Pts',(-0.030200332564593,0.00503252942117453,
-0.00434874567463202));
#50634=CARTESIAN_POINT('Ctrl Pts',(-0.0242709975026047,0.00376627432077694,
-0.00569823276424395));
#50635=CARTESIAN_POINT('Ctrl Pts',(-0.015132689504921,0.0025,-0.0102218440523409));
#50636=CARTESIAN_POINT('Ctrl Pts',(-0.04,0.00521956265744013,-0.00445486800099385));
#50637=CARTESIAN_POINT('Ctrl Pts',(-0.0302179513244113,0.00521956265744013,
-0.00445486800099385));
#50638=CARTESIAN_POINT('Ctrl Pts',(-0.0242840353156208,0.00406812352596598,
-0.00570645561443391));
#50639=CARTESIAN_POINT('Ctrl Pts',(-0.0151417169189439,0.00291666494051817,
-0.0102165076472256));
#50640=CARTESIAN_POINT('Ctrl Pts',(-0.04,0.00560724895560903,-0.00464290068538419));
#50641=CARTESIAN_POINT('Ctrl Pts',(-0.0302531888727876,0.00560724895560903,
-0.00464290068538419));
#50642=CARTESIAN_POINT('Ctrl Pts',(-0.0243101706144599,0.00467874072064833,
-0.00571926407880603));
#50643=CARTESIAN_POINT('Ctrl Pts',(-0.0151597764656002,0.00375021261144434,
-0.0102058320476674));
#50644=CARTESIAN_POINT('Ctrl Pts',(-0.04,0.00622010312641127,-0.00484777123182973));
#50645=CARTESIAN_POINT('Ctrl Pts',(-0.030289515056412,0.00622010312641127,
-0.00484777123182973));
#50646=CARTESIAN_POINT('Ctrl Pts',(-0.0243413031901115,0.00561041051155431,
-0.00572840549436799));
#50647=CARTESIAN_POINT('Ctrl Pts',(-0.0151868693264875,0.00500069755002587,
-0.0101898165551843));
#50648=CARTESIAN_POINT('Ctrl Pts',(-0.04,0.00685442072891309,-0.00497216498332829));
#50649=CARTESIAN_POINT('Ctrl Pts',(-0.0303161560626962,0.00685442072891309,
-0.00497216498332829));
#50650=CARTESIAN_POINT('Ctrl Pts',(-0.0243678035878454,0.00655264832435518,
-0.00572893819065769));
#50651=CARTESIAN_POINT('Ctrl Pts',(-0.0152139550980222,0.00625085527589332,
-0.0101738052534537));
#50652=CARTESIAN_POINT('Ctrl Pts',(-0.04,0.00728473228062269,-0.005));
#50653=CARTESIAN_POINT('Ctrl Pts',(-0.0303257372905531,0.00728471479311311,
-0.005));
#50654=CARTESIAN_POINT('Ctrl Pts',(-0.0243815314752158,0.00718424112369502,
-0.005724907257076));
#50655=CARTESIAN_POINT('Ctrl Pts',(-0.015232000484084,0.00708374935728818,
-0.0101631380246945));
#50656=CARTESIAN_POINT('Ctrl Pts',(-0.04,0.00749999999999979,-0.005));
#50657=CARTESIAN_POINT('Ctrl Pts',(-0.0303290418474347,0.0075,-0.005));
#50658=CARTESIAN_POINT('Ctrl Pts',(-0.0243876928299813,0.0075,-0.00572224175535161));
#50659=CARTESIAN_POINT('Ctrl Pts',(-0.0152410184731965,0.00749997928621807,
-0.0101578071909577));
#50660=CARTESIAN_POINT('',(-0.0153166288848674,0.00749997934066271,-0.0101211250654636));
#50661=CARTESIAN_POINT('',(-0.0152002984431706,0.00249860370283979,-0.0101883828166932));
#50662=CARTESIAN_POINT('Ctrl Pts',(-0.015200302987251,0.00249860372052335,
-0.010188391982339));
#50663=CARTESIAN_POINT('Ctrl Pts',(-0.0152383462555177,0.00403177811962914,
-0.0101665731553613));
#50664=CARTESIAN_POINT('Ctrl Pts',(-0.0152771294947074,0.00569890335868286,
-0.010144166971735));
#50665=CARTESIAN_POINT('Ctrl Pts',(-0.0153166288848674,0.00749997934066271,
-0.0101211250654636));
#50666=CARTESIAN_POINT('',(-0.0151728897383989,0.00139471190135993,-0.0102040357394328));
#50667=CARTESIAN_POINT('',(-0.0151728647969064,0.0013947315415857,-0.0102039854802522));
#50668=CARTESIAN_POINT('',(-0.0264247148113527,0.00412797976408685,-0.00580905681399726));
#50669=CARTESIAN_POINT('Ctrl Pts',(-0.015172889738406,0.00139471190135982,
-0.0102040357394293));
#50670=CARTESIAN_POINT('Ctrl Pts',(-0.0153640466907317,0.00139164697469342,
-0.0101088087777892));
#50671=CARTESIAN_POINT('Ctrl Pts',(-0.0155523144542564,0.00138937495703902,
-0.010015498686153));
#50672=CARTESIAN_POINT('Ctrl Pts',(-0.0157270793130222,0.00138796132752518,
-0.00992929088300855));
#50673=CARTESIAN_POINT('Ctrl Pts',(-0.0158387317023676,0.00138705819909317,
-0.00987421512424748));
#50674=CARTESIAN_POINT('Ctrl Pts',(-0.0159421944236299,0.00138650141184947,
-0.00982334442246595));
#50675=CARTESIAN_POINT('Ctrl Pts',(-0.016044808187784,0.00138620424068754,
-0.00977303537098498));
#50676=CARTESIAN_POINT('Ctrl Pts',(-0.0161409303235507,0.00138592586938902,
-0.00972590900819523));
#50677=CARTESIAN_POINT('Ctrl Pts',(-0.016241951248696,0.00138584744702312,
-0.0096765029580068));
#50678=CARTESIAN_POINT('Ctrl Pts',(-0.0163580264003874,0.00138615564543367,
-0.00961995244320662));
#50679=CARTESIAN_POINT('Ctrl Pts',(-0.0164981544591239,0.00138652770822528,
-0.00955168362129225));
#50680=CARTESIAN_POINT('Ctrl Pts',(-0.0166503211155925,0.001387535621787,
-0.0094778791870578));
#50681=CARTESIAN_POINT('Ctrl Pts',(-0.0167914691573054,0.00138908714879256,
-0.00940974092434808));
#50682=CARTESIAN_POINT('Ctrl Pts',(-0.0169946940172579,0.00139132103638031,
-0.00931163549738969));
#50683=CARTESIAN_POINT('Ctrl Pts',(-0.0171844689503031,0.00139465213309412,
-0.00922066972026411));
#50684=CARTESIAN_POINT('Ctrl Pts',(-0.0173610695246576,0.001398705432113,
-0.00913648779519181));
#50685=CARTESIAN_POINT('Ctrl Pts',(-0.017480860043453,0.0014014548387561,
-0.00907938607559399));
#50686=CARTESIAN_POINT('Ctrl Pts',(-0.0175941508771455,0.00140451717652119,
-0.00902560988865672));
#50687=CARTESIAN_POINT('Ctrl Pts',(-0.0177050956254356,0.00140798029570822,
-0.00897315003992925));
#50688=CARTESIAN_POINT('Ctrl Pts',(-0.017772581403461,0.00141008685141575,
-0.00894123961820105));
#50689=CARTESIAN_POINT('Ctrl Pts',(-0.0178405165978862,0.00141240430644739,
-0.00890920270627398));
#50690=CARTESIAN_POINT('Ctrl Pts',(-0.0178988704357995,0.00141453537558346,
-0.00888174239928231));
#50691=CARTESIAN_POINT('Ctrl Pts',(-0.0179464182169222,0.00141627180993745,
-0.00885936723574392));
#50692=CARTESIAN_POINT('Ctrl Pts',(-0.0179891513800797,0.00141789221730591,
-0.00883928301160839));
#50693=CARTESIAN_POINT('Ctrl Pts',(-0.0180512194881658,0.00142043815040328,
-0.0088101886104058));
#50694=CARTESIAN_POINT('Ctrl Pts',(-0.0181250746488341,0.00142346756927483,
-0.00877556903295086));
#50695=CARTESIAN_POINT('Ctrl Pts',(-0.0182194266673454,0.00142766991273628,
-0.00873147419872672));
#50696=CARTESIAN_POINT('Ctrl Pts',(-0.0183003383205456,0.00143163411086214,
-0.00869379760743843));
#50697=CARTESIAN_POINT('Ctrl Pts',(-0.0184171707451642,0.00143735821685176,
-0.00863939447343388));
#50698=CARTESIAN_POINT('Ctrl Pts',(-0.0185254060865838,0.00144331181171606,
-0.00858924034070737));
#50699=CARTESIAN_POINT('Ctrl Pts',(-0.0186347757749826,0.00144997327833353,
-0.00853878889151528));
#50700=CARTESIAN_POINT('Ctrl Pts',(-0.018693175629497,0.0014535302847309,
-0.00851184945942952));
#50701=CARTESIAN_POINT('Ctrl Pts',(-0.0187510592544907,0.0014572490992189,
-0.00848521670979728));
#50702=CARTESIAN_POINT('Ctrl Pts',(-0.0188082658532537,0.00146111809363485,
-0.00845896220693822));
#50703=CARTESIAN_POINT('Ctrl Pts',(-0.0189299079947893,0.00146934499012099,
-0.00840313553620804));
#50704=CARTESIAN_POINT('Ctrl Pts',(-0.0190484922899703,0.00147829167063493,
-0.00834903053934462));
#50705=CARTESIAN_POINT('Ctrl Pts',(-0.0191557127031988,0.00148709445690661,
-0.00830034702239981));
#50706=CARTESIAN_POINT('Ctrl Pts',(-0.0192629331164272,0.00149589724317828,
-0.00825166350545499));
#50707=CARTESIAN_POINT('Ctrl Pts',(-0.0193587928518425,0.00150422786878183,
-0.00820832664749509));
#50708=CARTESIAN_POINT('Ctrl Pts',(-0.019478661225813,0.00151594892376546,
-0.00815447593113739));
#50709=CARTESIAN_POINT('Ctrl Pts',(-0.0195350531068573,0.00152146307496695,
-0.00812914194945058));
#50710=CARTESIAN_POINT('Ctrl Pts',(-0.0195967582311657,0.00152771365395053,
-0.00810149537074743));
#50711=CARTESIAN_POINT('Ctrl Pts',(-0.0196600682347633,0.00153443781289968,
-0.00807322828599476));
#50712=CARTESIAN_POINT('Ctrl Pts',(-0.0197313319862307,0.00154200673984564,
-0.00804140995732551));
#50713=CARTESIAN_POINT('Ctrl Pts',(-0.0198046286135981,0.00155018308598661,
-0.00800880776207714));
#50714=CARTESIAN_POINT('Ctrl Pts',(-0.0198746319117117,0.00155840063442004,
-0.00797779417403623));
#50715=CARTESIAN_POINT('Ctrl Pts',(-0.020040699008046,0.00157789492174793,
-0.00790422140458601));
#50716=CARTESIAN_POINT('Ctrl Pts',(-0.020189696337606,0.00159751834165863,
-0.00783885656312635));
#50717=CARTESIAN_POINT('Ctrl Pts',(-0.0203399517608801,0.00161942796698918,
-0.00777356369181081));
#50718=CARTESIAN_POINT('Ctrl Pts',(-0.0204627449085639,0.00163733315670072,
-0.00772020443851101));
#50719=CARTESIAN_POINT('Ctrl Pts',(-0.0205803987442986,0.00165603419083452,
-0.00766953351201657));
#50720=CARTESIAN_POINT('Ctrl Pts',(-0.0206899501216064,0.00167476087238793,
-0.00762273306682818));
#50721=CARTESIAN_POINT('Ctrl Pts',(-0.0207880478009765,0.00169152966204479,
-0.00758082565151955));
#50722=CARTESIAN_POINT('Ctrl Pts',(-0.0208861318571135,0.0017092486297667,
-0.00753920099683491));
#50723=CARTESIAN_POINT('Ctrl Pts',(-0.0210010048825742,0.0017317941529701,
-0.00749096649832249));
#50724=CARTESIAN_POINT('Ctrl Pts',(-0.02113621012128,0.00175833017249457,
-0.00743419462469013));
#50725=CARTESIAN_POINT('Ctrl Pts',(-0.0212846632902717,0.00179016196917818,
-0.00737263337366511));
#50726=CARTESIAN_POINT('Ctrl Pts',(-0.021419463383592,0.00182188843346957,
-0.00731753419372364));
#50727=CARTESIAN_POINT('Ctrl Pts',(-0.0215086395923106,0.00184287688927745,
-0.00728108365537715));
#50728=CARTESIAN_POINT('Ctrl Pts',(-0.0215942891562261,0.00186422684960349,
-0.00724641235429145));
#50729=CARTESIAN_POINT('Ctrl Pts',(-0.0216779850746412,0.00188622057174032,
-0.00721285036718868));
#50730=CARTESIAN_POINT('Ctrl Pts',(-0.021765752732351,0.00190928427081698,
-0.00717765561633489));
#50731=CARTESIAN_POINT('Ctrl Pts',(-0.0218514083708002,0.00193287245044484,
-0.00714365232694369));
#50732=CARTESIAN_POINT('Ctrl Pts',(-0.0219362391982793,0.00195743414150113,
-0.00711033167457065));
#50733=CARTESIAN_POINT('Ctrl Pts',(-0.0220774356881042,0.00199831579578145,
-0.00705487118581248));
#50734=CARTESIAN_POINT('Ctrl Pts',(-0.0222163758277559,0.00204183958808548,
-0.007001269044706));
#50735=CARTESIAN_POINT('Ctrl Pts',(-0.0223589628768257,0.00209034777808599,
-0.00694744377558152));
#50736=CARTESIAN_POINT('Ctrl Pts',(-0.0225872162011364,0.00216799968052833,
-0.00686128029376652));
#50737=CARTESIAN_POINT('Ctrl Pts',(-0.0228248207747851,0.00225873667442951,
-0.00677476643823198));
#50738=CARTESIAN_POINT('Ctrl Pts',(-0.0230511297423702,0.00235518715086805,
-0.0066960403563144));
#50739=CARTESIAN_POINT('Ctrl Pts',(-0.0231077069842665,0.00237929976997769,
-0.006676358835835));
#50740=CARTESIAN_POINT('Ctrl Pts',(-0.0231635748117954,0.00240377040747212,
-0.00665715528197924));
#50741=CARTESIAN_POINT('Ctrl Pts',(-0.023219476345564,0.0024289001944486,
-0.00663817707029671));
#50742=CARTESIAN_POINT('Ctrl Pts',(-0.0232753778793326,0.00245402998142509,
-0.00661919885861419));
#50743=CARTESIAN_POINT('Ctrl Pts',(-0.0233313130972234,0.0024798189490564,
-0.00660044587602993));
#50744=CARTESIAN_POINT('Ctrl Pts',(-0.0233880311148421,0.00250656652116927,
-0.00658168097578289));
#50745=CARTESIAN_POINT('Ctrl Pts',(-0.0235014671500793,0.00256006166539502,
-0.00654415117528881));
#50746=CARTESIAN_POINT('Ctrl Pts',(-0.0236180513149816,0.00261738621136591,
-0.00650661794344506));
#50747=CARTESIAN_POINT('Ctrl Pts',(-0.0237278917023892,0.00267334490073194,
-0.00647224236002402));
#50748=CARTESIAN_POINT('Ctrl Pts',(-0.0238338075057732,0.00272730419275926,
-0.00643909501212436));
#50749=CARTESIAN_POINT('Ctrl Pts',(-0.0239334197217683,0.00278000891741973,
-0.00640881009814871));
#50750=CARTESIAN_POINT('Ctrl Pts',(-0.0240375209246323,0.00283607172543691,
-0.00637800229702447));
#50751=CARTESIAN_POINT('Ctrl Pts',(-0.0240413782707934,0.00283814906605682,
-0.00637686075062412));
#50752=CARTESIAN_POINT('Ctrl Pts',(-0.0240452417268192,0.00284023114535695,
-0.00637571858570592));
#50753=CARTESIAN_POINT('Ctrl Pts',(-0.0240491118410187,0.00284231820402006,
-0.00637457564477758));
#50754=CARTESIAN_POINT('Ctrl Pts',(-0.0241032697900432,0.00287152427155755,
-0.0063585814561453));
#50755=CARTESIAN_POINT('Ctrl Pts',(-0.0241587067718473,0.00290175501435321,
-0.00634244114415675));
#50756=CARTESIAN_POINT('Ctrl Pts',(-0.0242188370468896,0.00293500164702928,
-0.00632525504927828));
#50757=CARTESIAN_POINT('Ctrl Pts',(-0.0242822586570924,0.00297006809195497,
-0.00630712824361301));
#50758=CARTESIAN_POINT('Ctrl Pts',(-0.0243507542959291,0.00300850547177018,
-0.00628796647954365));
#50759=CARTESIAN_POINT('Ctrl Pts',(-0.0244026806904869,0.00303785624166982,
-0.00627365709734696));
#50760=CARTESIAN_POINT('Ctrl Pts',(-0.0244609125934436,0.00307077112434273,
-0.00625761010308629));
#50761=CARTESIAN_POINT('Ctrl Pts',(-0.0245027620972734,0.00309461595014579,
-0.00624626073921518));
#50762=CARTESIAN_POINT('Ctrl Pts',(-0.0245606802234146,0.00312774433649193,
-0.00623079155141568));
#50763=CARTESIAN_POINT('Ctrl Pts',(-0.024598014513208,0.00314909904629757,
-0.00622082004199969));
#50764=CARTESIAN_POINT('Ctrl Pts',(-0.0246394426369129,0.00317286623215922,
-0.00620987083642133));
#50765=CARTESIAN_POINT('Ctrl Pts',(-0.0246820683894351,0.00319736290427895,
-0.00619875383540347));
#50766=CARTESIAN_POINT('Ctrl Pts',(-0.0247868163902898,0.00325756072555608,
-0.00617143505360567));
#50767=CARTESIAN_POINT('Ctrl Pts',(-0.0248987288283024,0.00332221997852365,
-0.00614300928379103));
#50768=CARTESIAN_POINT('Ctrl Pts',(-0.0250319267246202,0.00339816141664959,
-0.0061105002291567));
#50769=CARTESIAN_POINT('Ctrl Pts',(-0.025040910428721,0.00340328338499874,
-0.00610830761399155));
#50770=CARTESIAN_POINT('Ctrl Pts',(-0.0250499912615901,0.00340845601431403,
-0.00610609669903062));
#50771=CARTESIAN_POINT('Ctrl Pts',(-0.0250591736190017,0.00341368127427967,
-0.00610386674487505));
#50772=CARTESIAN_POINT('Ctrl Pts',(-0.0251318364236611,0.00345503035569324,
-0.00608622043511567));
#50773=CARTESIAN_POINT('Ctrl Pts',(-0.025210875135261,0.00349968439401741,
-0.00606743730546045));
#50774=CARTESIAN_POINT('Ctrl Pts',(-0.0252803579825825,0.00353851440133161,
-0.00605123333538441));
#50775=CARTESIAN_POINT('Ctrl Pts',(-0.0253765429748567,0.00359226671715477,
-0.00602880220602436));
#50776=CARTESIAN_POINT('Ctrl Pts',(-0.0254566923453874,0.0036363488594505,
-0.0060106534133979));
#50777=CARTESIAN_POINT('Ctrl Pts',(-0.0255299124417394,0.0036761538151833,
-0.00599432966967733));
#50778=CARTESIAN_POINT('Ctrl Pts',(-0.0255790076456114,0.00370284365191094,
-0.00598338434775283));
#50779=CARTESIAN_POINT('Ctrl Pts',(-0.0256196248685335,0.00372468467997514,
-0.00597446684985712));
#50780=CARTESIAN_POINT('Ctrl Pts',(-0.0256528411804496,0.0037424500534779,
-0.00596722158133266));
#50781=CARTESIAN_POINT('Ctrl Pts',(-0.0256841652496382,0.00375920338208849,
-0.00596038905600223));
#50782=CARTESIAN_POINT('Ctrl Pts',(-0.0257148294720635,0.00377554739889252,
-0.00595373195874594));
#50783=CARTESIAN_POINT('Ctrl Pts',(-0.0257622051350364,0.00380048230091671,
-0.00594359467047805));
#50784=CARTESIAN_POINT('Ctrl Pts',(-0.0258061642031996,0.00382361897044148,
-0.00593418845391045));
#50785=CARTESIAN_POINT('Ctrl Pts',(-0.0258599297734075,0.00385162737452401,
-0.00592281763862265));
#50786=CARTESIAN_POINT('Ctrl Pts',(-0.0259087270781427,0.00387670604391645,
-0.00591263710437559));
#50787=CARTESIAN_POINT('Ctrl Pts',(-0.0259536558801419,0.0038997965522478,
-0.00590326365209347));
#50788=CARTESIAN_POINT('Ctrl Pts',(-0.0259943389037606,0.00392045407114615,
-0.00589487706119322));
#50789=CARTESIAN_POINT('Ctrl Pts',(-0.0260350849839353,0.0039408431970337,
-0.00588654105989476));
#50790=CARTESIAN_POINT('Ctrl Pts',(-0.0260488265955664,0.00394771942778381,
-0.00588372974425634));
#50791=CARTESIAN_POINT('Ctrl Pts',(-0.0260625759974508,0.00395456380062419,
-0.0058809247125566));
#50792=CARTESIAN_POINT('Ctrl Pts',(-0.0260764997386049,0.00396145957792697,
-0.00587809239311163));
#50793=CARTESIAN_POINT('Ctrl Pts',(-0.0261869194675372,0.00401614530154976,
-0.00585563119235378));
#50794=CARTESIAN_POINT('Ctrl Pts',(-0.0263081686292907,0.00407431886964289,
-0.00583164341641599));
#50795=CARTESIAN_POINT('Ctrl Pts',(-0.0264247242280828,0.00412797324082191,
-0.00580908996388195));
#50796=CARTESIAN_POINT('',(-0.0328171231859669,0.00544959481071556,-0.00491819439550167));
#50797=CARTESIAN_POINT('Ctrl Pts',(-0.0264247148113527,0.00412797976408685,
-0.00580905681399726));
#50798=CARTESIAN_POINT('Ctrl Pts',(-0.0266806623606955,0.004265817161036,
-0.00576358983715232));
#50799=CARTESIAN_POINT('Ctrl Pts',(-0.0271941586176829,0.00451878908321525,
-0.00567666122695133));
#50800=CARTESIAN_POINT('Ctrl Pts',(-0.0279187082618112,0.00481814426352985,
-0.00556288680148345));
#50801=CARTESIAN_POINT('Ctrl Pts',(-0.0287529968670884,0.00509216436953578,
-0.00544119748457045));
#50802=CARTESIAN_POINT('Ctrl Pts',(-0.0293995276465761,0.00524409592488056,
-0.00535269372197882));
#50803=CARTESIAN_POINT('Ctrl Pts',(-0.0298940640370636,0.0053307414006189,
-0.00528612781180627));
#50804=CARTESIAN_POINT('Ctrl Pts',(-0.0304875804327081,0.00541300424438409,
-0.0052085859306323));
#50805=CARTESIAN_POINT('Ctrl Pts',(-0.0311383125186733,0.00547351091878673,
-0.00512782359057905));
#50806=CARTESIAN_POINT('Ctrl Pts',(-0.0320222448303377,0.00549729197974687,
-0.00502013830682495));
#50807=CARTESIAN_POINT('Ctrl Pts',(-0.032554724307738,0.00547129131445063,
-0.00495300644550675));
#50808=CARTESIAN_POINT('Ctrl Pts',(-0.0328171226451392,0.0054495948957978,
-0.00491819447958816));
#50809=CARTESIAN_POINT('Ctrl Pts',(-0.0399999990786919,0.00503253317335571,
-0.00434874780361082));
#50810=CARTESIAN_POINT('Ctrl Pts',(-0.0398079283434003,0.00503365259361514,
-0.00434938296194158));
#50811=CARTESIAN_POINT('Ctrl Pts',(-0.0396323617472513,0.00503489684903665,
-0.00435089211560653));
#50812=CARTESIAN_POINT('Ctrl Pts',(-0.0394783469992459,0.00503629893077916,
-0.00435286393834884));
#50813=CARTESIAN_POINT('Ctrl Pts',(-0.0393243322512405,0.00503770101252167,
-0.00435483576109114));
#50814=CARTESIAN_POINT('Ctrl Pts',(-0.0391918691385965,0.00503927926839014,
-0.00435723757858893));
#50815=CARTESIAN_POINT('Ctrl Pts',(-0.0390658193474297,0.00504149043886893,
-0.00436023263436879));
#50816=CARTESIAN_POINT('Ctrl Pts',(-0.0390027944518462,0.00504259602410833,
-0.00436173016225873));
#50817=CARTESIAN_POINT('Ctrl Pts',(-0.0389413729181224,0.00504386058504307,
-0.00436337471752688));
#50818=CARTESIAN_POINT('Ctrl Pts',(-0.0388715003915693,0.00504548027850166,
-0.00436546028537351));
#50819=CARTESIAN_POINT('Ctrl Pts',(-0.0388016278650162,0.00504709997196025,
-0.00436754585322015));
#50820=CARTESIAN_POINT('Ctrl Pts',(-0.0387233046123729,0.00504906597787632,
-0.00437008823748018));
#50821=CARTESIAN_POINT('Ctrl Pts',(-0.0386461502734439,0.00505118109228873,
-0.0043728342611483));
#50822=CARTESIAN_POINT('Ctrl Pts',(-0.0384918415955858,0.00505541132111354,
-0.00437832630848453));
#50823=CARTESIAN_POINT('Ctrl Pts',(-0.0383422076850759,0.00506025879694506,
-0.00438459512348587));
#50824=CARTESIAN_POINT('Ctrl Pts',(-0.0381946501383217,0.00506566602230368,
-0.00439158507208406));
#50825=CARTESIAN_POINT('Ctrl Pts',(-0.0378995350448133,0.00507648047302089,
-0.00440556496928044));
#50826=CARTESIAN_POINT('Ctrl Pts',(-0.0376127246200382,0.00508955164697904,
-0.00442239696763909));
#50827=CARTESIAN_POINT('Ctrl Pts',(-0.0373174662030721,0.00510514094597655,
-0.00444258389671857));
#50828=CARTESIAN_POINT('Ctrl Pts',(-0.0371698369945891,0.00511293559547531,
-0.00445267736125831));
#50829=CARTESIAN_POINT('Ctrl Pts',(-0.0370200961537913,0.00512135807816629,
-0.00446361373187541));
#50830=CARTESIAN_POINT('Ctrl Pts',(-0.0368619128206017,0.00513094709709688,
-0.00447600706817314));
#50831=CARTESIAN_POINT('Ctrl Pts',(-0.0367037294874121,0.00514053611602746,
-0.00448840040447088));
#50832=CARTESIAN_POINT('Ctrl Pts',(-0.036537106172115,0.00515126175938117,
-0.00450230894043891));
#50833=CARTESIAN_POINT('Ctrl Pts',(-0.0363950645278357,0.00516076588467846,
-0.00451469899300244));
#50834=CARTESIAN_POINT('Ctrl Pts',(-0.0362530228835564,0.00517027000997575,
-0.00452708904556598));
#50835=CARTESIAN_POINT('Ctrl Pts',(-0.0361355575855477,0.00517860019854412,
-0.00453786216343966));
#50836=CARTESIAN_POINT('Ctrl Pts',(-0.0360038343615319,0.00518824122937477,
-0.00455034475502334));
#50837=CARTESIAN_POINT('Ctrl Pts',(-0.0358721111375161,0.00519788226020543,
-0.00456282734660702));
#50838=CARTESIAN_POINT('Ctrl Pts',(-0.0357261339316059,0.00520880455506361,
-0.00457708358477853));
#50839=CARTESIAN_POINT('Ctrl Pts',(-0.0355774733705788,0.0052202231385025,
-0.00459211847497182));
#50840=CARTESIAN_POINT('Ctrl Pts',(-0.0354288128095516,0.0052316417219414,
-0.00460715336516512));
#50841=CARTESIAN_POINT('Ctrl Pts',(-0.0352774671293249,0.00524356784153638,
-0.00462294121804181));
#50842=CARTESIAN_POINT('Ctrl Pts',(-0.0351160105361898,0.00525659897498482,
-0.00464033438166046));
#50843=CARTESIAN_POINT('Ctrl Pts',(-0.0349545539430548,0.00526963010843325,
-0.00465772754527911));
#50844=CARTESIAN_POINT('Ctrl Pts',(-0.0347829889395164,0.00528375105812449,
-0.00467676133373444));
#50845=CARTESIAN_POINT('Ctrl Pts',(-0.0346194848568192,0.00529730904529849,
-0.0046953590234092));
#50846=CARTESIAN_POINT('Ctrl Pts',(-0.0342924766914248,0.00532442501964648,
-0.00473255440275871));
#50847=CARTESIAN_POINT('Ctrl Pts',(-0.0339976954346225,0.005349370351003,
-0.00476779921072633));
#50848=CARTESIAN_POINT('Ctrl Pts',(-0.0337017730542888,0.00537440420893885,
-0.00480443044263055));
#50849=CARTESIAN_POINT('Ctrl Pts',(-0.0334581371642852,0.00539501483748121,
-0.00483458930650848));
#50850=CARTESIAN_POINT('Ctrl Pts',(-0.033213727355736,0.00541565703700328,
-0.00486576883655851));
#50851=CARTESIAN_POINT('Ctrl Pts',(-0.0329721975600362,0.00543630250710774,
-0.0048976089131913));
#50852=CARTESIAN_POINT('Ctrl Pts',(-0.0329203630568065,0.00544073321381913,
-0.00490444208485144));
#50853=CARTESIAN_POINT('Ctrl Pts',(-0.0328686603418303,0.00544516406868864,
-0.00491130527685778));
#50854=CARTESIAN_POINT('Ctrl Pts',(-0.0328171242669787,0.00544959475255144,
-0.00491819426162666));
#50855=CARTESIAN_POINT('Ctrl Pts',(-0.04,0.00749999999999979,-0.005));
#50856=CARTESIAN_POINT('Ctrl Pts',(-0.0303557247091859,0.0075,-0.005));
#50857=CARTESIAN_POINT('Ctrl Pts',(-0.0244205064310119,0.0075,-0.00571826182059907));
#50858=CARTESIAN_POINT('Ctrl Pts',(-0.0153166543938371,0.00749997945719785,
-0.0101211778088248));
#50859=CARTESIAN_POINT('Ctrl Pts',(-0.04,0.0100485913697267,0.00430251487755884));
#50860=CARTESIAN_POINT('Ctrl Pts',(-0.0301947260752482,0.0100485913697267,
0.00430251487755884));
#50861=CARTESIAN_POINT('Ctrl Pts',(-0.0242897188632192,0.0113547636009066,
0.00566740485375001));
#50862=CARTESIAN_POINT('Ctrl Pts',(-0.015132689504921,0.0126609342369608,
0.0102218440523409));
#50863=CARTESIAN_POINT('Ctrl Pts',(-0.04,0.0100244455634135,0.00431627900887509));
#50864=CARTESIAN_POINT('Ctrl Pts',(-0.0301965679597973,0.0100244455634135,
0.00431627900887509));
#50865=CARTESIAN_POINT('Ctrl Pts',(-0.0242906767905071,0.0113158683097808,
0.0056688196752123));
#50866=CARTESIAN_POINT('Ctrl Pts',(-0.015132689504921,0.0126072894913072,
0.0102218440523409));
#50867=CARTESIAN_POINT('Ctrl Pts',(-0.04,0.0100002997571002,0.00433004314019135));
#50868=CARTESIAN_POINT('Ctrl Pts',(-0.0301984098443463,0.0100002997571002,
0.00433004314019135));
#50869=CARTESIAN_POINT('Ctrl Pts',(-0.0242916347177951,0.0112769730186549,
0.00567023449667458));
#50870=CARTESIAN_POINT('Ctrl Pts',(-0.015132689504921,0.0125536447456536,
0.0102218440523409));
#50871=CARTESIAN_POINT('Ctrl Pts',(-0.04,0.00997615395078692,0.0043438072715076));
#50872=CARTESIAN_POINT('Ctrl Pts',(-0.0302002517288954,0.00997615395078692,
0.0043438072715076));
#50873=CARTESIAN_POINT('Ctrl Pts',(-0.024292592645083,0.011238077727529,
0.00567164931813686));
#50874=CARTESIAN_POINT('Ctrl Pts',(-0.015132689504921,0.0125,0.0102218440523409));
#50875=CARTESIAN_POINT('Ctrl Pts',(-0.04,0.00978860990508501,0.00445071531338999));
#50876=CARTESIAN_POINT('Ctrl Pts',(-0.030214557918366,0.00978860990508501,
0.00445071531338999));
#50877=CARTESIAN_POINT('Ctrl Pts',(-0.0243000330078826,0.0109359722537311,
0.00568263844550496));
#50878=CARTESIAN_POINT('Ctrl Pts',(-0.015132689504921,0.0120833333333333,
0.0102218440523409));
#50879=CARTESIAN_POINT('Ctrl Pts',(-0.04,0.00939955463535607,0.00464026426357805));
#50880=CARTESIAN_POINT('Ctrl Pts',(-0.0302431702683995,0.00939955463535607,
0.00464026426357805));
#50881=CARTESIAN_POINT('Ctrl Pts',(-0.0243148560847983,0.010324886351761,
0.00570100281151992));
#50882=CARTESIAN_POINT('Ctrl Pts',(-0.015132689504921,0.0112502172223832,
0.0102218440523409));
#50883=CARTESIAN_POINT('Ctrl Pts',(-0.04,0.00878403081131148,0.00484680862067135));
#50884=CARTESIAN_POINT('Ctrl Pts',(-0.0302697286340305,0.00878403081131148,
0.00484680862067135));
#50885=CARTESIAN_POINT('Ctrl Pts',(-0.0243287164435937,0.00939236853247558,
0.00571836367863856));
#50886=CARTESIAN_POINT('Ctrl Pts',(-0.015132689504921,0.0100007058837482,
0.0102218440523409));
#50887=CARTESIAN_POINT('Ctrl Pts',(-0.04,0.00814718747550223,0.00497205619922113));
#50888=CARTESIAN_POINT('Ctrl Pts',(-0.0302858937355252,0.00814718747550223,
0.00497205619922113));
#50889=CARTESIAN_POINT('Ctrl Pts',(-0.0243371647192728,0.00844902839074704,
0.00572692482666522));
#50890=CARTESIAN_POINT('Ctrl Pts',(-0.015132689504921,0.00875086923557139,
0.0102218440523409));
#50891=CARTESIAN_POINT('Ctrl Pts',(-0.04,0.00771565028284425,0.005));
#50892=CARTESIAN_POINT('Ctrl Pts',(-0.0302893398503779,0.00771565028284425,
0.005));
#50893=CARTESIAN_POINT('Ctrl Pts',(-0.0243389737765017,0.00781637598055064,
0.00572818395833523));
#50894=CARTESIAN_POINT('Ctrl Pts',(-0.015132689504921,0.00791710167825684,
0.0102218440523409));
#50895=CARTESIAN_POINT('Ctrl Pts',(-0.04,0.00728479953731841,0.005));
#50896=CARTESIAN_POINT('Ctrl Pts',(-0.0302893395753294,0.00728479953731841,
0.005));
#50897=CARTESIAN_POINT('Ctrl Pts',(-0.0243389736389774,0.00718428394112105,
0.00572818395833523));
#50898=CARTESIAN_POINT('Ctrl Pts',(-0.015132689504921,0.0070837683449235,
0.0102218440523409));
#50899=CARTESIAN_POINT('Ctrl Pts',(-0.04,0.00685462242848371,0.00497218239515157));
#50900=CARTESIAN_POINT('Ctrl Pts',(-0.0302859072730621,0.00685462242848371,
0.00497218239515157));
#50901=CARTESIAN_POINT('Ctrl Pts',(-0.0243371722033388,0.00655274665477437,
0.00572688218702066));
#50902=CARTESIAN_POINT('Ctrl Pts',(-0.015132689504921,0.00625087081123028,
0.0102218440523409));
#50903=CARTESIAN_POINT('Ctrl Pts',(-0.04,0.00622049631377248,0.00484786604032014));
#50904=CARTESIAN_POINT('Ctrl Pts',(-0.030269763463618,0.00622049631377248,
0.00484786604032014));
#50905=CARTESIAN_POINT('Ctrl Pts',(-0.0243287375276573,0.00561060229378754,
0.00571834998513381));
#50906=CARTESIAN_POINT('Ctrl Pts',(-0.015132689504921,0.00500070790691571,
0.0102218440523409));
#50907=CARTESIAN_POINT('Ctrl Pts',(-0.04,0.00560781375559217,0.00464312151315633));
#50908=CARTESIAN_POINT('Ctrl Pts',(-0.0302432149127319,0.00560781375559217,
0.00464312151315633));
#50909=CARTESIAN_POINT('Ctrl Pts',(-0.0243148866463651,0.0046790161922589,
0.00570121346148063));
#50910=CARTESIAN_POINT('Ctrl Pts',(-0.015132689504921,0.00375021778988959,
0.0102218440523409));
#50911=CARTESIAN_POINT('Ctrl Pts',(-0.04,0.00522022257304718,0.00445520250630582));
#50912=CARTESIAN_POINT('Ctrl Pts',(-0.0302146387773497,0.00522022257304718,
0.00445520250630582));
#50913=CARTESIAN_POINT('Ctrl Pts',(-0.0243000856243898,0.00406844524938924,
0.00568308051796475));
#50914=CARTESIAN_POINT('Ctrl Pts',(-0.015132689504921,0.00291666666666667,
0.0102218440523409));
#50915=CARTESIAN_POINT('Ctrl Pts',(-0.04,0.00503323066735754,0.0043491434857377));
#50916=CARTESIAN_POINT('Ctrl Pts',(-0.0302003506952954,0.00503323066735754,
0.0043491434857377));
#50917=CARTESIAN_POINT('Ctrl Pts',(-0.0242926564701765,0.00376661607994243,
0.00567219736021384));
#50918=CARTESIAN_POINT('Ctrl Pts',(-0.015132689504921,0.0025,0.0102218440523409));
#50919=CARTESIAN_POINT('Ctrl Pts',(-0.04,0.00471683689703473,0.00416968965713194));
#50920=CARTESIAN_POINT('Ctrl Pts',(-0.0301761749956299,0.00471683689703473,
0.00416968965713194));
#50921=CARTESIAN_POINT('Ctrl Pts',(-0.024280086203548,0.00325591553083319,
0.00565378285557991));
#50922=CARTESIAN_POINT('Ctrl Pts',(-0.015132689504921,0.00179499227708115,
0.0102218440523409));
#50923=CARTESIAN_POINT('Ctrl Pts',(-0.04,0.00440044312671191,0.00399023582852618));
#50924=CARTESIAN_POINT('Ctrl Pts',(-0.0301519992959643,0.00440044312671191,
0.00399023582852618));
#50925=CARTESIAN_POINT('Ctrl Pts',(-0.0242675159369196,0.00274521498172396,
0.005635368350946));
#50926=CARTESIAN_POINT('Ctrl Pts',(-0.015132689504921,0.00108998455416231,
0.0102218440523409));
#50927=CARTESIAN_POINT('Ctrl Pts',(-0.04,0.00408404935638909,0.00381078199992041));
#50928=CARTESIAN_POINT('Ctrl Pts',(-0.0301278235962988,0.00408404935638909,
0.00381078199992041));
#50929=CARTESIAN_POINT('Ctrl Pts',(-0.0242549456702911,0.00223451443261473,
0.00561695384631207));
#50930=CARTESIAN_POINT('Ctrl Pts',(-0.015132689504921,0.000384976831243464,
0.0102218440523409));
#50931=CARTESIAN_POINT('',(-0.0151954874261301,0.00138726386665834,0.0101904076586258));
#50932=CARTESIAN_POINT('',(-0.0151988434694278,0.00250046000682414,0.0101890120162147));
#50933=CARTESIAN_POINT('',(-0.0151988171013996,0.00250046001831896,0.0101889589173828));
#50934=CARTESIAN_POINT('',(-0.0152015959590704,0.0114763663518353,0.0101878882534135));
#50935=CARTESIAN_POINT('Ctrl Pts',(-0.0152015961008204,0.0114763663334547,
0.0101878881836326));
#50936=CARTESIAN_POINT('Ctrl Pts',(-0.0152017816534068,0.011398632919723,
0.0101878129849584));
#50937=CARTESIAN_POINT('Ctrl Pts',(-0.0152019618681523,0.0113209171151958,
0.010187739932766));
#50938=CARTESIAN_POINT('Ctrl Pts',(-0.01520213666228,0.0112432182788952,
0.0101876690159898));
#50939=CARTESIAN_POINT('Ctrl Pts',(-0.0152030730346569,0.0108269855086917,
0.0101872891147244));
#50940=CARTESIAN_POINT('Ctrl Pts',(-0.0152038537517294,0.0104112394262679,
0.0101869703999302));
#50941=CARTESIAN_POINT('Ctrl Pts',(-0.0152044807446706,0.0099958840151301,
0.0101867127986388));
#50942=CARTESIAN_POINT('Ctrl Pts',(-0.0152051090343512,0.00957966957078026,
0.0101864546645795));
#50943=CARTESIAN_POINT('Ctrl Pts',(-0.015205583009041,0.00916384747612361,
0.0101862579082725));
#50944=CARTESIAN_POINT('Ctrl Pts',(-0.0152059010693488,0.00874832374241293,
0.0101861245001562));
#50945=CARTESIAN_POINT('Ctrl Pts',(-0.01520621978241,0.00833194723164394,
0.0101859908182471));
#50946=CARTESIAN_POINT('Ctrl Pts',(-0.0152063819377999,0.00791587037027076,
0.0101859207682779));
#50947=CARTESIAN_POINT('Ctrl Pts',(-0.0152063872987604,0.00750000000000001,
0.0101859181580662));
#50948=CARTESIAN_POINT('Ctrl Pts',(-0.0152063926594201,0.00708415296700099,
0.0101859155480011));
#50949=CARTESIAN_POINT('Ctrl Pts',(-0.0152062412439683,0.00666851248133758,
0.0101859801722236));
#50950=CARTESIAN_POINT('Ctrl Pts',(-0.01520593249939,0.00625314726721103,
0.010186109005589));
#50951=CARTESIAN_POINT('Ctrl Pts',(-0.0152056231325436,0.00583694489345328,
0.0101862380986153));
#50952=CARTESIAN_POINT('Ctrl Pts',(-0.0152051558060071,0.00542101895440168,
0.0101864316392808));
#50953=CARTESIAN_POINT('Ctrl Pts',(-0.0152045313571514,0.0050054370581099,
0.0101866883096197));
#50954=CARTESIAN_POINT('Ctrl Pts',(-0.0152039056601427,0.00458902449362444,
0.0101869454929931));
#50955=CARTESIAN_POINT('Ctrl Pts',(-0.0152031221583381,0.0041729573969788,
0.0101872660473249));
#50956=CARTESIAN_POINT('Ctrl Pts',(-0.0152021782357305,0.00375730094918648,
0.0101876505057982));
#50957=CARTESIAN_POINT('Ctrl Pts',(-0.0152012258433854,0.00333791485133816,
0.0101880384139849));
#50958=CARTESIAN_POINT('Ctrl Pts',(-0.0152001103659201,0.00291894870724609,
0.0101884911917733));
#50959=CARTESIAN_POINT('Ctrl Pts',(-0.0151988434694278,0.00250046000682414,
0.0101890120162147));
#50960=CARTESIAN_POINT('',(-0.0312397316217442,0.0094458100603598,0.00513213307870327));
#50961=CARTESIAN_POINT('Ctrl Pts',(-0.0152015959590704,0.0114763663518353,
0.0101878882534135));
#50962=CARTESIAN_POINT('Ctrl Pts',(-0.0164822330050404,0.0115970872170385,
0.00955739480663315));
#50963=CARTESIAN_POINT('Ctrl Pts',(-0.0190840779032895,0.0117290721415925,
0.00834467796691021));
#50964=CARTESIAN_POINT('Ctrl Pts',(-0.0223800331608592,0.0115286687609144,
0.00700184797404235));
#50965=CARTESIAN_POINT('Ctrl Pts',(-0.024989720469363,0.0104626073224454,
0.00625685260897244));
#50966=CARTESIAN_POINT('Ctrl Pts',(-0.0269857198322412,0.0097622199194132,
0.00582377715676942));
#50967=CARTESIAN_POINT('Ctrl Pts',(-0.0290810941162661,0.00943689998545597,
0.00544737164840719));
#50968=CARTESIAN_POINT('Ctrl Pts',(-0.0305231562376279,0.00939584156846951,
0.00523939408016512));
#50969=CARTESIAN_POINT('Ctrl Pts',(-0.0312397316217442,0.0094458100603598,
0.00513213307870327));
#50970=CARTESIAN_POINT('Ctrl Pts',(-0.0399999963113939,0.00997613772986841,
0.00434381651807744));
#50971=CARTESIAN_POINT('Ctrl Pts',(-0.0395727207349401,0.00997285044000123,
0.00434569041850028));
#50972=CARTESIAN_POINT('Ctrl Pts',(-0.0391774221470677,0.00996743224495432,
0.00435266025984037));
#50973=CARTESIAN_POINT('Ctrl Pts',(-0.0388081300295977,0.00995937345471727,
0.00436370338220723));
#50974=CARTESIAN_POINT('Ctrl Pts',(-0.038623483760588,0.00995534405501007,
0.0043692249496786));
#50975=CARTESIAN_POINT('Ctrl Pts',(-0.0384453396441767,0.00995066250224038,
0.00437577831952124));
#50976=CARTESIAN_POINT('Ctrl Pts',(-0.0382796892328055,0.0099455119793533,
0.00438289030257414));
#50977=CARTESIAN_POINT('Ctrl Pts',(-0.0381140388214343,0.00994036145646621,
0.00439000228562705));
#50978=CARTESIAN_POINT('Ctrl Pts',(-0.0379608807865865,0.00993471250155751,
0.00439761931275741));
#50979=CARTESIAN_POINT('Ctrl Pts',(-0.0377962431644136,0.00992758518542438,
0.00440693404825424));
#50980=CARTESIAN_POINT('Ctrl Pts',(-0.0376316055422407,0.00992045786929125,
0.00441624878375107));
#50981=CARTESIAN_POINT('Ctrl Pts',(-0.0374554905385062,0.00991188455435292,
0.00442732222488304));
#50982=CARTESIAN_POINT('Ctrl Pts',(-0.0372779553803839,0.00990245493066738,
0.00443955772907257));
#50983=CARTESIAN_POINT('Ctrl Pts',(-0.0371004202222617,0.00989302530698183,
0.0044517932332621));
#50984=CARTESIAN_POINT('Ctrl Pts',(-0.0369214637592435,0.00988272837523341,
0.00446516860036496));
#50985=CARTESIAN_POINT('Ctrl Pts',(-0.0367394606492448,0.00987155476925158,
0.00447975421625176));
#50986=CARTESIAN_POINT('Ctrl Pts',(-0.0365574575392462,0.00986038116326974,
0.00449433983213856));
#50987=CARTESIAN_POINT('Ctrl Pts',(-0.0363724078513935,0.00984832902852278,
0.00451013306105462));
#50988=CARTESIAN_POINT('Ctrl Pts',(-0.0361807646956626,0.00983512789932526,
0.00452749358356716));
#50989=CARTESIAN_POINT('Ctrl Pts',(-0.0360849431177971,0.0098285273347265,
0.00453617384482344));
#50990=CARTESIAN_POINT('Ctrl Pts',(-0.0359874734742924,0.00982164264879878,
0.00454525213533095));
#50991=CARTESIAN_POINT('Ctrl Pts',(-0.035893843336345,0.00981489791188518,
0.00455418267100008));
#50992=CARTESIAN_POINT('Ctrl Pts',(-0.0358470282673713,0.00981152554342839,
0.00455864793883465));
#50993=CARTESIAN_POINT('Ctrl Pts',(-0.0358011728108698,0.00980818594822577,
0.00456307163081677));
#50994=CARTESIAN_POINT('Ctrl Pts',(-0.0357484897779608,0.00980428569995241,
0.00456823103120321));
#50995=CARTESIAN_POINT('Ctrl Pts',(-0.0356958067450518,0.00980038545167904,
0.00457339043158964));
#50996=CARTESIAN_POINT('Ctrl Pts',(-0.0356362972078298,0.0097959327453508,
0.00457930316019586));
#50997=CARTESIAN_POINT('Ctrl Pts',(-0.0356018745250502,0.00979334381551296,
0.00458274850248771));
#50998=CARTESIAN_POINT('Ctrl Pts',(-0.0355674518422706,0.00979075488567512,
0.00458619384477956));
#50999=CARTESIAN_POINT('Ctrl Pts',(-0.035558114721345,0.00979002055266094,
0.004587151616026));
#51000=CARTESIAN_POINT('Ctrl Pts',(-0.0355408565612769,0.00978866582053624,
0.00458891568512121));
#51001=CARTESIAN_POINT('Ctrl Pts',(-0.0355235984012088,0.00978731108841154,
0.00459067975421642));
#51002=CARTESIAN_POINT('Ctrl Pts',(-0.0354984196904949,0.00978533935191339,
0.00459325763773581));
#51003=CARTESIAN_POINT('Ctrl Pts',(-0.0354733783364266,0.00978335509992397,
0.00459584349182381));
#51004=CARTESIAN_POINT('Ctrl Pts',(-0.0354232956282899,0.00977938659594515,
0.00460101519999981));
#51005=CARTESIAN_POINT('Ctrl Pts',(-0.035373761755283,0.00977536405827277,
0.00460620989793128));
#51006=CARTESIAN_POINT('Ctrl Pts',(-0.0353190429282953,0.00977087262090177,
0.00461201651237702));
#51007=CARTESIAN_POINT('Ctrl Pts',(-0.0352096052743198,0.00976188974615977,
0.00462362974126851));
#51008=CARTESIAN_POINT('Ctrl Pts',(-0.0350794285821523,0.0097510360376019,
0.00463770164690174));
#51009=CARTESIAN_POINT('Ctrl Pts',(-0.0349328736445292,0.00973875823053989,
0.00465393589977913));
#51010=CARTESIAN_POINT('Ctrl Pts',(-0.0347863187069061,0.00972648042347788,
0.00467017015265652));
#51011=CARTESIAN_POINT('Ctrl Pts',(-0.0346233849589686,0.00971277610529657,
0.00468856026966512));
#51012=CARTESIAN_POINT('Ctrl Pts',(-0.0344434237965824,0.00969774093599419,
0.00470937315437457));
#51013=CARTESIAN_POINT('Ctrl Pts',(-0.0342634626341962,0.00968270576669181,
0.00473018603908403));
#51014=CARTESIAN_POINT('Ctrl Pts',(-0.0340664737728119,0.00966633834195001,
0.00475341814438052));
#51015=CARTESIAN_POINT('Ctrl Pts',(-0.0338507957444424,0.00964862558079126,
0.00477957655683347));
#51016=CARTESIAN_POINT('Ctrl Pts',(-0.033635117716073,0.00963091281963251,
0.00480573496928642));
#51017=CARTESIAN_POINT('Ctrl Pts',(-0.0334007516791016,0.00961186312715902,
0.00483483833198576));
#51018=CARTESIAN_POINT('Ctrl Pts',(-0.0331551679662072,0.00959217322514504,
0.00486632682771846));
#51019=CARTESIAN_POINT('Ctrl Pts',(-0.0330760295422204,0.00958582822858368,
0.00487647387654605));
#51020=CARTESIAN_POINT('Ctrl Pts',(-0.0329957316495097,0.00957941374634901,
0.00488686539521972));
#51021=CARTESIAN_POINT('Ctrl Pts',(-0.0329117016047792,0.00957272879821522,
0.00489785656965405));
#51022=CARTESIAN_POINT('Ctrl Pts',(-0.0328653499124219,0.0095690413235707,
0.00490391939560707));
#51023=CARTESIAN_POINT('Ctrl Pts',(-0.0328178634923766,0.00956527148213439,
0.00491016513951892));
#51024=CARTESIAN_POINT('Ctrl Pts',(-0.0327688172992972,0.00956138477500662,
0.0049166573228122));
#51025=CARTESIAN_POINT('Ctrl Pts',(-0.0326308562556758,0.00955045193520946,
0.00493491905377004));
#51026=CARTESIAN_POINT('Ctrl Pts',(-0.0324805400366365,0.00953861874307939,
0.00495519116579573));
#51027=CARTESIAN_POINT('Ctrl Pts',(-0.0323568441831232,0.00952894684544298,
0.00497213739513634));
#51028=CARTESIAN_POINT('Ctrl Pts',(-0.0322331483296099,0.00951927494780657,
0.00498908362447695));
#51029=CARTESIAN_POINT('Ctrl Pts',(-0.0321360619477995,0.00951173925946108,
0.00500261247870721));
#51030=CARTESIAN_POINT('Ctrl Pts',(-0.0320408372393364,0.00950445735094549,
0.00501598963619049));
#51031=CARTESIAN_POINT('Ctrl Pts',(-0.0319456125308732,0.00949717544242991,
0.00502936679367378));
#51032=CARTESIAN_POINT('Ctrl Pts',(-0.0318522535426534,0.00949015539818618,
0.00504262417088863));
#51033=CARTESIAN_POINT('Ctrl Pts',(-0.0317610696020343,0.00948339134457126,
0.00505571215967831));
#51034=CARTESIAN_POINT('Ctrl Pts',(-0.031578701720796,0.00946986323734143,
0.00508188813725767));
#51035=CARTESIAN_POINT('Ctrl Pts',(-0.0314050335764244,0.00945735900266527,
0.00510738446670119));
#51036=CARTESIAN_POINT('Ctrl Pts',(-0.0312397480889472,0.00944581580409354,
0.00513212950872993));
#51037=CARTESIAN_POINT('',(-0.0328230358245329,0.00544566815053618,0.00491342083293496));
#51038=CARTESIAN_POINT('Ctrl Pts',(-0.0328230369063753,0.00544566823007687,
0.004913420741839));
#51039=CARTESIAN_POINT('Ctrl Pts',(-0.0328639380316224,0.00544232996851928,
0.00490802387191221));
#51040=CARTESIAN_POINT('Ctrl Pts',(-0.0329048023388109,0.00543898823253315,
0.0049026586055584));
#51041=CARTESIAN_POINT('Ctrl Pts',(-0.0329456376870304,0.00543564306204493,
0.00489732356927106));
#51042=CARTESIAN_POINT('Ctrl Pts',(-0.0334983654612919,0.00539036443166469,
0.0048251110656123));
#51043=CARTESIAN_POINT('Ctrl Pts',(-0.0340455908507357,0.00534450047275511,
0.00475826196747422));
#51044=CARTESIAN_POINT('Ctrl Pts',(-0.0346080623193213,0.00529790266814098,
0.00469454242292275));
#51045=CARTESIAN_POINT('Ctrl Pts',(-0.0352120889970945,0.00524786223287521,
0.00462611529914093));
#51046=CARTESIAN_POINT('Ctrl Pts',(-0.0358336884751567,0.00519690059485905,
0.0045615118622913));
#51047=CARTESIAN_POINT('Ctrl Pts',(-0.0364254518271606,0.00515762208071706,
0.00451052778445893));
#51048=CARTESIAN_POINT('Ctrl Pts',(-0.0367213335031625,0.00513798282364607,
0.00448503574554275));
#51049=CARTESIAN_POINT('Ctrl Pts',(-0.0370097554634641,0.00512128557881895,
0.00446291352900774));
#51050=CARTESIAN_POINT('Ctrl Pts',(-0.0373032936896531,0.00510605563371512,
0.00444304865414545));
#51051=CARTESIAN_POINT('Ctrl Pts',(-0.037596831915842,0.00509082568861129,
0.00442318377928316));
#51052=CARTESIAN_POINT('Ctrl Pts',(-0.0378954859573303,0.00507705411343856,
0.00440558951191052));
#51053=CARTESIAN_POINT('Ctrl Pts',(-0.0382016060804483,0.00506597225077648,
0.00439128773751753));
#51054=CARTESIAN_POINT('Ctrl Pts',(-0.0383546661420073,0.00506043131944544,
0.00438413685032104));
#51055=CARTESIAN_POINT('Ctrl Pts',(-0.0385095939076617,0.00505554447971043,
0.00437784345578198));
#51056=CARTESIAN_POINT('Ctrl Pts',(-0.0386482553555084,0.00505173469434079,
0.00437294110524465));
#51057=CARTESIAN_POINT('Ctrl Pts',(-0.0387869168033552,0.00504792490897116,
0.00436803875470732));
#51058=CARTESIAN_POINT('Ctrl Pts',(-0.0389093103817168,0.00504523305797351,
0.00436445359723158));
#51059=CARTESIAN_POINT('Ctrl Pts',(-0.0390446531092923,0.00504293774392477,
0.00436126274908846));
#51060=CARTESIAN_POINT('Ctrl Pts',(-0.0393153385644433,0.00503834711582729,
0.00435488105280222));
#51061=CARTESIAN_POINT('Ctrl Pts',(-0.0396378214009135,0.00503522981875482,
0.00435027737761781));
#51062=CARTESIAN_POINT('Ctrl Pts',(-0.0399999989166321,0.00503323485180867,
0.00434914585909333));
#51063=CARTESIAN_POINT('',(-0.0264682077184971,0.00413293976380557,0.00578983210446623));
#51064=CARTESIAN_POINT('Ctrl Pts',(-0.0328230352836106,0.00544566811076599,
0.00491342087848311));
#51065=CARTESIAN_POINT('Ctrl Pts',(-0.0317248902824274,0.00553525857937583,
0.00505830862461719));
#51066=CARTESIAN_POINT('Ctrl Pts',(-0.0306169938636662,0.00546790864877236,
0.00518271767823649));
#51067=CARTESIAN_POINT('Ctrl Pts',(-0.0295432381737695,0.00525773711428087,
0.00532646011294394));
#51068=CARTESIAN_POINT('Ctrl Pts',(-0.0294386032779061,0.00523725640639555,
0.00534046746566699));
#51069=CARTESIAN_POINT('Ctrl Pts',(-0.0293344280137762,0.00521502239184281,
0.00535450046456667));
#51070=CARTESIAN_POINT('Ctrl Pts',(-0.029230698113076,0.00519108565783119,
0.00536858848140193));
#51071=CARTESIAN_POINT('Ctrl Pts',(-0.0288021936660945,0.0050922038802439,
0.00542678556654621));
#51072=CARTESIAN_POINT('Ctrl Pts',(-0.0283812536935357,0.00496418264609604,
0.00548594698764365));
#51073=CARTESIAN_POINT('Ctrl Pts',(-0.0279671299999509,0.00481124380670639,
0.00554783288921987));
#51074=CARTESIAN_POINT('Ctrl Pts',(-0.0274527576160298,0.00462128240959336,
0.005624699775172));
#51075=CARTESIAN_POINT('Ctrl Pts',(-0.0269519544474792,0.0043856239194066,
0.00570367476051854));
#51076=CARTESIAN_POINT('Ctrl Pts',(-0.0264682077184971,0.00413293976380557,
0.00578983210446623));
#51077=CARTESIAN_POINT('Ctrl Pts',(-0.0264682077184971,0.00413293976380557,
0.00578983210446622));
#51078=CARTESIAN_POINT('Ctrl Pts',(-0.0255345075599796,0.00370448613396262,
0.00596797782102129));
#51079=CARTESIAN_POINT('Ctrl Pts',(-0.0242258662820284,0.00284076935409089,
0.00627087795151936));
#51080=CARTESIAN_POINT('Ctrl Pts',(-0.022409245668868,0.00204459924778921,
0.00690371256898279));
#51081=CARTESIAN_POINT('Ctrl Pts',(-0.0204776433343773,0.00155987639176132,
0.00768508726377031));
#51082=CARTESIAN_POINT('Ctrl Pts',(-0.0180574935154255,0.00137301442411395,
0.00878450427407825));
#51083=CARTESIAN_POINT('Ctrl Pts',(-0.0161475216239444,0.00137134461148134,
0.00971405996459154));
#51084=CARTESIAN_POINT('Ctrl Pts',(-0.0151954862452661,0.00138726386753766,
0.0101904052898562));
#51085=CARTESIAN_POINT('Ctrl Pts',(-0.04,0.00749999999999979,-0.005));
#51086=CARTESIAN_POINT('Ctrl Pts',(-0.0303290418474347,0.0075,-0.005));
#51087=CARTESIAN_POINT('Ctrl Pts',(-0.0243876928299813,0.0075,-0.00572224175535161));
#51088=CARTESIAN_POINT('Ctrl Pts',(-0.0152410184731965,0.00749997928621807,
-0.0101578071909577));
#51089=CARTESIAN_POINT('Ctrl Pts',(-0.04,0.00771571946746142,-0.005));
#51090=CARTESIAN_POINT('Ctrl Pts',(-0.030332352871244,0.00771570651417863,
-0.005));
#51091=CARTESIAN_POINT('Ctrl Pts',(-0.0243938667366865,0.00781640214171287,
-0.00571957082345507));
#51092=CARTESIAN_POINT('Ctrl Pts',(-0.015250055386927,0.00791708269062151,
-0.0101524651702489));
#51093=CARTESIAN_POINT('Ctrl Pts',(-0.04,0.00814739511140643,-0.0049720382424295));
#51094=CARTESIAN_POINT('Ctrl Pts',(-0.0303359967783258,0.00814739511140643,
-0.0049720382424295));
#51095=CARTESIAN_POINT('Ctrl Pts',(-0.0244048070000265,0.00844913472747877,
-0.00571297156313869));
#51096=CARTESIAN_POINT('Ctrl Pts',(-0.0152681197724132,0.00875085370023442,
-0.010141786710297));
#51097=CARTESIAN_POINT('Ctrl Pts',(-0.04,0.00878443578896302,-0.00484671062820502));
#51098=CARTESIAN_POINT('Ctrl Pts',(-0.0303292164550866,0.00878443578896302,
-0.00484671062820502));
#51099=CARTESIAN_POINT('Ctrl Pts',(-0.0244153222548556,0.00939257582974028,
-0.00569640045348333));
#51100=CARTESIAN_POINT('Ctrl Pts',(-0.0152951986997117,0.0100006955268584,
-0.0101257794544224));
#51101=CARTESIAN_POINT('Ctrl Pts',(-0.04,0.00940013645719661,-0.00464003578100023));
#51102=CARTESIAN_POINT('Ctrl Pts',(-0.0303128163764084,0.00940013645719661,
-0.00464003578100023));
#51103=CARTESIAN_POINT('Ctrl Pts',(-0.024421239683557,0.0103251841843068,
-0.00567102489989924));
#51104=CARTESIAN_POINT('Ctrl Pts',(-0.0153222705788916,0.0112502120439379,
-0.0101097763649254));
#51105=CARTESIAN_POINT('Ctrl Pts',(-0.04,0.00978928948362159,-0.0044503691604976));
#51106=CARTESIAN_POINT('Ctrl Pts',(-0.030290878085034,0.00978928948362159,
-0.0044503691604976));
#51107=CARTESIAN_POINT('Ctrl Pts',(-0.0244198128798258,0.0109363202673876,
-0.00564731163699517));
#51108=CARTESIAN_POINT('Ctrl Pts',(-0.0153403208502169,0.0120833316071848,
-0.0100991062483243));
#51109=CARTESIAN_POINT('Ctrl Pts',(-0.04,0.00997687591821936,-0.00434339564002003));
#51110=CARTESIAN_POINT('Ctrl Pts',(-0.0302799089538077,0.00997687591821936,
-0.00434339564002003));
#51111=CARTESIAN_POINT('Ctrl Pts',(-0.0244191294928241,0.0112384475634125,
-0.00563364610458802));
#51112=CARTESIAN_POINT('Ctrl Pts',(-0.0153493483390368,0.0125,-0.010093769798994));
#51113=CARTESIAN_POINT('Ctrl Pts',(-0.04,0.00998137799264972,-0.00434082827552856));
#51114=CARTESIAN_POINT('Ctrl Pts',(-0.0302796456946583,0.00998137799264972,
-0.00434082827552856));
#51115=CARTESIAN_POINT('Ctrl Pts',(-0.024419113091536,0.0112456986185171,
-0.00563331813181025));
#51116=CARTESIAN_POINT('Ctrl Pts',(-0.0153495649987685,0.0125100000414276,
-0.01009364172421));
#51117=CARTESIAN_POINT('Ctrl Pts',(-0.04,0.00998588006708007,-0.00433826091103709));
#51118=CARTESIAN_POINT('Ctrl Pts',(-0.0302793824355088,0.00998588006708007,
-0.00433826091103709));
#51119=CARTESIAN_POINT('Ctrl Pts',(-0.024419096690248,0.0112529496736217,
-0.00563299015903248));
#51120=CARTESIAN_POINT('Ctrl Pts',(-0.0153497816585002,0.0125200000828552,
-0.0100935136494261));
#51121=CARTESIAN_POINT('Ctrl Pts',(-0.04,0.00999038214151043,-0.00433569354654562));
#51122=CARTESIAN_POINT('Ctrl Pts',(-0.0302791191763594,0.00999038214151043,
-0.00433569354654562));
#51123=CARTESIAN_POINT('Ctrl Pts',(-0.0244190802889599,0.0112602007287263,
-0.0056326621862547));
#51124=CARTESIAN_POINT('Ctrl Pts',(-0.0153499983182319,0.0125300001242828,
-0.0100933855746422));
#51125=CARTESIAN_POINT('',(-0.0312862171088903,0.00944638115495657,-0.00512344456391754));
#51126=CARTESIAN_POINT('',(-0.0153993022433853,0.0114667765373308,-0.0100716954734317));
#51127=CARTESIAN_POINT('Ctrl Pts',(-0.0312862115324821,0.00944637453608856,
-0.00512344689700562));
#51128=CARTESIAN_POINT('Ctrl Pts',(-0.0309637776590882,0.00942387733413622,
-0.0051712822208625));
#51129=CARTESIAN_POINT('Ctrl Pts',(-0.0306252671936168,0.00941459983377785,
-0.00522057750595682));
#51130=CARTESIAN_POINT('Ctrl Pts',(-0.0302766727676078,0.0094192040795314,
-0.00527223065634118));
#51131=CARTESIAN_POINT('Ctrl Pts',(-0.0301023755546034,0.00942150620240818,
-0.00529805723153336));
#51132=CARTESIAN_POINT('Ctrl Pts',(-0.0299255532958684,0.00942727365630772,
-0.00532444668236705));
#51133=CARTESIAN_POINT('Ctrl Pts',(-0.0297403618928456,0.00943736002554799,
-0.00535253435011197));
#51134=CARTESIAN_POINT('Ctrl Pts',(-0.029556761151514,0.0094473597600909,
-0.00538038076488105));
#51135=CARTESIAN_POINT('Ctrl Pts',(-0.0293649521540202,0.00946162638074927,
-0.00541002676602812));
#51136=CARTESIAN_POINT('Ctrl Pts',(-0.0291876741818143,0.00947800447060625,
-0.00543813008769592));
#51137=CARTESIAN_POINT('Ctrl Pts',(-0.0291861382986962,0.00947814636545876,
-0.00543837356643599));
#51138=CARTESIAN_POINT('Ctrl Pts',(-0.0291846035006668,0.0094782883980757,
-0.00543861692592945));
#51139=CARTESIAN_POINT('Ctrl Pts',(-0.0291830698022148,0.0094784305660575,
-0.00543886016370823));
#51140=CARTESIAN_POINT('Ctrl Pts',(-0.0290045102947476,0.00949498234960806,
-0.00546717891040807));
#51141=CARTESIAN_POINT('Ctrl Pts',(-0.0288408630926145,0.00951330253321414,
-0.00549375476339945));
#51142=CARTESIAN_POINT('Ctrl Pts',(-0.0286701482711043,0.00953506074917197,
-0.00552219615883888));
#51143=CARTESIAN_POINT('Ctrl Pts',(-0.028508184501729,0.00955570361216557,
-0.00554917961329769));
#51144=CARTESIAN_POINT('Ctrl Pts',(-0.0283399114830045,0.00957969213306091,
-0.00557789203041364));
#51145=CARTESIAN_POINT('Ctrl Pts',(-0.0281683704016501,0.00960696702812576,
-0.00560802085849635));
#51146=CARTESIAN_POINT('Ctrl Pts',(-0.0281591018784983,0.00960844071591165,
-0.0056096487469206));
#51147=CARTESIAN_POINT('Ctrl Pts',(-0.0281498237908751,0.00960992389677818,
-0.00561128075793803));
#51148=CARTESIAN_POINT('Ctrl Pts',(-0.0281405366360636,0.00961141669311603,
-0.00561291680941586));
#51149=CARTESIAN_POINT('Ctrl Pts',(-0.0279593635666388,0.00964053804406211,
-0.00564483277011575));
#51150=CARTESIAN_POINT('Ctrl Pts',(-0.0277747902540233,0.00967354473406514,
-0.00567833500513236));
#51151=CARTESIAN_POINT('Ctrl Pts',(-0.0276041796877202,0.0097071526084523,
-0.0057101570143216));
#51152=CARTESIAN_POINT('Ctrl Pts',(-0.0274515130799449,0.00973722577618398,
-0.00573863214514608));
#51153=CARTESIAN_POINT('Ctrl Pts',(-0.0273100027030909,0.0097677872656343,
-0.00576563349689761));
#51154=CARTESIAN_POINT('Ctrl Pts',(-0.0271674409538542,0.00980147476959505,
-0.00579334150457946));
#51155=CARTESIAN_POINT('Ctrl Pts',(-0.0271506846889891,0.00980543429409607,
-0.00579659821767458));
#51156=CARTESIAN_POINT('Ctrl Pts',(-0.0271339143954177,0.00980943896688865,
-0.00579986504241665));
#51157=CARTESIAN_POINT('Ctrl Pts',(-0.0271171104745114,0.00981349342444696,
-0.00580314598638567));
#51158=CARTESIAN_POINT('Ctrl Pts',(-0.0269573393483396,0.00985204307328881,
-0.00583434109351309));
#51159=CARTESIAN_POINT('Ctrl Pts',(-0.0267945505097115,0.00989516287810736,
-0.00586677365462162));
#51160=CARTESIAN_POINT('Ctrl Pts',(-0.0266247015642492,0.00994409565256879,
-0.00590153635079375));
#51161=CARTESIAN_POINT('Ctrl Pts',(-0.0264784296662473,0.00998623597775886,
-0.00593147357256995));
#51162=CARTESIAN_POINT('Ctrl Pts',(-0.02632699118218,0.0100328896891732,
-0.00596318698623446));
#51163=CARTESIAN_POINT('Ctrl Pts',(-0.0261854108087996,0.0100788793244123,
-0.005993548729033));
#51164=CARTESIAN_POINT('Ctrl Pts',(-0.0260760741453728,0.0101143952165463,
-0.0060169958465547));
#51165=CARTESIAN_POINT('Ctrl Pts',(-0.0259768435751314,0.0101478543253226,
-0.00603864076498111));
#51166=CARTESIAN_POINT('Ctrl Pts',(-0.0258650339339585,0.0101868563097126,
-0.00606350292810076));
#51167=CARTESIAN_POINT('Ctrl Pts',(-0.0257714448770845,0.0102195025010159,
-0.00608431353417914));
#51168=CARTESIAN_POINT('Ctrl Pts',(-0.0256712562003281,0.0102555305630453,
-0.00610698811533278));
#51169=CARTESIAN_POINT('Ctrl Pts',(-0.0255880677504924,0.0102861067539666,
-0.00612610003138942));
#51170=CARTESIAN_POINT('Ctrl Pts',(-0.025525742218938,0.0103090147100091,
-0.0061404188500428));
#51171=CARTESIAN_POINT('Ctrl Pts',(-0.0254695370675074,0.0103300005111268,
-0.00615347166176308));
#51172=CARTESIAN_POINT('Ctrl Pts',(-0.0254073476614081,0.0103535531862672,
-0.00616807571128237));
#51173=CARTESIAN_POINT('Ctrl Pts',(-0.0253535877382479,0.0103739134065231,
-0.00618070025023894));
#51174=CARTESIAN_POINT('Ctrl Pts',(-0.02529536568145,0.0103962193642769,
-0.0061944786610525));
#51175=CARTESIAN_POINT('Ctrl Pts',(-0.0252255351681319,0.0104234572923136,
-0.00621124134451748));
#51176=CARTESIAN_POINT('Ctrl Pts',(-0.0251985237534633,0.0104339933020599,
-0.00621772538383666));
#51177=CARTESIAN_POINT('Ctrl Pts',(-0.0251697766855383,0.0104452709085224,
-0.00622465763411363));
#51178=CARTESIAN_POINT('Ctrl Pts',(-0.0251388823553466,0.0104574636526724,
-0.00623215469285687));
#51179=CARTESIAN_POINT('Ctrl Pts',(-0.0250835008335655,0.0104793205021827,
-0.00624559400419674));
#51180=CARTESIAN_POINT('Ctrl Pts',(-0.0250212132534462,0.010504071707771,
-0.00626089235119378));
#51181=CARTESIAN_POINT('Ctrl Pts',(-0.0249682462297451,0.0105251887155644,
-0.00627405373492803));
#51182=CARTESIAN_POINT('Ctrl Pts',(-0.0249152792060441,0.0105463057233577,
-0.00628721511866228));
#51183=CARTESIAN_POINT('Ctrl Pts',(-0.0248716198962152,0.010563783125094,
-0.0062981968652453));
#51184=CARTESIAN_POINT('Ctrl Pts',(-0.0248308177276274,0.0105801367421535,
-0.006308532384367));
#51185=CARTESIAN_POINT('Ctrl Pts',(-0.0247900155590396,0.0105964903592131,
-0.00631886790348869));
#51186=CARTESIAN_POINT('Ctrl Pts',(-0.0247520767790388,0.010611722753729,
-0.00632857766546725));
#51187=CARTESIAN_POINT('Ctrl Pts',(-0.0247266465107074,0.0106219494716524,
-0.00633511323708019));
#51188=CARTESIAN_POINT('Ctrl Pts',(-0.0247012162423761,0.0106321761895758,
-0.00634164880869312));
#51189=CARTESIAN_POINT('Ctrl Pts',(-0.0246882845826022,0.0106373932110363,
-0.00634497791720677));
#51190=CARTESIAN_POINT('Ctrl Pts',(-0.0246557765988998,0.0106503533471222,
-0.00635343174145392));
#51191=CARTESIAN_POINT('Ctrl Pts',(-0.0246232686151974,0.010663313483208,
-0.00636188556570107));
#51192=CARTESIAN_POINT('Ctrl Pts',(-0.0245712030177206,0.0106840242428176,
-0.0063755247135945));
#51193=CARTESIAN_POINT('Ctrl Pts',(-0.0245254529294777,0.0107021203012,
-0.00638766004577755));
#51194=CARTESIAN_POINT('Ctrl Pts',(-0.0244797028412348,0.0107202163595824,
-0.0063997953779606));
#51195=CARTESIAN_POINT('Ctrl Pts',(-0.0244402539648504,0.0107356922099638,
-0.00641038150709176));
#51196=CARTESIAN_POINT('Ctrl Pts',(-0.024401787931292,0.0107507207636909,
-0.00642078275342784));
#51197=CARTESIAN_POINT('Ctrl Pts',(-0.0243591309274041,0.0107673867158431,
-0.00643231724150351));
#51198=CARTESIAN_POINT('Ctrl Pts',(-0.0243176756195971,0.010783475382793,
-0.00644363819738632));
#51199=CARTESIAN_POINT('Ctrl Pts',(-0.0242760142822199,0.0107994740995014,
-0.00645512973178214));
#51200=CARTESIAN_POINT('Ctrl Pts',(-0.0242425392407811,0.0108123291286123,
-0.00646436322293515));
#51201=CARTESIAN_POINT('Ctrl Pts',(-0.0242089312259155,0.0108251258562557,
-0.00647370735869068));
#51202=CARTESIAN_POINT('Ctrl Pts',(-0.024174459610266,0.010838108471594,
-0.00648337374583902));
#51203=CARTESIAN_POINT('Ctrl Pts',(-0.0240197131328595,0.0108963887103726,
-0.00652676710969123));
#51204=CARTESIAN_POINT('Ctrl Pts',(-0.0238475900116139,0.0109583780048465,
-0.00657681974123949));
#51205=CARTESIAN_POINT('Ctrl Pts',(-0.0236840952009517,0.0110132374264567,
-0.00662623310201612));
#51206=CARTESIAN_POINT('Ctrl Pts',(-0.023559442320716,0.0110550637381547,
-0.00666390718915064));
#51207=CARTESIAN_POINT('Ctrl Pts',(-0.02343984587656,0.0110929839294159,
-0.00670106327199141));
#51208=CARTESIAN_POINT('Ctrl Pts',(-0.0233211950613739,0.0111283428589419,
-0.00673881179428615));
#51209=CARTESIAN_POINT('Ctrl Pts',(-0.0232842233788922,0.0111393607277469,
-0.00675057426197967));
#51210=CARTESIAN_POINT('Ctrl Pts',(-0.0232473428984237,0.0111501264223963,
-0.00676239639079376));
#51211=CARTESIAN_POINT('Ctrl Pts',(-0.0232104306701419,0.011160684460551,
-0.00677431468288953));
#51212=CARTESIAN_POINT('Ctrl Pts',(-0.0230550584291699,0.0112051257236427,
-0.0068244815743961));
#51213=CARTESIAN_POINT('Ctrl Pts',(-0.0228991648663235,0.011246033504623,
-0.00687629484282091));
#51214=CARTESIAN_POINT('Ctrl Pts',(-0.0227355114221791,0.0112845271283102,
-0.00693227480508791));
#51215=CARTESIAN_POINT('Ctrl Pts',(-0.0225718579780346,0.0113230207519974,
-0.0069882547673549));
#51216=CARTESIAN_POINT('Ctrl Pts',(-0.0224004800995218,0.0113591090087216,
-0.00704849884169404));
#51217=CARTESIAN_POINT('Ctrl Pts',(-0.0222392771988294,0.0113895631001835,
-0.00710647929768051));
#51218=CARTESIAN_POINT('Ctrl Pts',(-0.0220780742981369,0.0114200171916454,
-0.00716445975366698));
#51219=CARTESIAN_POINT('Ctrl Pts',(-0.0219269954221904,0.0114448262895038,
-0.00722004153282126));
#51220=CARTESIAN_POINT('Ctrl Pts',(-0.0217673568540159,0.0114682300935694,
-0.00727984153866872));
#51221=CARTESIAN_POINT('Ctrl Pts',(-0.0216875375699287,0.0114799319956022,
-0.00730974154159246));
#51222=CARTESIAN_POINT('Ctrl Pts',(-0.021605583025283,0.0114912832570369,
-0.00734070775038529));
#51223=CARTESIAN_POINT('Ctrl Pts',(-0.0215184026942123,0.0115023523934568,
-0.00737397795079087));
#51224=CARTESIAN_POINT('Ctrl Pts',(-0.0214655245275965,0.0115090662431603,
-0.00739415758510492));
#51225=CARTESIAN_POINT('Ctrl Pts',(-0.0214107408238448,0.0115157425792275,
-0.00741518063249471));
#51226=CARTESIAN_POINT('Ctrl Pts',(-0.0213583486924787,0.0115218521168936,
-0.00743539184785046));
#51227=CARTESIAN_POINT('Ctrl Pts',(-0.0213243618199888,0.0115258153852741,
-0.00744850290062213));
#51228=CARTESIAN_POINT('Ctrl Pts',(-0.021291382533558,0.0115295445612725,
-0.00746127024107871));
#51229=CARTESIAN_POINT('Ctrl Pts',(-0.0212605955531625,0.0115329354582865,
-0.00747322299350472));
#51230=CARTESIAN_POINT('Ctrl Pts',(-0.0211639702187287,0.0115435778322313,
-0.00751073686091653));
#51231=CARTESIAN_POINT('Ctrl Pts',(-0.0210875286442459,0.0115512268304107,
-0.00754069354848727));
#51232=CARTESIAN_POINT('Ctrl Pts',(-0.0209983247349625,0.0115594801200226,
-0.00757590331316513));
#51233=CARTESIAN_POINT('Ctrl Pts',(-0.0208728650989734,0.0115710878479657,
-0.00762542361216579));
#51234=CARTESIAN_POINT('Ctrl Pts',(-0.0207377907557496,0.0115819903082155,
-0.00767933231628551));
#51235=CARTESIAN_POINT('Ctrl Pts',(-0.0206016312582355,0.0115913192905921,
-0.00773432223435744));
#51236=CARTESIAN_POINT('Ctrl Pts',(-0.0204234451009791,0.0116035277340071,
-0.00780628520695928));
#51237=CARTESIAN_POINT('Ctrl Pts',(-0.0202354512665399,0.0116136756292872,
-0.00788327400777926));
#51238=CARTESIAN_POINT('Ctrl Pts',(-0.0200394933157728,0.0116214249104022,
-0.00796472599078757));
#51239=CARTESIAN_POINT('Ctrl Pts',(-0.0199107219649714,0.0116265172549231,
-0.00801825115695901));
#51240=CARTESIAN_POINT('Ctrl Pts',(-0.0197826695329107,0.0116304803730488,
-0.00807194545716316));
#51241=CARTESIAN_POINT('Ctrl Pts',(-0.0196449142058159,0.0116335810938962,
-0.00813024414775876));
#51242=CARTESIAN_POINT('Ctrl Pts',(-0.0196207606883723,0.0116341247629989,
-0.00814046602788445));
#51243=CARTESIAN_POINT('Ctrl Pts',(-0.0195962052881846,0.0116346427084887,
-0.00815087403226374));
#51244=CARTESIAN_POINT('Ctrl Pts',(-0.0195711189395796,0.0116351346995956,
-0.00816152452180743));
#51245=CARTESIAN_POINT('Ctrl Pts',(-0.0194932364967061,0.0116366621227324,
-0.00819458976205108));
#51246=CARTESIAN_POINT('Ctrl Pts',(-0.0194102431613973,0.011637893906005,
-0.00823001122447739));
#51247=CARTESIAN_POINT('Ctrl Pts',(-0.0193375775331837,0.0116387231160456,
-0.00826116194303029));
#51248=CARTESIAN_POINT('Ctrl Pts',(-0.0193208662193722,0.0116389138140351,
-0.00826832584494639));
#51249=CARTESIAN_POINT('Ctrl Pts',(-0.0193047009403302,0.0116390852850543,
-0.00827526292998242));
#51250=CARTESIAN_POINT('Ctrl Pts',(-0.0192892688892072,0.0116392393051141,
-0.00828189123357834));
#51251=CARTESIAN_POINT('Ctrl Pts',(-0.0192067338142212,0.0116400630489629,
-0.00831734131924469));
#51252=CARTESIAN_POINT('Ctrl Pts',(-0.0191451581260807,0.0116403309325968,
-0.00834392987291784));
#51253=CARTESIAN_POINT('Ctrl Pts',(-0.0190762821376132,0.0116404432600024,
-0.00837376746968747));
#51254=CARTESIAN_POINT('Ctrl Pts',(-0.0190074061491457,0.011640555587408,
-0.0084036050664571));
#51255=CARTESIAN_POINT('Ctrl Pts',(-0.0189312438411869,0.011640467183901,
-0.00843672720352299));
#51256=CARTESIAN_POINT('Ctrl Pts',(-0.0188545740569457,0.0116400805608009,
-0.00847022736541512));
#51257=CARTESIAN_POINT('Ctrl Pts',(-0.0185478949199809,0.0116385340684007,
-0.00860422801298365));
#51258=CARTESIAN_POINT('Ctrl Pts',(-0.0182334449138913,0.0116327418153481,
-0.00874381723191419));
#51259=CARTESIAN_POINT('Ctrl Pts',(-0.0178774831716006,0.0116210616437134,
-0.00890496724854988));
#51260=CARTESIAN_POINT('Ctrl Pts',(-0.0176995023004553,0.011615221557896,
-0.00898554225686772));
#51261=CARTESIAN_POINT('Ctrl Pts',(-0.0175110655021848,0.0116077564505905,
-0.00907164313857367));
#51262=CARTESIAN_POINT('Ctrl Pts',(-0.0173323249853488,0.0115996854662668,
-0.00915403466834566));
#51263=CARTESIAN_POINT('Ctrl Pts',(-0.0173258280195924,0.0115993920973671,
-0.00915702948427783));
#51264=CARTESIAN_POINT('Ctrl Pts',(-0.0173193437858001,0.0115990978659295,
-0.00916001936559306));
#51265=CARTESIAN_POINT('Ctrl Pts',(-0.0173128720265079,0.0115988027869249,
-0.00916300441835151));
#51266=CARTESIAN_POINT('Ctrl Pts',(-0.016963249681542,0.0115828618025859,
-0.00932426522830298));
#51267=CARTESIAN_POINT('Ctrl Pts',(-0.0166501932368521,0.011564718427035,
-0.00947114780149651));
#51268=CARTESIAN_POINT('Ctrl Pts',(-0.0163378303803881,0.0115430555440284,
-0.009619580783559));
#51269=CARTESIAN_POINT('Ctrl Pts',(-0.0163272006767041,0.0115423183564193,
-0.00962463195588502));
#51270=CARTESIAN_POINT('Ctrl Pts',(-0.0163165717881284,0.0115415774297594,
-0.00962968513938956));
#51271=CARTESIAN_POINT('Ctrl Pts',(-0.0163059450208025,0.0115408327300449,
-0.00963473971397893));
#51272=CARTESIAN_POINT('Ctrl Pts',(-0.015998514756725,0.0115192887154964,
-0.00978096755102024));
#51273=CARTESIAN_POINT('Ctrl Pts',(-0.0156922675390135,0.0114944014941102,
-0.00992875512006374));
#51274=CARTESIAN_POINT('Ctrl Pts',(-0.0153993022433853,0.0114667765373308,
-0.0100716954734317));
#51275=CARTESIAN_POINT('Ctrl Pts',(-0.0153166543934544,0.0074999794584345,
-0.010121177809007));
#51276=CARTESIAN_POINT('Ctrl Pts',(-0.0153260430540535,0.00792901066112673,
-0.0101156468647559));
#51277=CARTESIAN_POINT('Ctrl Pts',(-0.015335030986271,0.00834507843141892,
-0.0101103306587591));
#51278=CARTESIAN_POINT('Ctrl Pts',(-0.0153436173262386,0.00874821533256098,
-0.0101052264670943));
#51279=CARTESIAN_POINT('Ctrl Pts',(-0.0153527877473525,0.00917877540402363,
-0.0100997750655438));
#51280=CARTESIAN_POINT('Ctrl Pts',(-0.0153615002389735,0.00959458555346814,
-0.010094565527106));
#51281=CARTESIAN_POINT('Ctrl Pts',(-0.0153697578474766,0.00999565020811485,
-0.0100895982399535));
#51282=CARTESIAN_POINT('Ctrl Pts',(-0.015378671278209,0.0104285675614914,
-0.0100842364490736));
#51283=CARTESIAN_POINT('Ctrl Pts',(-0.0153870543983629,0.0108443042696742,
-0.0100791569642583));
#51284=CARTESIAN_POINT('Ctrl Pts',(-0.015394903833982,0.0112428257310516,
-0.010074363848708));
#51285=CARTESIAN_POINT('Ctrl Pts',(-0.015396386273589,0.0113180902503411,
-0.0100734586238386));
#51286=CARTESIAN_POINT('Ctrl Pts',(-0.015397849684388,0.0113927406309423,
-0.0100725636187554));
#51287=CARTESIAN_POINT('Ctrl Pts',(-0.0153992941382262,0.0114667764973816,
-0.0100716788736061));
#51288=CARTESIAN_POINT('Ctrl Pts',(-0.0312862281526355,0.00944638107869527,
-0.00512344313018988));
#51289=CARTESIAN_POINT('Ctrl Pts',(-0.0314562756363666,0.00945826354092308,
-0.00509821111361097));
#51290=CARTESIAN_POINT('Ctrl Pts',(-0.0316300000451325,0.00947077019190787,
-0.00507294851419576));
#51291=CARTESIAN_POINT('Ctrl Pts',(-0.0318165997466437,0.00948464848780534,
-0.00504641821905065));
#51292=CARTESIAN_POINT('Ctrl Pts',(-0.0318632496720215,0.00948811806177971,
-0.00503978564526438));
#51293=CARTESIAN_POINT('Ctrl Pts',(-0.0319107047314941,0.00949167410932467,
-0.00503307702218328));
#51294=CARTESIAN_POINT('Ctrl Pts',(-0.0319555148891595,0.00949505711749807,
-0.00502677439109328));
#51295=CARTESIAN_POINT('Ctrl Pts',(-0.0320003250468249,0.00949844012567147,
-0.00502047176000328));
#51296=CARTESIAN_POINT('Ctrl Pts',(-0.0320424889665942,0.00950164756885702,
-0.00501456480075179));
#51297=CARTESIAN_POINT('Ctrl Pts',(-0.0320969589552305,0.00950581482965032,
-0.00500698754389991));
#51298=CARTESIAN_POINT('Ctrl Pts',(-0.032205898932503,0.0095141493512369,
-0.00499183303019616));
#51299=CARTESIAN_POINT('Ctrl Pts',(-0.032364079079264,0.00952635477605135,
-0.0049701229080083));
#51300=CARTESIAN_POINT('Ctrl Pts',(-0.0325078832619222,0.00953752434301051,
-0.00495080406393419));
#51301=CARTESIAN_POINT('Ctrl Pts',(-0.0326516874445805,0.00954869390996967,
-0.00493148521986007));
#51302=CARTESIAN_POINT('Ctrl Pts',(-0.0327811014399474,0.00955879432134487,
-0.00491443693059583));
#51303=CARTESIAN_POINT('Ctrl Pts',(-0.0329095981928218,0.00956888639698524,
-0.0048977528006591));
#51304=CARTESIAN_POINT('Ctrl Pts',(-0.0329276637186178,0.00957030525503992,
-0.00489540715710769));
#51305=CARTESIAN_POINT('Ctrl Pts',(-0.0329457110008698,0.00957172411000436,
-0.00489306911910923));
#51306=CARTESIAN_POINT('Ctrl Pts',(-0.0329637309158827,0.00957314220261207,
-0.00489073980242877));
#51307=CARTESIAN_POINT('Ctrl Pts',(-0.0330738833326562,0.00958181074116154,
-0.00487650111919418));
#51308=CARTESIAN_POINT('Ctrl Pts',(-0.0331830176598123,0.00959045057343606,
-0.00486259022841222));
#51309=CARTESIAN_POINT('Ctrl Pts',(-0.033289018186645,0.00959889021079495,
-0.00484924797714197));
#51310=CARTESIAN_POINT('Ctrl Pts',(-0.0335357006488678,0.00961853077849934,
-0.00481819813717152));
#51311=CARTESIAN_POINT('Ctrl Pts',(-0.0337654170511146,0.00963707680202003,
-0.00479020187725715));
#51312=CARTESIAN_POINT('Ctrl Pts',(-0.0339807978056659,0.00965465621567979,
-0.00476455503025098));
#51313=CARTESIAN_POINT('Ctrl Pts',(-0.0341961785602172,0.00967223562933955,
-0.0047389081832448));
#51314=CARTESIAN_POINT('Ctrl Pts',(-0.0343972246080754,0.00968885149610345,
-0.00471562001397164));
#51315=CARTESIAN_POINT('Ctrl Pts',(-0.0345829605600567,0.00970430948850187,
-0.00469454328516853));
#51316=CARTESIAN_POINT('Ctrl Pts',(-0.0347686965120379,0.00971976748090028,
-0.00467346655636542));
#51317=CARTESIAN_POINT('Ctrl Pts',(-0.0349391223186177,0.00973406623614095,
-0.00465459899770515));
#51318=CARTESIAN_POINT('Ctrl Pts',(-0.0350953496941226,0.00974715838514988,
-0.00463763982327587));
#51319=CARTESIAN_POINT('Ctrl Pts',(-0.0352515770696274,0.0097602505341588,
-0.00462068064884658));
#51320=CARTESIAN_POINT('Ctrl Pts',(-0.0353936065559122,0.00977213873693642,
-0.00460563662168135));
#51321=CARTESIAN_POINT('Ctrl Pts',(-0.0355178737630501,0.00978245291917888,
-0.00459271866193936));
#51322=CARTESIAN_POINT('Ctrl Pts',(-0.035642140970188,0.00979276710142133,
-0.00457980070219737));
#51323=CARTESIAN_POINT('Ctrl Pts',(-0.0357486448359685,0.00980150018491219,
-0.00456899286053882));
#51324=CARTESIAN_POINT('Ctrl Pts',(-0.0358504812553988,0.00980947077143243,
-0.0045589750680604));
#51325=CARTESIAN_POINT('Ctrl Pts',(-0.035901399465114,0.00981345606469256,
-0.00455396617182119));
#51326=CARTESIAN_POINT('Ctrl Pts',(-0.0359511514008514,0.00981725524023119,
-0.00454916449715817));
#51327=CARTESIAN_POINT('Ctrl Pts',(-0.0359830568732576,0.00981967355013075,
-0.00454610807859423));
#51328=CARTESIAN_POINT('Ctrl Pts',(-0.0359990096094606,0.00982088270508053,
-0.00454457986931226));
#51329=CARTESIAN_POINT('Ctrl Pts',(-0.036010500404943,0.00982174404162896,
-0.00454348243588464));
#51330=CARTESIAN_POINT('Ctrl Pts',(-0.0360409115717217,0.00982391760366982,
-0.00454065001146376));
#51331=CARTESIAN_POINT('Ctrl Pts',(-0.0360713227385004,0.00982609116571067,
-0.00453781758704287));
#51332=CARTESIAN_POINT('Ctrl Pts',(-0.0361206549855137,0.00982958271525947,
-0.00453326238401915));
#51333=CARTESIAN_POINT('Ctrl Pts',(-0.0361678405239929,0.00983286823482105,
-0.00452897731231815));
#51334=CARTESIAN_POINT('Ctrl Pts',(-0.0362622116009512,0.0098394392739442,
-0.00452040716891616));
#51335=CARTESIAN_POINT('Ctrl Pts',(-0.0363479935782716,0.00984516645782268,
-0.00451287649901968));
#51336=CARTESIAN_POINT('Ctrl Pts',(-0.0364361982614431,0.00985086055000014,
-0.00450536150740648));
#51337=CARTESIAN_POINT('Ctrl Pts',(-0.0365244029446146,0.00985655464217761,
-0.00449784651579328));
#51338=CARTESIAN_POINT('Ctrl Pts',(-0.0366150308907188,0.00986222133347914,
-0.00449035860128791));
#51339=CARTESIAN_POINT('Ctrl Pts',(-0.0367053796526332,0.0098676622596607,
-0.00448315369924367));
#51340=CARTESIAN_POINT('Ctrl Pts',(-0.0368860771764619,0.00987854411202381,
-0.00446874389515518));
#51341=CARTESIAN_POINT('Ctrl Pts',(-0.0370656574686301,0.00988851651328245,
-0.00445545394930328));
#51342=CARTESIAN_POINT('Ctrl Pts',(-0.0372462195336707,0.00989774443788289,
-0.00444316275356318));
#51343=CARTESIAN_POINT('Ctrl Pts',(-0.0374267815987114,0.00990697236248332,
-0.00443087155782307));
#51344=CARTESIAN_POINT('Ctrl Pts',(-0.037608325543134,0.00991545838883364,
-0.00441958371644594));
#51345=CARTESIAN_POINT('Ctrl Pts',(-0.0377903686107517,0.00992317554436644,
-0.00440939607922095));
#51346=CARTESIAN_POINT('Ctrl Pts',(-0.0385185405140091,0.00995404415093073,
-0.00436864555087132));
#51347=CARTESIAN_POINT('Ctrl Pts',(-0.0392547002352749,0.00997273853647701,
-0.00434575504846055));
#51348=CARTESIAN_POINT('Ctrl Pts',(-0.0399999969037804,0.00997686116634681,
-0.00434340405242746));
#51349=CARTESIAN_POINT('Origin',(-0.14,0.0075,0.));
#51350=CARTESIAN_POINT('',(-0.14,0.0075,-0.004));
#51351=CARTESIAN_POINT('Origin',(-0.14,0.0075,0.));
#51352=CARTESIAN_POINT('Origin',(-0.0475,0.0025,4.33680868994202E-19));
#51353=CARTESIAN_POINT('Ctrl Pts',(-0.0475,0.00292794117647059,0.00143766002569487));
#51354=CARTESIAN_POINT('Ctrl Pts',(-0.0475073233962253,0.00292794075855509,
0.00143766066444556));
#51355=CARTESIAN_POINT('Ctrl Pts',(-0.0475146468511719,0.00292791816889614,
0.00143760919648263));
#51356=CARTESIAN_POINT('Ctrl Pts',(-0.047521969610817,0.00292787381968359,
0.0014375057980809));
#51357=CARTESIAN_POINT('Origin',(-0.0675,0.0025,4.33680868994202E-19));
#51358=CARTESIAN_POINT('Ctrl Pts',(-0.0675,0.00292794117647059,0.00143766002569488));
#51359=CARTESIAN_POINT('Ctrl Pts',(-0.0675073233962253,0.00292794075855509,
0.00143766066444556));
#51360=CARTESIAN_POINT('Ctrl Pts',(-0.0675146468511718,0.00292791816889614,
0.00143760919648264));
#51361=CARTESIAN_POINT('Ctrl Pts',(-0.067521969610817,0.00292787381968359,
0.00143750579808091));
#51362=CARTESIAN_POINT('Origin',(-0.0875,0.0025,4.33680868994202E-19));
#51363=CARTESIAN_POINT('Ctrl Pts',(-0.0875,0.00292794117647059,0.00143766002569487));
#51364=CARTESIAN_POINT('Ctrl Pts',(-0.0875073233962253,0.00292794075855509,
0.00143766066444556));
#51365=CARTESIAN_POINT('Ctrl Pts',(-0.0875146468511718,0.00292791816889614,
0.00143760919648263));
#51366=CARTESIAN_POINT('Ctrl Pts',(-0.087521969610817,0.00292787381968359,
0.00143750579808091));
#51367=CARTESIAN_POINT('Origin',(-0.1075,0.0025,4.33680868994202E-19));
#51368=CARTESIAN_POINT('Ctrl Pts',(-0.1075,0.00292794117647059,0.00143766002569487));
#51369=CARTESIAN_POINT('Ctrl Pts',(-0.107507323396225,0.00292794075855509,
0.00143766066444556));
#51370=CARTESIAN_POINT('Ctrl Pts',(-0.107514646851172,0.00292791816889614,
0.00143760919648263));
#51371=CARTESIAN_POINT('Ctrl Pts',(-0.107521969610817,0.00292787381968359,
0.0014375057980809));
#51372=CARTESIAN_POINT('Origin',(-0.1275,0.0025,4.33680868994202E-19));
#51373=CARTESIAN_POINT('Ctrl Pts',(-0.1275,0.00292794117647059,0.00143766002569487));
#51374=CARTESIAN_POINT('Ctrl Pts',(-0.127507323396225,0.00292794075855509,
0.00143766066444555));
#51375=CARTESIAN_POINT('Ctrl Pts',(-0.127514646851172,0.00292791816889614,
0.00143760919648263));
#51376=CARTESIAN_POINT('Ctrl Pts',(-0.127521969610817,0.00292787381968359,
0.0014375057980809));
#51377=CARTESIAN_POINT('Origin',(0.00396253460616978,-0.0267643850402721,
0.));
#51378=CARTESIAN_POINT('',(-0.00847413551306003,0.0012,-0.00451935750764788));
#51379=CARTESIAN_POINT('',(-0.000426041560703257,0.0012,-0.0124834192096569));
#51380=CARTESIAN_POINT('Origin',(0.00396253460616978,0.0012,0.));
#51381=CARTESIAN_POINT('',(-0.000426041560703257,0.0128,-0.0124834192096569));
#51382=CARTESIAN_POINT('',(-0.000426041560703257,-0.0267643850402721,-0.0124834192096569));
#51383=CARTESIAN_POINT('',(-0.00847413551306003,0.0128,-0.00451935750764788));
#51384=CARTESIAN_POINT('Origin',(0.00396253460616978,0.0128,0.));
#51385=CARTESIAN_POINT('',(-0.00847413551306003,-0.0267643850402721,-0.00451935750764788));
#51386=CARTESIAN_POINT('Origin',(-0.00926982557395217,0.0172426406871193,
-0.003));
#51387=CARTESIAN_POINT('',(-0.0087336051435635,0.0128,-0.00440088102636655));
#51388=CARTESIAN_POINT('',(-0.0087336051435635,0.0172426406871193,-0.00440088102636655));
#51389=CARTESIAN_POINT('Origin',(-0.00926982557395217,0.0128,-0.003));
#51390=CARTESIAN_POINT('Origin',(-0.00926982557395217,0.0172426406871193,
0.003));
#51391=CARTESIAN_POINT('',(-0.0087336051435635,0.0128,0.00440088102636655));
#51392=CARTESIAN_POINT('Origin',(-0.00926982557395217,0.0128,0.003));
#51393=CARTESIAN_POINT('',(-0.0087336051435635,0.0172426406871193,0.00440088102636655));
#51394=CARTESIAN_POINT('Origin',(0.0125,0.0134,-4.59242549680257E-18));
#51395=CARTESIAN_POINT('',(-0.0218619061298847,0.0134036502117966,-0.00614822711587315));
#51396=CARTESIAN_POINT('',(-0.0246662622795289,0.0133985587966785,-0.00446937813281868));
#51397=CARTESIAN_POINT('Ctrl Pts',(-0.0218616087263876,0.0134072500816831,
-0.00614770820245367));
#51398=CARTESIAN_POINT('Ctrl Pts',(-0.0224316181952039,0.0134051358023753,
-0.00580540362823925));
#51399=CARTESIAN_POINT('Ctrl Pts',(-0.0229504127578444,0.0134033860935674,
-0.00549445185996141));
#51400=CARTESIAN_POINT('Ctrl Pts',(-0.0234178523021115,0.0134019533441035,
-0.00521477645854381));
#51401=CARTESIAN_POINT('Ctrl Pts',(-0.0238852918463787,0.0134005205946397,
-0.00493510105712622));
#51402=CARTESIAN_POINT('Ctrl Pts',(-0.0243013762672867,0.0133994057486489,
-0.00468670177378412));
#51403=CARTESIAN_POINT('Ctrl Pts',(-0.0246662622795289,0.0133985587966785,
-0.00446937813281868));
#51404=CARTESIAN_POINT('',(-0.0306437028537828,0.013404764132741,-0.000979164530978816));
#51405=CARTESIAN_POINT('Ctrl Pts',(-0.0246662622795289,0.0133985587966785,
-0.00446937813281868));
#51406=CARTESIAN_POINT('Ctrl Pts',(-0.02484870528565,0.0133981353206933,
-0.00436071631233596));
#51407=CARTESIAN_POINT('Ctrl Pts',(-0.0250183490525746,0.0133977787570224,
-0.00425982399334597));
#51408=CARTESIAN_POINT('Ctrl Pts',(-0.0251749322827964,0.0133974820191827,
-0.00416684462913048));
#51409=CARTESIAN_POINT('Ctrl Pts',(-0.0253315155130181,0.013397185281343,
-0.004073865264915));
#51410=CARTESIAN_POINT('Ctrl Pts',(-0.0254750382134319,0.0133969481647494,
-0.00398879886795332));
#51411=CARTESIAN_POINT('Ctrl Pts',(-0.0256065444454201,0.0133967612769716,
-0.00391103173174672));
#51412=CARTESIAN_POINT('Ctrl Pts',(-0.0257380506774083,0.0133965743891938,
-0.00383326459554012));
#51413=CARTESIAN_POINT('Ctrl Pts',(-0.0258575404382745,0.0133964384141437,
-0.00376279671161932));
#51414=CARTESIAN_POINT('Ctrl Pts',(-0.0259610836783824,0.013396345373031,
-0.00370191490119503));
#51415=CARTESIAN_POINT('Ctrl Pts',(-0.0260128552984361,0.0133962988524746,
-0.00367147399598301));
#51416=CARTESIAN_POINT('Ctrl Pts',(-0.026060640319222,0.0133962626606343,
-0.00364342966218188));
#51417=CARTESIAN_POINT('Ctrl Pts',(-0.0261094483981875,0.01339623361188,
-0.00361486343215608));
#51418=CARTESIAN_POINT('Ctrl Pts',(-0.0261216504179288,0.0133962263496915,
-0.0036077218746497));
#51419=CARTESIAN_POINT('Ctrl Pts',(-0.026133916378215,0.0133962195615091,
-0.00360054769753044));
#51420=CARTESIAN_POINT('Ctrl Pts',(-0.0261453683469057,0.0133962135826212,
-0.00359385233772909));
#51421=CARTESIAN_POINT('Ctrl Pts',(-0.0261568203155964,0.0133962076037333,
-0.00358715697792774));
#51422=CARTESIAN_POINT('Ctrl Pts',(-0.0261674582927879,0.0133962024308566,
-0.00358094043562296));
#51423=CARTESIAN_POINT('Ctrl Pts',(-0.026176404350354,0.0133961982804328,
-0.00357571415486204));
#51424=CARTESIAN_POINT('Ctrl Pts',(-0.0261942964654848,0.0133961899795853,
-0.00356526159334099));
#51425=CARTESIAN_POINT('Ctrl Pts',(-0.026205420924764,0.0133961850720793,
-0.00355877011808311));
#51426=CARTESIAN_POINT('Ctrl Pts',(-0.0262385426891691,0.0133961752170391,
-0.00353948251138114));
#51427=CARTESIAN_POINT('Ctrl Pts',(-0.0262716644535742,0.013396165361999,
-0.00352019490467917));
#51428=CARTESIAN_POINT('Ctrl Pts',(-0.0263267834553753,0.0133961525896145,
-0.00348811104702352));
#51429=CARTESIAN_POINT('Ctrl Pts',(-0.0263761483878874,0.0133961459372958,
-0.00345937581224427));
#51430=CARTESIAN_POINT('Ctrl Pts',(-0.0264255133203996,0.0133961392849771,
-0.00343064057746502));
#51431=CARTESIAN_POINT('Ctrl Pts',(-0.0264691242400881,0.0133961370250713,
-0.00340525406450762));
#51432=CARTESIAN_POINT('Ctrl Pts',(-0.0265137570553487,0.0133961377888301,
-0.00337927420988169));
#51433=CARTESIAN_POINT('Ctrl Pts',(-0.0266030226858698,0.0133961393163476,
-0.00332731450062983));
#51434=CARTESIAN_POINT('Ctrl Pts',(-0.0266963758413186,0.013396154777692,
-0.00327298132539457));
#51435=CARTESIAN_POINT('Ctrl Pts',(-0.0267889834642484,0.0133961847528988,
-0.00321908664941024));
#51436=CARTESIAN_POINT('Ctrl Pts',(-0.0269741987101078,0.0133962447033124,
-0.00311129729744156));
#51437=CARTESIAN_POINT('Ctrl Pts',(-0.0271564318922438,0.0133963600240961,
-0.00300526205486268));
#51438=CARTESIAN_POINT('Ctrl Pts',(-0.0273394739295583,0.0133965307135107,
-0.00289877688381003));
#51439=CARTESIAN_POINT('Ctrl Pts',(-0.0275225159668727,0.0133967014029252,
-0.00279229171275739));
#51440=CARTESIAN_POINT('Ctrl Pts',(-0.0277063668386704,0.0133969284195639,
-0.00268535658059987));
#51441=CARTESIAN_POINT('Ctrl Pts',(-0.0278900176482774,0.013397210548563,
-0.00257856036789178));
#51442=CARTESIAN_POINT('Ctrl Pts',(-0.0280736684578844,0.0133974926775621,
-0.00247176415518369));
#51443=CARTESIAN_POINT('Ctrl Pts',(-0.0282571192073703,0.0133978296700538,
-0.00236510686401149));
#51444=CARTESIAN_POINT('Ctrl Pts',(-0.0284406190592505,0.0133982212239526,
-0.00225844573750197));
#51445=CARTESIAN_POINT('Ctrl Pts',(-0.0288076187630104,0.0133990043317502,
-0.00204512348448318));
#51446=CARTESIAN_POINT('Ctrl Pts',(-0.0291748147033377,0.013400006110592,
-0.00183178560108586));
#51447=CARTESIAN_POINT('Ctrl Pts',(-0.0295420174056225,0.0134012198710319,
-0.0016185646073897));
#51448=CARTESIAN_POINT('Ctrl Pts',(-0.0299092201079074,0.0134024336314718,
-0.00140534361369354));
#51449=CARTESIAN_POINT('Ctrl Pts',(-0.0302764295548016,0.0134038593389672,
-0.00119223948020539));
#51450=CARTESIAN_POINT('Ctrl Pts',(-0.0306437239536334,0.0134054880398384,
-0.000979235456812336));
#51451=CARTESIAN_POINT('',(-0.0306436021829707,0.0134038303428005,0.000979384968266446));
#51452=CARTESIAN_POINT('Ctrl Pts',(-0.0306436988839239,0.0134001848071171,
-0.00097915009888143));
#51453=CARTESIAN_POINT('Ctrl Pts',(-0.0308844167416533,0.013400058464486,
-0.000838923509007557));
#51454=CARTESIAN_POINT('Ctrl Pts',(-0.031065303511043,0.0133999548660539,
-0.000605834760277834));
#51455=CARTESIAN_POINT('Ctrl Pts',(-0.0311468606481766,0.0133999055193688,
-0.000343687857538236));
#51456=CARTESIAN_POINT('Ctrl Pts',(-0.0311814513686478,0.0133998845900247,
-0.000232503839146404));
#51457=CARTESIAN_POINT('Ctrl Pts',(-0.0311988532204896,0.0133998706262688,
-0.000116311864112296));
#51458=CARTESIAN_POINT('Ctrl Pts',(-0.0311987881631695,0.013399869793343,
-2.04344619827451E-7));
#51459=CARTESIAN_POINT('Ctrl Pts',(-0.0311986370453371,0.0133998678585886,
0.000269495000961271));
#51460=CARTESIAN_POINT('Ctrl Pts',(-0.0311014259137929,0.0133999302301344,
0.00054031925079773));
#51461=CARTESIAN_POINT('Ctrl Pts',(-0.0309232168780912,0.0134000273529956,
0.000746743782210436));
#51462=CARTESIAN_POINT('Ctrl Pts',(-0.0308438164757785,0.0134000706257411,
0.000838715498329324));
#51463=CARTESIAN_POINT('Ctrl Pts',(-0.0307490092605827,0.0134001278742394,
0.000917856093433611));
#51464=CARTESIAN_POINT('Ctrl Pts',(-0.0306435804364503,0.0134001832092226,
0.00097927422772854));
#51465=CARTESIAN_POINT('',(-0.0245961457050751,0.0133984902066176,0.00450908869591151));
#51466=CARTESIAN_POINT('Ctrl Pts',(-0.030643579828093,0.0134054497566434,
0.000979354044147875));
#51467=CARTESIAN_POINT('Ctrl Pts',(-0.0302704345009344,0.0134038023831892,
0.00119668648055279));
#51468=CARTESIAN_POINT('Ctrl Pts',(-0.0298972641109317,0.0134023788653426,
0.00141392650844518));
#51469=CARTESIAN_POINT('Ctrl Pts',(-0.0295239969009407,0.0134011751550314,
0.00163111223813555));
#51470=CARTESIAN_POINT('Ctrl Pts',(-0.0291507239793726,0.0133999714263015,
0.00184830129111021));
#51471=CARTESIAN_POINT('Ctrl Pts',(-0.028777354208528,0.0133989876278009,
0.00206543600036375));
#51472=CARTESIAN_POINT('Ctrl Pts',(-0.0284040972083492,0.0133982196073921,
0.00228238672419007));
#51473=CARTESIAN_POINT('Ctrl Pts',(-0.0282174687082596,0.0133978355971879,
0.00239086208610336));
#51474=CARTESIAN_POINT('Ctrl Pts',(-0.0280308683699045,0.0133975054496782,
0.00249929139868863));
#51475=CARTESIAN_POINT('Ctrl Pts',(-0.02784402991443,0.0133972282005621,
0.00260782754683863));
#51476=CARTESIAN_POINT('Ctrl Pts',(-0.0276571914589556,0.013396950951446,
0.00271636369498863));
#51477=CARTESIAN_POINT('Ctrl Pts',(-0.0274701148862677,0.0133967268540346,
0.00282500668007215));
#51478=CARTESIAN_POINT('Ctrl Pts',(-0.0272838802758687,0.0133965560148374,
0.00293312914716413));
#51479=CARTESIAN_POINT('Ctrl Pts',(-0.0270976456654697,0.0133963851756403,
0.00304125161425611));
#51480=CARTESIAN_POINT('Ctrl Pts',(-0.0269122530287835,0.0133962666334186,
0.00314885357996413));
#51481=CARTESIAN_POINT('Ctrl Pts',(-0.026723644556908,0.0133961988639523,
0.00325828413831277));
#51482=CARTESIAN_POINT('Ctrl Pts',(-0.0266293403209695,0.0133961649792191,
0.00331299941748751));
#51483=CARTESIAN_POINT('Ctrl Pts',(-0.0265342321084859,0.0133961444583619,
0.00336817181498661));
#51484=CARTESIAN_POINT('Ctrl Pts',(-0.0264434931177796,0.0133961370186881,
0.00342080412543893));
#51485=CARTESIAN_POINT('Ctrl Pts',(-0.0263981236224262,0.0133961332988513,
0.00344712028066522));
#51486=CARTESIAN_POINT('Ctrl Pts',(-0.0263538464463589,0.0133961323911641,
0.00347280143798082));
#51487=CARTESIAN_POINT('Ctrl Pts',(-0.0263034087596331,0.0133961350177981,
0.00350204927193081));
#51488=CARTESIAN_POINT('Ctrl Pts',(-0.0262529710729073,0.0133961376444321,
0.00353129710588081));
#51489=CARTESIAN_POINT('Ctrl Pts',(-0.0261963728170893,0.0133961455241088,
0.00356411151466535));
#51490=CARTESIAN_POINT('Ctrl Pts',(-0.0261633185455084,0.0133961521945727,
0.00358328433450696));
#51491=CARTESIAN_POINT('Ctrl Pts',(-0.0261302642739275,0.0133961588650367,
0.00360245715434857));
#51492=CARTESIAN_POINT('Ctrl Pts',(-0.0261207540577249,0.013396162339358,
0.00360798850995018));
#51493=CARTESIAN_POINT('Ctrl Pts',(-0.0261040014070238,0.013396168779049,
0.00361774460599147));
#51494=CARTESIAN_POINT('Ctrl Pts',(-0.0260872487563228,0.0133961752187401,
0.00362750070203276));
#51495=CARTESIAN_POINT('Ctrl Pts',(-0.0260632536437238,0.0133961853949361,
0.003641481490354));
#51496=CARTESIAN_POINT('Ctrl Pts',(-0.0260395330951174,0.0133961977045661,
0.00365532466296406));
#51497=CARTESIAN_POINT('Ctrl Pts',(-0.0260336029579654,0.0133962007819736,
0.00365878545611685));
#51498=CARTESIAN_POINT('Ctrl Pts',(-0.0260276899814467,0.0133962039823826,
0.0036622376489649));
#51499=CARTESIAN_POINT('Ctrl Pts',(-0.0260217836934467,0.0133962073090115,
0.00366568731888552));
#51500=CARTESIAN_POINT('Ctrl Pts',(-0.0260166156914465,0.0133962102198117,
0.00366870578006609));
#51501=CARTESIAN_POINT('Ctrl Pts',(-0.0260114528103434,0.0133962132272588,
0.00367172230963));
#51502=CARTESIAN_POINT('Ctrl Pts',(-0.0260062880346306,0.0133962163339297,
0.00367474097893365));
#51503=CARTESIAN_POINT('Ctrl Pts',(-0.0259701346046417,0.0133962380806259,
0.00369587166405896));
#51504=CARTESIAN_POINT('Ctrl Pts',(-0.0259338883400778,0.0133962646035691,
0.00371710719892812));
#51505=CARTESIAN_POINT('Ctrl Pts',(-0.0258951429137755,0.0133962973664198,
0.00373984404161307));
#51506=CARTESIAN_POINT('Ctrl Pts',(-0.0257939303715984,0.0133963829510096,
0.00379923824291234));
#51507=CARTESIAN_POINT('Ctrl Pts',(-0.0256756638564315,0.0133965123590765,
0.00386887687484338));
#51508=CARTESIAN_POINT('Ctrl Pts',(-0.0255445494680514,0.0133966946948038,
0.00394632154718793));
#51509=CARTESIAN_POINT('Ctrl Pts',(-0.0254134350796713,0.0133968770305312,
0.00402376621953248));
#51510=CARTESIAN_POINT('Ctrl Pts',(-0.0252694728254696,0.0133971115725649,
0.00410901694869879));
#51511=CARTESIAN_POINT('Ctrl Pts',(-0.0251115451843419,0.0133974079443082,
0.00420272793954665));
#51512=CARTESIAN_POINT('Ctrl Pts',(-0.0249536175432143,0.0133977043160516,
0.00429643893039451));
#51513=CARTESIAN_POINT('Ctrl Pts',(-0.0247817245066117,0.0133980627385854,
0.00439861016754807));
#51514=CARTESIAN_POINT('Ctrl Pts',(-0.0245961457050751,0.0133984902066176,
0.00450908869591151));
#51515=CARTESIAN_POINT('',(-0.0217115430864154,0.013403672751003,0.00623566005618913));
#51516=CARTESIAN_POINT('Ctrl Pts',(-0.0245961457050751,0.0133984902066176,
0.00450908869591151));
#51517=CARTESIAN_POINT('Ctrl Pts',(-0.0242249881020029,0.0133993451426819,
0.00473004575263784));
#51518=CARTESIAN_POINT('Ctrl Pts',(-0.0237990859267062,0.0134004767238543,
0.00498422950764963));
#51519=CARTESIAN_POINT('Ctrl Pts',(-0.0233182712556556,0.0134019301764394,
0.00527185391241485));
#51520=CARTESIAN_POINT('Ctrl Pts',(-0.0228374565846051,0.0134033836290245,
0.00555947831718007));
#51521=CARTESIAN_POINT('Ctrl Pts',(-0.0223017296223626,0.0134051576682972,
0.00588054379428986));
#51522=CARTESIAN_POINT('Ctrl Pts',(-0.0217112388916228,0.0134072933313472,
0.00623513020576297));
#51523=CARTESIAN_POINT('',(-0.0196330755873382,0.013399961279499,0.00732918595449924));
#51524=CARTESIAN_POINT('Ctrl Pts',(-0.0217107156962388,0.0134,0.00623430285898128));
#51525=CARTESIAN_POINT('Ctrl Pts',(-0.0210382714245267,0.0134,0.00663741032810192));
#51526=CARTESIAN_POINT('Ctrl Pts',(-0.0203387252089173,0.0134,0.00698909350869522));
#51527=CARTESIAN_POINT('Ctrl Pts',(-0.0196330752480917,0.0134,0.00732918602429228));
#51528=CARTESIAN_POINT('',(-0.0170139362062251,0.0134,0.00887744578929155));
#51529=CARTESIAN_POINT('',(-0.0169180511005122,0.0134,0.00893412666903227));
#51530=CARTESIAN_POINT('',(-0.00395280707079757,0.0134,0.00203751601562436));
#51531=CARTESIAN_POINT('',(0.00979635300466746,0.0134,-0.0051627258920988));
#51532=CARTESIAN_POINT('',(-0.00395280707079757,0.0134,-0.00203751601562436));
#51533=CARTESIAN_POINT('Origin',(-0.00501982557395217,0.0134,-2.16840434497101E-19));
#51534=CARTESIAN_POINT('',(-0.0170139362062251,0.0134,-0.00887744578929154));
#51535=CARTESIAN_POINT('',(0.00979635300466746,0.0134,0.0051627258920988));
#51536=CARTESIAN_POINT('',(-0.0198053127327029,0.0133999927310859,-0.00722737050826749));
#51537=CARTESIAN_POINT('',(-0.021610272031846,0.0134,-0.00616039858740607));
#51538=CARTESIAN_POINT('Ctrl Pts',(-0.0198053128281438,0.0134,-0.0072273706664189));
#51539=CARTESIAN_POINT('Ctrl Pts',(-0.0205037791748502,0.0134,-0.00689234317033915));
#51540=CARTESIAN_POINT('Ctrl Pts',(-0.0211960792182919,0.0134,-0.00654557458054435));
#51541=CARTESIAN_POINT('Ctrl Pts',(-0.0218610959359586,0.0134,-0.00614689907887388));
#51542=CARTESIAN_POINT('',(-0.00501982557395217,0.0134,-0.0012));
#51543=CARTESIAN_POINT('Origin',(-0.00501982557395217,0.0134,-2.16840434497101E-19));
#51544=CARTESIAN_POINT('',(-0.00926982557395217,0.0134,-0.0025));
#51545=CARTESIAN_POINT('Origin',(-0.00926982557395217,0.0134,-0.003));
#51546=CARTESIAN_POINT('',(-0.00926982557395217,0.0134,0.0035));
#51547=CARTESIAN_POINT('Origin',(-0.00926982557395217,0.0134,0.003));
#51548=CARTESIAN_POINT('Origin',(-0.00501982557395217,-0.0233872477181734,
-2.16840434497101E-19));
#51549=CARTESIAN_POINT('',(-0.00386002285313196,0.0136,0.00221469132133082));
#51550=CARTESIAN_POINT('',(-0.00386002285313196,0.0148,0.00221469132133082));
#51551=CARTESIAN_POINT('',(-0.00386002285313196,-0.0233872477181734,0.00221469132133082));
#51552=CARTESIAN_POINT('',(-0.00386002285313196,0.0148,-0.00221469132133082));
#51553=CARTESIAN_POINT('Origin',(-0.00501982557395217,0.0148,-2.16840434497101E-19));
#51554=CARTESIAN_POINT('',(-0.00386002285313196,0.0136,-0.00221469132133082));
#51555=CARTESIAN_POINT('',(-0.00386002285313196,-0.0233872477181734,-0.00221469132133082));
#51556=CARTESIAN_POINT('Origin',(-0.00501982557395217,0.0136,-2.16840434497101E-19));
#51557=CARTESIAN_POINT('Origin',(-0.0170198255739522,-0.0233872477181734,
0.00910629506495907));
#51558=CARTESIAN_POINT('',(-0.016701694953409,0.0136,0.00893969452982874));
#51559=CARTESIAN_POINT('',(-0.016701694953409,0.0148,0.00893969452982874));
#51560=CARTESIAN_POINT('',(-0.016701694953409,-0.0233872477181734,0.00893969452982874));
#51561=CARTESIAN_POINT('',(-0.00386002285313196,0.0148,0.00221469132133081));
#51562=CARTESIAN_POINT('',(-0.0170198255739522,0.0136,0.00910629506495907));
#51563=CARTESIAN_POINT('Origin',(-0.0170198255739522,-0.0233872477181734,
-0.00910629506495906));
#51564=CARTESIAN_POINT('',(-0.016701694953409,0.0148,-0.00893969452982874));
#51565=CARTESIAN_POINT('',(-0.0170198255739522,0.0148,-0.00910629506495906));
#51566=CARTESIAN_POINT('',(-0.016701694953409,0.0136,-0.00893969452982874));
#51567=CARTESIAN_POINT('',(-0.016701694953409,-0.0233872477181734,-0.00893969452982874));
#51568=CARTESIAN_POINT('',(-0.0170198255739522,0.0136,-0.00910629506495906));
#51569=CARTESIAN_POINT('Ctrl Pts',(-0.0364455123647001,0.00340591076454288,
0.00292997690155913));
#51570=CARTESIAN_POINT('Ctrl Pts',(-0.0333747951719863,0.00232389768505854,
0.00146510792779752));
#51571=CARTESIAN_POINT('Ctrl Pts',(-0.030666089939513,3.24199491719774E-5,
0.00106768719154779));
#51572=CARTESIAN_POINT('Ctrl Pts',(-0.0362669964429192,0.00344366530354269,
0.00299137018949283));
#51573=CARTESIAN_POINT('Ctrl Pts',(-0.0331820842563904,0.00233996001538881,
0.00154459652507376));
#51574=CARTESIAN_POINT('Ctrl Pts',(-0.0304662723539453,3.26377421315948E-5,
0.0011853206571064));
#51575=CARTESIAN_POINT('Ctrl Pts',(-0.0359048356083394,0.00352223993193398,
0.00311624801154962));
#51576=CARTESIAN_POINT('Ctrl Pts',(-0.0327954167543044,0.00237267298125369,
0.00170402429165362));
#51577=CARTESIAN_POINT('Ctrl Pts',(-0.0300695591452557,3.30817301717868E-5,
0.00141885729043467));
#51578=CARTESIAN_POINT('Ctrl Pts',(-0.0353368818305699,0.00364968519670089,
0.00331160069857409));
#51579=CARTESIAN_POINT('Ctrl Pts',(-0.0322062130942011,0.00242275749036137,
0.00194751119469747));
#51580=CARTESIAN_POINT('Ctrl Pts',(-0.0294809352339733,3.37643438218347E-5,
0.00176534062295578));
#51581=CARTESIAN_POINT('Ctrl Pts',(-0.0347324273520965,0.00378725469799749,
0.00351789412330234));
#51582=CARTESIAN_POINT('Ctrl Pts',(-0.0316008826462354,0.00247324053409076,
0.0021994531946527));
#51583=CARTESIAN_POINT('Ctrl Pts',(-0.0288961484974036,3.44571825927306E-5,
0.00210954619418795));
#51584=CARTESIAN_POINT('Ctrl Pts',(-0.034185048803803,0.00391106611448223,
0.00370294412137096));
#51585=CARTESIAN_POINT('Ctrl Pts',(-0.0310754271943663,0.00251527669127259,
0.00242122290368142));
#51586=CARTESIAN_POINT('Ctrl Pts',(-0.0284093302761368,3.50404667023504E-5,
0.00239608347560846));
#51587=CARTESIAN_POINT('Ctrl Pts',(-0.0337092817698781,0.00401634422797446,
0.00386315824648985));
#51588=CARTESIAN_POINT('Ctrl Pts',(-0.0306359820359663,0.00254880604501725,
0.00261003824762744));
#51589=CARTESIAN_POINT('Ctrl Pts',(-0.0280183594648203,3.55115239250338E-5,
0.00262621551190547));
#51590=CARTESIAN_POINT('Ctrl Pts',(-0.0333296829265055,0.00409863588959051,
0.00399102434511768));
#51591=CARTESIAN_POINT('Ctrl Pts',(-0.0302949405967055,0.00257390378796406,
0.00275874528091764));
#51592=CARTESIAN_POINT('Ctrl Pts',(-0.0277240786605853,3.58677457098526E-5,
0.00279944354024005));
#51593=CARTESIAN_POINT('Ctrl Pts',(-0.0329218081184897,0.0041847120404232,
0.00412899533261083));
#51594=CARTESIAN_POINT('Ctrl Pts',(-0.0299393669415808,0.00259903849304822,
0.00291659451345235));
#51595=CARTESIAN_POINT('Ctrl Pts',(-0.0274278861496425,3.62288611593448E-5,
0.00297381181250567));
#51596=CARTESIAN_POINT('Ctrl Pts',(-0.0325522084676953,0.00426011777198721,
0.00425525216837874));
#51597=CARTESIAN_POINT('Ctrl Pts',(-0.0296275829358075,0.00262014249564209,
0.0030580312060908));
#51598=CARTESIAN_POINT('Ctrl Pts',(-0.0271786832862726,3.65364297070277E-5,
0.00312053589766483));
#51599=CARTESIAN_POINT('Ctrl Pts',(-0.0322332366460956,0.00432315291499516,
0.00436573860390773));
#51600=CARTESIAN_POINT('Ctrl Pts',(-0.0293659012756563,0.00263726882200995,
0.0031791299793348));
#51601=CARTESIAN_POINT('Ctrl Pts',(-0.0269772499404853,3.67891538465943E-5,
0.00323915086441261));
#51602=CARTESIAN_POINT('Ctrl Pts',(-0.0319804392227183,0.00437197070979676,
0.00445434196535493));
#51603=CARTESIAN_POINT('Ctrl Pts',(-0.0291625050568359,0.00265029366328149,
0.00327461785404188));
#51604=CARTESIAN_POINT('Ctrl Pts',(-0.02682493216657,3.69830684658742E-5,
0.00332885375602016));
#51605=CARTESIAN_POINT('Ctrl Pts',(-0.0317565244407999,0.00441413023968693,
0.00453399430810753));
#51606=CARTESIAN_POINT('Ctrl Pts',(-0.0289859845398002,0.0026613659398422,
0.00335880113672149));
#51607=CARTESIAN_POINT('Ctrl Pts',(-0.0266967639933256,3.71494125987322E-5,
0.00340434438765406));
#51608=CARTESIAN_POINT('Ctrl Pts',(-0.031567895438941,0.00444890207989184,
0.00460205596168863));
#51609=CARTESIAN_POINT('Ctrl Pts',(-0.0288397235658548,0.00267041177898812,
0.00342947624865893));
#51610=CARTESIAN_POINT('Ctrl Pts',(-0.0265933374933781,3.72862647502668E-5,
0.0034652694975214));
#51611=CARTESIAN_POINT('Ctrl Pts',(-0.0314211815457098,0.00447555725281909,
0.00465555130782646));
#51612=CARTESIAN_POINT('Ctrl Pts',(-0.0287272506203122,0.00267731062923309,
0.00348432164762575));
#51613=CARTESIAN_POINT('Ctrl Pts',(-0.0265152767808677,3.73911234432494E-5,
0.00351125648332721));
#51614=CARTESIAN_POINT('Ctrl Pts',(-0.0312686963284664,0.0045028342054351,
0.0047117935449501));
#51615=CARTESIAN_POINT('Ctrl Pts',(-0.0286117065954078,0.00268434106128931,
0.00354120125203931));
#51616=CARTESIAN_POINT('Ctrl Pts',(-0.0264366758557256,3.74984711339515E-5,
0.0035575661347842));
#51617=CARTESIAN_POINT('Ctrl Pts',(-0.0311096964982641,0.00453085160163887,
0.00477123004504529));
#51618=CARTESIAN_POINT('Ctrl Pts',(-0.0284926931804869,0.00269155560975046,
0.00360039129491648));
#51619=CARTESIAN_POINT('Ctrl Pts',(-0.0263574774216831,3.7609087124493E-5,
0.00360423290822119));
#51620=CARTESIAN_POINT('Ctrl Pts',(-0.0309713914373861,0.00455473602616356,
0.00482359862602796));
#51621=CARTESIAN_POINT('Ctrl Pts',(-0.0283904108244781,0.00269767648006451,
0.00365176307124788));
#51622=CARTESIAN_POINT('Ctrl Pts',(-0.0262909288458718,3.77033890942823E-5,
0.00364345014849943));
#51623=CARTESIAN_POINT('Ctrl Pts',(-0.0308561825197073,0.00457455485418223,
0.0048679434459117));
#51624=CARTESIAN_POINT('Ctrl Pts',(-0.0283061545418152,0.00270282781575326,
0.0036945215769936));
#51625=CARTESIAN_POINT('Ctrl Pts',(-0.0262373176226958,3.77828009240422E-5,
0.00367504736385796));
#51626=CARTESIAN_POINT('Ctrl Pts',(-0.030783451543195,0.00458653413502901,
0.00489576854994378));
#51627=CARTESIAN_POINT('Ctrl Pts',(-0.0282530896816562,0.00270580485141099,
0.00372142305380727));
#51628=CARTESIAN_POINT('Ctrl Pts',(-0.0262036563470202,3.78291696305176E-5,
0.00369488599018227));
#51629=CARTESIAN_POINT('Ctrl Pts',(-0.0307293296760956,0.0045962451598897,
0.0049174436794188));
#51630=CARTESIAN_POINT('Ctrl Pts',(-0.0282142654926756,0.00270852223581756,
0.00374156046938465));
#51631=CARTESIAN_POINT('Ctrl Pts',(-0.0261799863912769,3.78706614478648E-5,
0.00370884079396693));
#51632=CARTESIAN_POINT('Ctrl Pts',(-0.0307015264051103,0.00459992790810007,
0.00492738598974962));
#51633=CARTESIAN_POINT('Ctrl Pts',(-0.0281936909151507,0.00270914622671935,
0.00375170204460587));
#51634=CARTESIAN_POINT('Ctrl Pts',(-0.0261664601757535,3.78812763338712E-5,
0.00371680943126161));
#51635=CARTESIAN_POINT('Ctrl Pts',(-0.0306759785647499,0.00460670317667091,
0.00493977799715337));
#51636=CARTESIAN_POINT('Ctrl Pts',(-0.0281766044250891,0.002711744575781,
0.00376154458782346));
#51637=CARTESIAN_POINT('Ctrl Pts',(-0.0261579338285578,3.79191187909183E-5,
0.00372184690489322));
#51638=CARTESIAN_POINT('Ctrl Pts',(-0.0306739081276985,0.00460190391753511,
0.00493571878828618));
#51639=CARTESIAN_POINT('Ctrl Pts',(-0.0281724315802146,0.00270877101912153,
0.0037615151616685));
#51640=CARTESIAN_POINT('Ctrl Pts',(-0.0261512462899574,3.78780240191974E-5,
0.00372576551137767));
#51641=CARTESIAN_POINT('Ctrl Pts',(-0.0305817008950556,0.00464718206751526,
0.00500013630428141));
#51642=CARTESIAN_POINT('Ctrl Pts',(-0.028121665557071,0.00273053660259818,
0.00380025138698242));
#51643=CARTESIAN_POINT('Ctrl Pts',(-0.0261438777031298,3.81864845659119E-5,
0.00373024570056496));
#51644=CARTESIAN_POINT('Ctrl Pts',(-0.0304512352465178,0.00470705887529274,
0.00508932502427095));
#51645=CARTESIAN_POINT('Ctrl Pts',(-0.0280486526672015,0.00275918545777291,
0.00385443627071402));
#51646=CARTESIAN_POINT('Ctrl Pts',(-0.0261310958420302,3.8592713764993E-5,
0.0037379588375763));
#51647=CARTESIAN_POINT('Ctrl Pts',(-0.0302097657705172,0.00481654509266694,
0.00525862778588942));
#51648=CARTESIAN_POINT('Ctrl Pts',(-0.0279154643696936,0.00281236805077608,
0.00395458858415277));
#51649=CARTESIAN_POINT('Ctrl Pts',(-0.0261121862462621,3.93455240931729E-5,
0.0037494416009322));
#51650=CARTESIAN_POINT('Ctrl Pts',(-0.0298456573331352,0.0049707839105292,
0.00552107347107061));
#51651=CARTESIAN_POINT('Ctrl Pts',(-0.0277156005697513,0.00288931259523331,
0.0041046739806172));
#51652=CARTESIAN_POINT('Ctrl Pts',(-0.0260883721232669,4.04305341557616E-5,
0.00376397058687835));
#51653=CARTESIAN_POINT('Ctrl Pts',(-0.029294757673212,0.00518712242800417,
0.00593483822630104));
#51654=CARTESIAN_POINT('Ctrl Pts',(-0.0274151742246471,0.00300185665309095,
0.00433081235633842));
#51655=CARTESIAN_POINT('Ctrl Pts',(-0.0260624466832064,4.20073033700595E-5,
0.00377997647220182));
#51656=CARTESIAN_POINT('Ctrl Pts',(-0.0285524571140508,0.0054366086587878,
0.00654380090261184));
#51657=CARTESIAN_POINT('Ctrl Pts',(-0.027001949242104,0.00314768404954061,
0.00463992614113889));
#51658=CARTESIAN_POINT('Ctrl Pts',(-0.0260335236074697,4.401142030668E-5,
0.00379796151968866));
#51659=CARTESIAN_POINT('Ctrl Pts',(-0.0280809156183133,0.00556967658510273,
0.00696339051093119));
#51660=CARTESIAN_POINT('Ctrl Pts',(-0.0267268473930116,0.00323774605000878,
0.00484327138018103));
#51661=CARTESIAN_POINT('Ctrl Pts',(-0.0260064442295,4.52205599225896E-5,
0.00381451140871031));
#51662=CARTESIAN_POINT('Ctrl Pts',(-0.0277524351262434,0.00565354262612152,
0.00726569554266335));
#51663=CARTESIAN_POINT('Ctrl Pts',(-0.0265287908709839,0.0032993317982997,
0.00498871081272797));
#51664=CARTESIAN_POINT('Ctrl Pts',(-0.0259804809093425,4.60369483617543E-5,
0.00383023176033879));
#51665=CARTESIAN_POINT('Ctrl Pts',(-0.0274161511476627,0.00573049620110287,
0.00758476525177793));
#51666=CARTESIAN_POINT('Ctrl Pts',(-0.0263196182699441,0.00336105701133233,
0.00514148687082381));
#51667=CARTESIAN_POINT('Ctrl Pts',(-0.025946633572234,4.68447015644706E-5,
0.00385061772352051));
#51668=CARTESIAN_POINT('Ctrl Pts',(-0.027107213168873,0.00579088786390267,
0.00788764517379605));
#51669=CARTESIAN_POINT('Ctrl Pts',(-0.0261194595041263,0.00341582373363926,
0.00528685403998759));
#51670=CARTESIAN_POINT('Ctrl Pts',(-0.0259051879585585,4.75500473328697E-5,
0.00387546346390592));
#51671=CARTESIAN_POINT('Ctrl Pts',(-0.0268222191277561,0.00583771371380135,
0.00817407869531208));
#51672=CARTESIAN_POINT('Ctrl Pts',(-0.0259277666571967,0.00346424929736276,
0.00542562025819949));
#51673=CARTESIAN_POINT('Ctrl Pts',(-0.0258569234762942,4.8164363075934E-5,
0.00390431639822479));
#51674=CARTESIAN_POINT('Ctrl Pts',(-0.0265096649800296,0.00588051745048727,
0.00849409109638237));
#51675=CARTESIAN_POINT('Ctrl Pts',(-0.0257106286229303,0.00351508733799058,
0.00558256061587452));
#51676=CARTESIAN_POINT('Ctrl Pts',(-0.0257937198450575,4.88001461067806E-5,
0.00394203740391715));
#51677=CARTESIAN_POINT('Ctrl Pts',(-0.0261995682192878,0.00591132484202696,
0.00881840166566976));
#51678=CARTESIAN_POINT('Ctrl Pts',(-0.0254860437689506,0.00356200174806162,
0.00574482934744544));
#51679=CARTESIAN_POINT('Ctrl Pts',(-0.0257163416563158,4.93751853691084E-5,
0.00398814680952696));
#51680=CARTESIAN_POINT('Ctrl Pts',(-0.0257938698545106,0.00593627093979265,
0.00924940881465935));
#51681=CARTESIAN_POINT('Ctrl Pts',(-0.0251803962446941,0.0036180473812791,
0.00596617519969835));
#51682=CARTESIAN_POINT('Ctrl Pts',(-0.0255947569082474,5.00467832057705E-5,
0.00406052623970451));
#51683=CARTESIAN_POINT('Ctrl Pts',(-0.0253923226440449,0.00593971548210584,
0.00968302452453125));
#51684=CARTESIAN_POINT('Ctrl Pts',(-0.0248623974297738,0.00366536133344948,
0.00619779346020047));
#51685=CARTESIAN_POINT('Ctrl Pts',(-0.0254454981240691,5.05928833255763E-5,
0.00414930233341545));
#51686=CARTESIAN_POINT('Ctrl Pts',(-0.0249986734962245,0.00592312729945216,
0.0101112731277479));
#51687=CARTESIAN_POINT('Ctrl Pts',(-0.0245372400514592,0.00370302273718345,
0.00643685192505727));
#51688=CARTESIAN_POINT('Ctrl Pts',(-0.0252710108219186,5.10068228760653E-5,
0.00425303531907116));
#51689=CARTESIAN_POINT('Ctrl Pts',(-0.0246605209153862,0.00589409094509935,
0.0104799528591913));
#51690=CARTESIAN_POINT('Ctrl Pts',(-0.0242485447068516,0.00372845658143586,
0.00665116676847146));
#51691=CARTESIAN_POINT('Ctrl Pts',(-0.0250999117617437,5.1268439305896E-5,
0.00435472885127864));
#51692=CARTESIAN_POINT('Ctrl Pts',(-0.0243597776620712,0.00585707152211605,
0.0108072836977489));
#51693=CARTESIAN_POINT('Ctrl Pts',(-0.0239851571629279,0.00374548999173081,
0.0068485555891743));
#51694=CARTESIAN_POINT('Ctrl Pts',(-0.0249313947513967,5.14269322207653E-5,
0.00445487455205838));
#51695=CARTESIAN_POINT('Ctrl Pts',(-0.0239953492978759,0.0058002555009245,
0.0112023189097569));
#51696=CARTESIAN_POINT('Ctrl Pts',(-0.023659184141879,0.00375987256159987,
0.00709506282792327));
#51697=CARTESIAN_POINT('Ctrl Pts',(-0.0247094746225135,5.15372030271051E-5,
0.00458674636673381));
#51698=CARTESIAN_POINT('Ctrl Pts',(-0.0235913514326662,0.00571925070838247,
0.0116362329642894));
#51699=CARTESIAN_POINT('Ctrl Pts',(-0.0232884818635941,0.00376590220862389,
0.00737905762402919));
#51700=CARTESIAN_POINT('Ctrl Pts',(-0.0244363149918091,5.15321333879219E-5,
0.00474905568053847));
#51701=CARTESIAN_POINT('Ctrl Pts',(-0.023158991970489,0.0056129492390785,
0.0120931021922947));
#51702=CARTESIAN_POINT('Ctrl Pts',(-0.0228826498218856,0.00376066312518332,
0.0076944351282338));
#51703=CARTESIAN_POINT('Ctrl Pts',(-0.0241133983629133,5.13796891134259E-5,
0.00494092386423699));
#51704=CARTESIAN_POINT('Ctrl Pts',(-0.0226319129215638,0.00546354818217184,
0.012639550107198));
#51705=CARTESIAN_POINT('Ctrl Pts',(-0.0223791154247985,0.00374157039263029,
0.00809045414576035));
#51706=CARTESIAN_POINT('Ctrl Pts',(-0.0236876437050478,5.10365477415924E-5,
0.00519388996668408));
#51707=CARTESIAN_POINT('Ctrl Pts',(-0.0220427484603341,0.00526875827317497,
0.0132307259340806));
#51708=CARTESIAN_POINT('Ctrl Pts',(-0.0218054301955835,0.00370089266382102,
0.00854835534568239));
#51709=CARTESIAN_POINT('Ctrl Pts',(-0.0231644666249741,5.04164249423466E-5,
0.00550472954656049));
#51710=CARTESIAN_POINT('Ctrl Pts',(-0.0214022105896984,0.00503087002550459,
0.0138443682153251));
#51711=CARTESIAN_POINT('Ctrl Pts',(-0.0211724262978549,0.00363502645902371,
0.00905918822391987));
#51712=CARTESIAN_POINT('Ctrl Pts',(-0.0225455170232091,4.94807903072516E-5,
0.00587244025833354));
#51713=CARTESIAN_POINT('Ctrl Pts',(-0.0206076112485532,0.0047135341608338,
0.014569016759525));
#51714=CARTESIAN_POINT('Ctrl Pts',(-0.0203790291879768,0.00353078858065994,
0.00970228983916538));
#51715=CARTESIAN_POINT('Ctrl Pts',(-0.0217277835251736,4.80490545205933E-5,
0.00635818294222504));
#51716=CARTESIAN_POINT('Ctrl Pts',(-0.0200569456108525,0.00447901500725725,
0.01503294755748));
#51717=CARTESIAN_POINT('Ctrl Pts',(-0.01982337570409,0.00343879995533105,
0.0101515640080081));
#51718=CARTESIAN_POINT('Ctrl Pts',(-0.0211192082891102,4.68180167576593E-5,
0.00671958904311641));
#51719=CARTESIAN_POINT('Ctrl Pts',(-0.0196993664659313,0.00432573469918011,
0.0153197074216856));
#51720=CARTESIAN_POINT('Ctrl Pts',(-0.0194607362281236,0.00337353450158482,
0.0104416089908505));
#51721=CARTESIAN_POINT('Ctrl Pts',(-0.0207133290522096,4.59510186099511E-5,
0.00696056413499288));
#51722=CARTESIAN_POINT('',(-0.0307219745744663,7.95258423531978E-5,0.00107599969506516));
#51723=CARTESIAN_POINT('Origin',(-0.0367510524517764,-0.00895601651477296,
0.0114205245397328));
#51724=CARTESIAN_POINT('',(-0.0262191092076098,0.00012427284417193,0.0037259611256264));
#51725=CARTESIAN_POINT('Ctrl Pts',(-0.0307219740115217,7.95260984898368E-5,
0.00107600024689227));
#51726=CARTESIAN_POINT('Ctrl Pts',(-0.0305252572528752,8.13345891118369E-5,
0.00119223192931586));
#51727=CARTESIAN_POINT('Ctrl Pts',(-0.0303284251623317,8.32609267468997E-5,
0.00130852983035956));
#51728=CARTESIAN_POINT('Ctrl Pts',(-0.0301316153384272,8.52758354696813E-5,
0.00142477868099659));
#51729=CARTESIAN_POINT('Ctrl Pts',(-0.0299369158857927,8.72691385358141E-5,
0.00153978100730014));
#51730=CARTESIAN_POINT('Ctrl Pts',(-0.0297422370116984,8.93491181379123E-5,
0.00165473599950342));
#51731=CARTESIAN_POINT('Ctrl Pts',(-0.0295476067310188,9.14849303570787E-5,
0.00176960141917011));
#51732=CARTESIAN_POINT('Ctrl Pts',(-0.0293540301943859,9.36091791165256E-5,
0.00188384494818485));
#51733=CARTESIAN_POINT('Ctrl Pts',(-0.0291605002719552,9.57886356598487E-5,
0.00199800069131126));
#51734=CARTESIAN_POINT('Ctrl Pts',(-0.028966900823677,9.79911655836168E-5,
0.00211212007243703));
#51735=CARTESIAN_POINT('Ctrl Pts',(-0.0288820222035214,9.895680728582E-5,
0.00216215273363064));
#51736=CARTESIAN_POINT('Ctrl Pts',(-0.028797129948477,9.99268420874477E-5,
0.00221217864547998));
#51737=CARTESIAN_POINT('Ctrl Pts',(-0.0287122065938775,0.00010089857280184,
0.0022622074254998));
#51738=CARTESIAN_POINT('Ctrl Pts',(-0.0286036039689568,0.000102141252236687,
0.00232618578407208));
#51739=CARTESIAN_POINT('Ctrl Pts',(-0.0284947741845346,0.000103390112473951,
0.0023902735069483));
#51740=CARTESIAN_POINT('Ctrl Pts',(-0.0283858420771839,0.000104631353219126,
0.00245439234151685));
#51741=CARTESIAN_POINT('Ctrl Pts',(-0.028288569628719,0.000105739736498895,
0.00251164815142346));
#51742=CARTESIAN_POINT('Ctrl Pts',(-0.0281912154713187,0.000106842034320342,
0.00256892885933081));
#51743=CARTESIAN_POINT('Ctrl Pts',(-0.0280938961439213,0.000107928199043347,
0.00262616431261735));
#51744=CARTESIAN_POINT('Ctrl Pts',(-0.0279959851842882,0.000109020966874701,
0.00268374771671787));
#51745=CARTESIAN_POINT('Ctrl Pts',(-0.0278981088942278,0.000110097405311395,
0.00274128566927246));
#51746=CARTESIAN_POINT('Ctrl Pts',(-0.027800296460405,0.000111147477837171,
0.00279876033041972));
#51747=CARTESIAN_POINT('Ctrl Pts',(-0.0277014984804252,0.000112208130765682,
0.00285681409924481));
#51748=CARTESIAN_POINT('Ctrl Pts',(-0.0276027651039974,0.000113241889062903,
0.00291480362867732));
#51749=CARTESIAN_POINT('Ctrl Pts',(-0.0275041250658499,0.000114238488510968,
0.0029727129547738));
#51750=CARTESIAN_POINT('Ctrl Pts',(-0.0274040669501753,0.000115249415359015,
0.00303145480197922));
#51751=CARTESIAN_POINT('Ctrl Pts',(-0.0273041037905599,0.000116222120639044,
0.00309011478667495));
#51752=CARTESIAN_POINT('Ctrl Pts',(-0.0272042255891732,0.000117146481370503,
0.00314870161633757));
#51753=CARTESIAN_POINT('Ctrl Pts',(-0.0271536039826784,0.000117614978245272,
0.00317839537729622));
#51754=CARTESIAN_POINT('Ctrl Pts',(-0.0271030047169357,0.000118071045377641,
0.0032080700472859));
#51755=CARTESIAN_POINT('Ctrl Pts',(-0.0270524214565589,0.00011851347969458,
0.00323772994986223));
#51756=CARTESIAN_POINT('Ctrl Pts',(-0.0270012925077992,0.000118960686959428,
0.00326770982122177));
#51757=CARTESIAN_POINT('Ctrl Pts',(-0.0269501798413928,0.000119393967140987,
0.00329767464809863));
#51758=CARTESIAN_POINT('Ctrl Pts',(-0.0268990741911264,0.000119812157868954,
0.00332763063128599));
#51759=CARTESIAN_POINT('Ctrl Pts',(-0.0268473465297388,0.000120235438431063,
0.00335795121123693));
#51760=CARTESIAN_POINT('Ctrl Pts',(-0.0267956259413342,0.000120643262574798,
0.00338826280173099));
#51761=CARTESIAN_POINT('Ctrl Pts',(-0.0267438961144647,0.000121034609501203,
0.00341857601094203));
#51762=CARTESIAN_POINT('Ctrl Pts',(-0.0267177717553492,0.000121232245725077,
0.00343388464836257));
#51763=CARTESIAN_POINT('Ctrl Pts',(-0.0266916451290816,0.000121425677806561,
0.00344919364504706));
#51764=CARTESIAN_POINT('Ctrl Pts',(-0.026665513235662,0.000121614815219698,
0.0034645049316798));
#51765=CARTESIAN_POINT('Ctrl Pts',(-0.0266391931547748,0.000121805314696052,
0.00347992648174471));
#51766=CARTESIAN_POINT('Ctrl Pts',(-0.0266128677255237,0.000121991457392134,
0.00349535035792513));
#51767=CARTESIAN_POINT('Ctrl Pts',(-0.0265865335877925,0.000122173105607934,
0.00351077869403059));
#51768=CARTESIAN_POINT('Ctrl Pts',(-0.0265599989071751,0.000122356137133028,
0.00352632452185281));
#51769=CARTESIAN_POINT('Ctrl Pts',(-0.0265334553754045,0.000122534606498225,
0.00354187488399971));
#51770=CARTESIAN_POINT('Ctrl Pts',(-0.0265068982539826,0.000122708637195116,
0.00355743286379766));
#51771=CARTESIAN_POINT('Ctrl Pts',(-0.0264801273676615,0.000122884068708525,
0.00357311607365837));
#51772=CARTESIAN_POINT('Ctrl Pts',(-0.0264533426686387,0.000123054986866343,
0.00358880702510529));
#51773=CARTESIAN_POINT('Ctrl Pts',(-0.0264265400040283,0.000123220680241195,
0.00360450809544571));
#51774=CARTESIAN_POINT('Ctrl Pts',(-0.0264151459496129,0.000123291117988962,
0.00361118276202975));
#51775=CARTESIAN_POINT('Ctrl Pts',(-0.0264037486565156,0.000123360612090243,
0.00361785925271107));
#51776=CARTESIAN_POINT('Ctrl Pts',(-0.0263923472133218,0.000123429359989684,
0.00362453821571575));
#51777=CARTESIAN_POINT('Ctrl Pts',(-0.0263767145458341,0.000123523621131379,
0.00363369582901427));
#51778=CARTESIAN_POINT('Ctrl Pts',(-0.0263610595312741,0.000123628241621857,
0.00364287217015774));
#51779=CARTESIAN_POINT('Ctrl Pts',(-0.0263454005924302,0.000123732914342874,
0.0036520516001013));
#51780=CARTESIAN_POINT('Ctrl Pts',(-0.0263317686235584,0.000123824037712654,
0.00366004279953693));
#51781=CARTESIAN_POINT('Ctrl Pts',(-0.0263181337153121,0.000123915187696385,
0.00366803631562752));
#51782=CARTESIAN_POINT('Ctrl Pts',(-0.0263045153126929,0.000123995921902339,
0.00367601595328584));
#51783=CARTESIAN_POINT('Ctrl Pts',(-0.0262907854281113,0.000124077317008691,
0.00368406091326504));
#51784=CARTESIAN_POINT('Ctrl Pts',(-0.0262770721649393,0.000124148203574728,
0.0036920918942593));
#51785=CARTESIAN_POINT('Ctrl Pts',(-0.0262633646773175,0.000124214468613312,
0.00370011806415441));
#51786=CARTESIAN_POINT('Ctrl Pts',(-0.0262564551243315,0.000124247870926547,
0.00370416382714869));
#51787=CARTESIAN_POINT('Ctrl Pts',(-0.026249547190954,0.000124280025057016,
0.00370820824545637));
#51788=CARTESIAN_POINT('Ctrl Pts',(-0.0262426750462274,0.0001242928932531,
0.00371222298187236));
#51789=CARTESIAN_POINT('Ctrl Pts',(-0.0262376653489532,0.00012430227398785,
0.00371514966850082));
#51790=CARTESIAN_POINT('Ctrl Pts',(-0.0262326274393708,0.000124326403532759,
0.00371809980664705));
#51791=CARTESIAN_POINT('Ctrl Pts',(-0.0262275856449859,0.000124352433508816,
0.00372105321361447));
#51792=CARTESIAN_POINT('Ctrl Pts',(-0.026224665565161,0.000124367509412776,
0.00372276375225252));
#51793=CARTESIAN_POINT('Ctrl Pts',(-0.0262220357872776,0.000124236843468986,
0.00372423694144539));
#51794=CARTESIAN_POINT('Ctrl Pts',(-0.0262191092076098,0.00012427284417193,
0.0037259611256264));
#51795=CARTESIAN_POINT('',(-0.0207569920523634,8.45301690043879E-5,0.0069665043144839));
#51796=CARTESIAN_POINT('Ctrl Pts',(-0.0262191092076098,0.00012427284417193,
0.0037259611256264));
#51797=CARTESIAN_POINT('Ctrl Pts',(-0.026218313252602,0.000124257642349168,
0.00372641839465707));
#51798=CARTESIAN_POINT('Ctrl Pts',(-0.0262174583909347,0.000124274509407832,
0.00372692500192157));
#51799=CARTESIAN_POINT('Ctrl Pts',(-0.0262165687577017,0.000124310605772055,
0.00372746087457822));
#51800=CARTESIAN_POINT('Ctrl Pts',(-0.0262104887075549,0.000124557300360844,
0.00373112320699108));
#51801=CARTESIAN_POINT('Ctrl Pts',(-0.026203466830604,0.000125314347699211,
0.00373557411719657));
#51802=CARTESIAN_POINT('Ctrl Pts',(-0.0261971149797945,0.000125703392451664,
0.00373946416591847));
#51803=CARTESIAN_POINT('Ctrl Pts',(-0.0261877584649919,0.000126276469983611,
0.00374519435378668));
#51804=CARTESIAN_POINT('Ctrl Pts',(-0.0261784184200931,0.000126837975953154,
0.00375091282474766));
#51805=CARTESIAN_POINT('Ctrl Pts',(-0.0261691966518907,0.00012731559893701,
0.00375652714292099));
#51806=CARTESIAN_POINT('Ctrl Pts',(-0.0261588155943136,0.000127853264988325,
0.00376284724975233));
#51807=CARTESIAN_POINT('Ctrl Pts',(-0.0261485536193207,0.00012829898441606,
0.00376906010303047));
#51808=CARTESIAN_POINT('Ctrl Pts',(-0.0261380673911856,0.000128789974380921,
0.00377543129488929));
#51809=CARTESIAN_POINT('Ctrl Pts',(-0.0261262956103143,0.000129341156960766,
0.00378258355912431));
#51810=CARTESIAN_POINT('Ctrl Pts',(-0.0261142716574951,0.000129932778179259,
0.00378991014955548));
#51811=CARTESIAN_POINT('Ctrl Pts',(-0.0261019504193946,0.000130510114165908,
0.00379741689306796));
#51812=CARTESIAN_POINT('Ctrl Pts',(-0.0260883874996105,0.000131145631604298,
0.00380568013408884));
#51813=CARTESIAN_POINT('Ctrl Pts',(-0.0260745686731552,0.0001317384880603,
0.00381408777172032));
#51814=CARTESIAN_POINT('Ctrl Pts',(-0.0260621770610233,0.000131810391501782,
0.0038214233342845));
#51815=CARTESIAN_POINT('Ctrl Pts',(-0.026049122476854,0.00013188614189801,
0.00382915136175217));
#51816=CARTESIAN_POINT('Ctrl Pts',(-0.0260375247560911,0.000131425149614633,
0.00383578351186937));
#51817=CARTESIAN_POINT('Ctrl Pts',(-0.0260264852753561,0.000130800874521038,
0.00384201505075769));
#51818=CARTESIAN_POINT('Ctrl Pts',(-0.0260155572388606,0.000130182901523054,
0.00384818368187621));
#51819=CARTESIAN_POINT('Ctrl Pts',(-0.0260051922966206,0.000129397723389961,
0.00385394717785739));
#51820=CARTESIAN_POINT('Ctrl Pts',(-0.0259948301686768,0.000128635554659348,
0.00385972339426267));
#51821=CARTESIAN_POINT('Ctrl Pts',(-0.0259851541880192,0.000127923854327597,
0.00386511712791609));
#51822=CARTESIAN_POINT('Ctrl Pts',(-0.0259754844107568,0.00012723076004095,
0.00387051909059551));
#51823=CARTESIAN_POINT('Ctrl Pts',(-0.0259655001182173,0.000126665520066985,
0.00387616921576119));
#51824=CARTESIAN_POINT('Ctrl Pts',(-0.0259504486967768,0.00012581341512019,
0.00388468683628603));
#51825=CARTESIAN_POINT('Ctrl Pts',(-0.0259346753191958,0.000125251151555231,
0.00389377221539224));
#51826=CARTESIAN_POINT('Ctrl Pts',(-0.0259174185138597,0.000125266953211752,
0.00390401171199071));
#51827=CARTESIAN_POINT('Ctrl Pts',(-0.0258978752943211,0.000125284848484745,
0.0039156078751328));
#51828=CARTESIAN_POINT('Ctrl Pts',(-0.025878398121216,0.000125281820980013,
0.00392716302802724));
#51829=CARTESIAN_POINT('Ctrl Pts',(-0.0258588900120178,0.000125282028506469,
0.00393874416856717));
#51830=CARTESIAN_POINT('Ctrl Pts',(-0.0258422233954665,0.000125282205805246,
0.00394863843492812));
#51831=CARTESIAN_POINT('Ctrl Pts',(-0.0258255312581991,0.000125284518560359,
0.00395855330740935));
#51832=CARTESIAN_POINT('Ctrl Pts',(-0.0258088207793041,0.000125289424603215,
0.00396848398787762));
#51833=CARTESIAN_POINT('Ctrl Pts',(-0.0257840514799041,0.000125296696641624,
0.00398320385313759));
#51834=CARTESIAN_POINT('Ctrl Pts',(-0.0257592419786764,0.000125309797834037,
0.00399795849075353));
#51835=CARTESIAN_POINT('Ctrl Pts',(-0.0257345055512984,0.000125296226632468,
0.00401266387494284));
#51836=CARTESIAN_POINT('Ctrl Pts',(-0.0257269516828363,0.000125292082336691,
0.00401715452091017));
#51837=CARTESIAN_POINT('Ctrl Pts',(-0.025719414317235,0.000125283071607205,
0.00402163368790882));
#51838=CARTESIAN_POINT('Ctrl Pts',(-0.0257118899152836,0.000125270118788965,
0.00402610384659461));
#51839=CARTESIAN_POINT('Ctrl Pts',(-0.0256803268705193,0.000125215784851918,
0.00404485508019595));
#51840=CARTESIAN_POINT('Ctrl Pts',(-0.0256489924869321,0.000125092034389544,
0.00406344745792039));
#51841=CARTESIAN_POINT('Ctrl Pts',(-0.0256177491731015,0.000124927750833351,
0.00408197378525708));
#51842=CARTESIAN_POINT('Ctrl Pts',(-0.0255564195001067,0.000124605267218635,
0.00411834040127974));
#51843=CARTESIAN_POINT('Ctrl Pts',(-0.0254954377548005,0.000124126490117409,
0.0041544542529373));
#51844=CARTESIAN_POINT('Ctrl Pts',(-0.0254347581974083,0.000123584215385121,
0.00419037491538026));
#51845=CARTESIAN_POINT('Ctrl Pts',(-0.0253754594351541,0.000123054280398638,
0.00422547818431893));
#51846=CARTESIAN_POINT('Ctrl Pts',(-0.0253164521623267,0.000122463921329405,
0.00426039531471784));
#51847=CARTESIAN_POINT('Ctrl Pts',(-0.0252575344012696,0.000121847452620448,
0.00429525749972636));
#51848=CARTESIAN_POINT('Ctrl Pts',(-0.0251998379772801,0.000121243763013611,
0.00432939700827802));
#51849=CARTESIAN_POINT('Ctrl Pts',(-0.0251422265861802,0.000120615089204082,
0.00436348431978858));
#51850=CARTESIAN_POINT('Ctrl Pts',(-0.0250845856810912,0.00011997913229085,
0.00439759301155981));
#51851=CARTESIAN_POINT('Ctrl Pts',(-0.0250280357281178,0.000119355211943296,
0.00443105613835619));
#51852=CARTESIAN_POINT('Ctrl Pts',(-0.0249714568511407,0.000118724306895247,
0.00446454015753084));
#51853=CARTESIAN_POINT('Ctrl Pts',(-0.0249147917049414,0.000118095225489086,
0.0044980816054591));
#51854=CARTESIAN_POINT('Ctrl Pts',(-0.0248591073634841,0.000117477032716725,
0.00453104249173021));
#51855=CARTESIAN_POINT('Ctrl Pts',(-0.0248033395066288,0.000116860609546021,
0.0045640589607905));
#51856=CARTESIAN_POINT('Ctrl Pts',(-0.0247474512262175,0.000116251253002794,
0.00459715428310829));
#51857=CARTESIAN_POINT('Ctrl Pts',(-0.0246382440577773,0.000115060554305916,
0.00466182341252776));
#51858=CARTESIAN_POINT('Ctrl Pts',(-0.0245285801009226,0.000113896810116591,
0.0047267918768944));
#51859=CARTESIAN_POINT('Ctrl Pts',(-0.0244183518607806,0.000112776485805999,
0.00479212631922648));
#51860=CARTESIAN_POINT('Ctrl Pts',(-0.0243110402029364,0.000111685804697981,
0.00485573204596173));
#51861=CARTESIAN_POINT('Ctrl Pts',(-0.0242031919125816,0.000110636321447355,
0.00491968572852661));
#51862=CARTESIAN_POINT('Ctrl Pts',(-0.0240947885822766,0.000109629476930135,
0.00498399669551821));
#51863=CARTESIAN_POINT('Ctrl Pts',(-0.0239887863865853,0.000108644934026843,
0.00504688317408824));
#51864=CARTESIAN_POINT('Ctrl Pts',(-0.0238822510031491,0.000107701166320274,
0.00511011274960858));
#51865=CARTESIAN_POINT('Ctrl Pts',(-0.0237753609545318,0.000106795374651794,
0.00517357556253613));
#51866=CARTESIAN_POINT('Ctrl Pts',(-0.0235670917864745,0.00010503049120691,
0.00529722923677397));
#51867=CARTESIAN_POINT('Ctrl Pts',(-0.0233574948382918,0.000103409482345986,
0.00542175804479225));
#51868=CARTESIAN_POINT('Ctrl Pts',(-0.0231469207294679,0.00010187771712088,
0.00554691553928123));
#51869=CARTESIAN_POINT('Ctrl Pts',(-0.0229414037745486,0.000100382738813845,
0.00566906724775274));
#51870=CARTESIAN_POINT('Ctrl Pts',(-0.0227349470379256,9.89726889956665E-5,
0.0057918231121365));
#51871=CARTESIAN_POINT('Ctrl Pts',(-0.0225281333326472,9.75825445919448E-5,
0.00591478789175411));
#51872=CARTESIAN_POINT('Ctrl Pts',(-0.02232403982328,9.6210684591173E-5,
0.00603613533034356));
#51873=CARTESIAN_POINT('Ctrl Pts',(-0.0221195951197529,9.48581312153604E-5,
0.00615768826359034));
#51874=CARTESIAN_POINT('Ctrl Pts',(-0.0219154123534245,9.34628299006657E-5,
0.00627902490392014));
#51875=CARTESIAN_POINT('Ctrl Pts',(-0.0215266328754144,9.08060703388838E-5,
0.00651005907266608));
#51876=CARTESIAN_POINT('Ctrl Pts',(-0.021138800462131,8.79873584830102E-5,
0.00674031620404643));
#51877=CARTESIAN_POINT('Ctrl Pts',(-0.0207569064093787,8.46249031451449E-5,
0.00696634980021813));
#51878=CARTESIAN_POINT('Ctrl Pts',(-0.0207569920523634,8.45301690043879E-5,
0.0069665043144839));
#51879=CARTESIAN_POINT('Ctrl Pts',(-0.0210089319175918,0.000156447471720346,
0.00687493731751199));
#51880=CARTESIAN_POINT('Ctrl Pts',(-0.0212588640564334,0.000233847770492934,
0.00678509563754937));
#51881=CARTESIAN_POINT('Ctrl Pts',(-0.0215066257862298,0.000317179867387291,
0.00669685818551664));
#51882=CARTESIAN_POINT('Ctrl Pts',(-0.0217186243241269,0.000388483384342961,
0.00662135737740526));
#51883=CARTESIAN_POINT('Ctrl Pts',(-0.0219289662434665,0.000464028822881538,
0.00654699979756583));
#51884=CARTESIAN_POINT('Ctrl Pts',(-0.0221376399317455,0.000544631803685119,
0.00647399888350404));
#51885=CARTESIAN_POINT('Ctrl Pts',(-0.0222947802331561,0.000605329330060039,
0.00641902604177432));
#51886=CARTESIAN_POINT('Ctrl Pts',(-0.0224509733069686,0.000668898321367291,
0.0063648219031823));
#51887=CARTESIAN_POINT('Ctrl Pts',(-0.0226062016136997,0.00073503623390973,
0.00631153256380226));
#51888=CARTESIAN_POINT('Ctrl Pts',(-0.0229675645848045,0.000889001661236195,
0.00618747790900306));
#51889=CARTESIAN_POINT('Ctrl Pts',(-0.0233240023418203,0.0010564663025375,
0.00606787748581256));
#51890=CARTESIAN_POINT('Ctrl Pts',(-0.023677835969773,0.0012347319140267,
0.00595343570009491));
#51891=CARTESIAN_POINT('Ctrl Pts',(-0.023951102370562,0.00137240679337031,
0.00586505208584131));
#51892=CARTESIAN_POINT('Ctrl Pts',(-0.0242233983168268,0.0015188332599898,
0.00578093151035615));
#51893=CARTESIAN_POINT('Ctrl Pts',(-0.0244935184573884,0.00166964263063737,
0.00570110719725304));
#51894=CARTESIAN_POINT('Ctrl Pts',(-0.024689744656477,0.00177919665918037,
0.00564311958654575));
#51895=CARTESIAN_POINT('Ctrl Pts',(-0.0248847564386643,0.00189105397096317,
0.00558743987649347));
#51896=CARTESIAN_POINT('Ctrl Pts',(-0.0250806101958126,0.00200380994308026,
0.00553329955785079));
#51897=CARTESIAN_POINT('Ctrl Pts',(-0.0251969754966454,0.00207080320788732,
0.0055011324217296));
#51898=CARTESIAN_POINT('Ctrl Pts',(-0.0253133795787861,0.00213803928365046,
0.00546964294750879));
#51899=CARTESIAN_POINT('Ctrl Pts',(-0.0254299810437924,0.00220515851977943,
0.00543888238066341));
#51900=CARTESIAN_POINT('Ctrl Pts',(-0.0257797854388112,0.00240651622816635,
0.00534660068012726));
#51901=CARTESIAN_POINT('Ctrl Pts',(-0.026131284877388,0.00260689990446499,
0.00526077943816682));
#51902=CARTESIAN_POINT('Ctrl Pts',(-0.0264893372228397,0.00279674832677038,
0.00518482321349141));
#51903=CARTESIAN_POINT('Ctrl Pts',(-0.0264943584335114,0.00279941069984568,
0.00518375802788164));
#51904=CARTESIAN_POINT('Ctrl Pts',(-0.0264993810855449,0.00280207069650618,
0.0051826944884762));
#51905=CARTESIAN_POINT('Ctrl Pts',(-0.0265044052058202,0.00280472828016308,
0.00518163259052267));
#51906=CARTESIAN_POINT('Ctrl Pts',(-0.0269770608500551,0.00305474656130141,
0.00508173210370392));
#51907=CARTESIAN_POINT('Ctrl Pts',(-0.0274625835314519,0.00328308994308195,
0.00499672802735591));
#51908=CARTESIAN_POINT('Ctrl Pts',(-0.0279619732697084,0.00347647507401588,
0.00491780008001345));
#51909=CARTESIAN_POINT('Ctrl Pts',(-0.028128375408712,0.00354091312104355,
0.00489150042213339));
#51910=CARTESIAN_POINT('Ctrl Pts',(-0.0282960786034483,0.00360180694979735,
0.00486620699844024));
#51911=CARTESIAN_POINT('Ctrl Pts',(-0.0284653497047326,0.00365860512073623,
0.00484126609095895));
#51912=CARTESIAN_POINT('Ctrl Pts',(-0.0288094782020681,0.00377407591916729,
0.00479056117471157));
#51913=CARTESIAN_POINT('Ctrl Pts',(-0.0291601534207853,0.00387258032277834,
0.00474130097945834));
#51914=CARTESIAN_POINT('Ctrl Pts',(-0.0295166264965012,0.00395137882575817,
0.00468944087823975));
#51915=CARTESIAN_POINT('Ctrl Pts',(-0.0296495805641012,0.00398076837073549,
0.00467009857198194));
#51916=CARTESIAN_POINT('Ctrl Pts',(-0.0297833918223292,0.00400739927173845,
0.00465035590312184));
#51917=CARTESIAN_POINT('Ctrl Pts',(-0.0299179316600492,0.00403142587061642,
0.00463026109732501));
#51918=CARTESIAN_POINT('Ctrl Pts',(-0.0301290446636343,0.00406912717560552,
0.00459872936010782));
#51919=CARTESIAN_POINT('Ctrl Pts',(-0.0303415965120746,0.00410071552300745,
0.00456669090118318));
#51920=CARTESIAN_POINT('Ctrl Pts',(-0.0305556012738504,0.00412637462228191,
0.00453376913295831));
#51921=CARTESIAN_POINT('Ctrl Pts',(-0.0312962755608384,0.00421518122126669,
0.00441982630755575));
#51922=CARTESIAN_POINT('Ctrl Pts',(-0.0320539645187785,0.00423329656380979,
0.00429539350663322));
#51923=CARTESIAN_POINT('Ctrl Pts',(-0.0328029016201836,0.0042087665877202,
0.00416971706663987));
#51924=CARTESIAN_POINT('Ctrl Pts',(-0.0364391610694963,0.00340557668880201,
-0.00293086975220482));
#51925=CARTESIAN_POINT('Ctrl Pts',(-0.0333515059907657,0.00231570437435815,
-0.00145682442346898));
#51926=CARTESIAN_POINT('Ctrl Pts',(-0.0306323136900912,3.78646002930885E-6,
-0.00106277624427272));
#51927=CARTESIAN_POINT('Ctrl Pts',(-0.0370882476239518,0.00326876767257525,
-0.00270781351667378));
#51928=CARTESIAN_POINT('Ctrl Pts',(-0.0336803404828681,0.00234022559976933,
-0.00130013403482534));
#51929=CARTESIAN_POINT('Ctrl Pts',(-0.0307001750317395,3.81513661006243E-6,
-0.0010227126334477));
#51930=CARTESIAN_POINT('Ctrl Pts',(-0.0380711951877001,0.00301807121471456,
-0.00226920015226592));
#51931=CARTESIAN_POINT('Ctrl Pts',(-0.034177376109665,0.00240378747134278,
-0.00103180215401773));
#51932=CARTESIAN_POINT('Ctrl Pts',(-0.030832739744055,3.89817058239106E-6,
-0.000927476398380698));
#51933=CARTESIAN_POINT('Ctrl Pts',(-0.0389548787833504,0.00272631412492715,
-0.0015547766452028));
#51934=CARTESIAN_POINT('Ctrl Pts',(-0.0346510542984124,0.00247046977074249,
-0.000698423070453612));
#51935=CARTESIAN_POINT('Ctrl Pts',(-0.0310253932093769,3.98754807420298E-6,
-0.000718402588876897));
#51936=CARTESIAN_POINT('Ctrl Pts',(-0.0394299081639852,0.00253997682056228,
-0.000776937711593115));
#51937=CARTESIAN_POINT('Ctrl Pts',(-0.0349404581571179,0.00249716840139465,
-0.000359675024101642));
#51938=CARTESIAN_POINT('Ctrl Pts',(-0.0311927692352808,4.02218976237312E-6,
-0.000404760023136305));
#51939=CARTESIAN_POINT('Ctrl Pts',(-0.0395722564060474,0.0024790222613675,
-1.15969768619817E-6));
#51940=CARTESIAN_POINT('Ctrl Pts',(-0.035039641525199,0.00250059432609173,
-5.23131714616352E-7));
#51941=CARTESIAN_POINT('Ctrl Pts',(-0.0312636285943568,4.02588199220811E-6,
-5.43240818511782E-7));
#51942=CARTESIAN_POINT('Ctrl Pts',(-0.0394285060247083,0.00254062091626967,
0.000782073488798124));
#51943=CARTESIAN_POINT('Ctrl Pts',(-0.0349395146745486,0.00249717010318348,
0.000361994712682985));
#51944=CARTESIAN_POINT('Ctrl Pts',(-0.0311921191911461,4.02220893042648E-6,
0.000407199219089637));
#51945=CARTESIAN_POINT('Ctrl Pts',(-0.0389546331855897,0.00272679970989166,
0.00155567037639612));
#51946=CARTESIAN_POINT('Ctrl Pts',(-0.0346508084577749,0.00247061634579135,
0.000698666670416455));
#51947=CARTESIAN_POINT('Ctrl Pts',(-0.0310250230018649,3.98777465588809E-6,
0.000718630607728727));
#51948=CARTESIAN_POINT('Ctrl Pts',(-0.0380701459630995,0.00301899823186677,
0.00227065266162116));
#51949=CARTESIAN_POINT('Ctrl Pts',(-0.0341767045856397,0.00240421141794788,
0.0010323670224691));
#51950=CARTESIAN_POINT('Ctrl Pts',(-0.0308322812675443,3.8988403441998E-6,
0.000927873377138205));
#51951=CARTESIAN_POINT('Ctrl Pts',(-0.03709649940938,0.00326823276024269,
0.0027060963939119));
#51952=CARTESIAN_POINT('Ctrl Pts',(-0.0336843534503945,0.00234128603914245,
0.00129828781356605));
#51953=CARTESIAN_POINT('Ctrl Pts',(-0.0307005310944394,3.81666377594922E-6,
0.00102250283151694));
#51954=CARTESIAN_POINT('Ctrl Pts',(-0.0364455123647001,0.00340591076454287,
0.00292997690155913));
#51955=CARTESIAN_POINT('Ctrl Pts',(-0.0333545450336161,0.002316762246266,
0.00145544770917396));
#51956=CARTESIAN_POINT('Ctrl Pts',(-0.0306323184676507,3.78802893956849E-6,
0.00106277396492297));
#51957=CARTESIAN_POINT('',(-0.0307218899246848,7.95071454126342E-5,-0.00107604988198002));
#51958=CARTESIAN_POINT('Origin',(-0.0367505097033021,-0.0089574493287422,
-0.0114196063907013));
#51959=CARTESIAN_POINT('Ctrl Pts',(-0.0307219761960901,7.95254459509771E-5,
0.00107599840369229));
#51960=CARTESIAN_POINT('Ctrl Pts',(-0.0307952892239638,7.23751598598542E-5,
0.00102702375505616));
#51961=CARTESIAN_POINT('Ctrl Pts',(-0.0308575640997885,6.60272950011091E-5,
0.000973667173881751));
#51962=CARTESIAN_POINT('Ctrl Pts',(-0.0309105260823048,6.0949682466073E-5,
0.000919868255617537));
#51963=CARTESIAN_POINT('Ctrl Pts',(-0.030939927140558,5.81309212559178E-5,
0.000890002584910073));
#51964=CARTESIAN_POINT('Ctrl Pts',(-0.0309663339185817,5.5725626318494E-5,
0.000860199941229648));
#51965=CARTESIAN_POINT('Ctrl Pts',(-0.0309891703178521,5.39114965788957E-5,
0.000832533674153722));
#51966=CARTESIAN_POINT('Ctrl Pts',(-0.0310271481280753,5.08945290545872E-5,
0.000786523608023947));
#51967=CARTESIAN_POINT('Ctrl Pts',(-0.0310563547759014,4.85596066354287E-5,
0.000744646729173092));
#51968=CARTESIAN_POINT('Ctrl Pts',(-0.0310830526124284,4.63540473445381E-5,
0.000701615877086658));
#51969=CARTESIAN_POINT('Ctrl Pts',(-0.0311013268778553,4.4844375358352E-5,
0.000672161909467244));
#51970=CARTESIAN_POINT('Ctrl Pts',(-0.0311184086269113,4.33922934027984E-5,
0.000642052125309306));
#51971=CARTESIAN_POINT('Ctrl Pts',(-0.0311354485141428,4.17989301285626E-5,
0.000608142095971056));
#51972=CARTESIAN_POINT('Ctrl Pts',(-0.0311673311584297,3.88176525061228E-5,
0.000544694410639605));
#51973=CARTESIAN_POINT('Ctrl Pts',(-0.0311994341201196,3.69670941630756E-5,
0.000469716090898414));
#51974=CARTESIAN_POINT('Ctrl Pts',(-0.0312241401658602,3.58729802009628E-5,
0.00039074032007412));
#51975=CARTESIAN_POINT('Ctrl Pts',(-0.0312319292952294,3.55280364861704E-5,
0.000365841455138563));
#51976=CARTESIAN_POINT('Ctrl Pts',(-0.0312390169873475,3.52581840626902E-5,
0.000340594862418149));
#51977=CARTESIAN_POINT('Ctrl Pts',(-0.0312453204200204,3.5051385148846E-5,
0.000315483955331365));
#51978=CARTESIAN_POINT('Ctrl Pts',(-0.0312716174731044,3.41886485579732E-5,
0.00021072470891631));
#51979=CARTESIAN_POINT('Ctrl Pts',(-0.0312835549901547,3.291925126843E-5,
0.000105666092760674));
#51980=CARTESIAN_POINT('Ctrl Pts',(-0.0312836230622852,3.28827347166887E-5,
4.69038162585774E-7));
#51981=CARTESIAN_POINT('Ctrl Pts',(-0.0312836911344156,3.28462181649474E-5,
-0.000104728016435503));
#51982=CARTESIAN_POINT('Ctrl Pts',(-0.0312718650099121,3.40805814071716E-5,
-0.000209842528665909));
#51983=CARTESIAN_POINT('Ctrl Pts',(-0.0312455288419261,3.49919317592131E-5,
-0.000314780646790837));
#51984=CARTESIAN_POINT('Ctrl Pts',(-0.0312392913232001,3.52077780770892E-5,
-0.000339634432551035));
#51985=CARTESIAN_POINT('Ctrl Pts',(-0.03123228377827,3.54866957373038E-5,
-0.000364608910458436));
#51986=CARTESIAN_POINT('Ctrl Pts',(-0.0312245862128562,3.58386645348763E-5,
-0.000389258505156901));
#51987=CARTESIAN_POINT('Ctrl Pts',(-0.0311997829739071,3.69727849638032E-5,
-0.000468684889271354));
#51988=CARTESIAN_POINT('Ctrl Pts',(-0.0311674726314981,3.88661463710896E-5,
-0.000544246841131906));
#51989=CARTESIAN_POINT('Ctrl Pts',(-0.0311354856583077,4.18439708565057E-5,
-0.000607984583139167));
#51990=CARTESIAN_POINT('Ctrl Pts',(-0.0311185461912651,4.34209490666401E-5,
-0.000641738429546463));
#51991=CARTESIAN_POINT('Ctrl Pts',(-0.0311015799906545,4.48476797169792E-5,
-0.000671707621614676));
#51992=CARTESIAN_POINT('Ctrl Pts',(-0.0310834529036156,4.63296669299169E-5,
-0.000700990744872741));
#51993=CARTESIAN_POINT('Ctrl Pts',(-0.0310567274409192,4.85146177657057E-5,
-0.000744163981509777));
#51994=CARTESIAN_POINT('Ctrl Pts',(-0.0310275253588562,5.08264957832321E-5,
-0.000786099484748195));
#51995=CARTESIAN_POINT('Ctrl Pts',(-0.0309894158192428,5.38536203572919E-5,
-0.000832278091066834));
#51996=CARTESIAN_POINT('Ctrl Pts',(-0.0309665454929332,5.56702606917277E-5,
-0.000859990831911842));
#51997=CARTESIAN_POINT('Ctrl Pts',(-0.0309401709900778,5.8085624176027E-5,
-0.000889753759681022));
#51998=CARTESIAN_POINT('Ctrl Pts',(-0.0309107199611745,6.09170276475944E-5,
-0.000919657366608743));
#51999=CARTESIAN_POINT('Ctrl Pts',(-0.0308578095907544,6.60037975184087E-5,
-0.00097338081799111));
#52000=CARTESIAN_POINT('Ctrl Pts',(-0.0307952836375779,7.23588730805084E-5,
-0.00102702773176624));
#52001=CARTESIAN_POINT('Ctrl Pts',(-0.0307218911474655,7.95069316882072E-5,
-0.00107604898256824));
#52002=CARTESIAN_POINT('Ctrl Pts',(-0.0306659720248312,3.23414461730682E-5,
-0.00106769530807909));
#52003=CARTESIAN_POINT('Ctrl Pts',(-0.0333716875076,0.0023228279927353,
-0.00146645907172397));
#52004=CARTESIAN_POINT('Ctrl Pts',(-0.0364391610694963,0.00340557668880201,
-0.0029308697522048));
#52005=CARTESIAN_POINT('Ctrl Pts',(-0.0304648451406503,3.25593610126452E-5,
-0.00118610079900385));
#52006=CARTESIAN_POINT('Ctrl Pts',(-0.033177519503754,0.00233892557013915,
-0.00154659656588374));
#52007=CARTESIAN_POINT('Ctrl Pts',(-0.036259057400032,0.00344353742848523,
-0.0029927617234314));
#52008=CARTESIAN_POINT('Ctrl Pts',(-0.0300655212000987,3.30036942474922E-5,
-0.00142117692855237));
#52009=CARTESIAN_POINT('Ctrl Pts',(-0.032787882853436,0.00237171648936093,
-0.00170736037005578));
#52010=CARTESIAN_POINT('Ctrl Pts',(-0.0358936020458381,0.00352256019043282,
-0.00311869399351504));
#52011=CARTESIAN_POINT('Ctrl Pts',(-0.0294730439529765,3.36869730645144E-5,
-0.00176993295614264));
#52012=CARTESIAN_POINT('Ctrl Pts',(-0.0321940369640194,0.00242192567971165,
-0.00195299737112982));
#52013=CARTESIAN_POINT('Ctrl Pts',(-0.0353202505619921,0.00365077259747625,
-0.00331582646852773));
#52014=CARTESIAN_POINT('Ctrl Pts',(-0.0288844566138175,3.43805751075243E-5,
-0.00211638087976133));
#52015=CARTESIAN_POINT('Ctrl Pts',(-0.0315837846962915,0.00247253394371439,
-0.00220730892162865));
#52016=CARTESIAN_POINT('Ctrl Pts',(-0.0347097518201094,0.0037892002750051,
-0.00352417393855777));
#52017=CARTESIAN_POINT('Ctrl Pts',(-0.0283946132121652,3.49644787594377E-5,
-0.00240470419248045));
#52018=CARTESIAN_POINT('Ctrl Pts',(-0.0310540109273581,0.00251466505539929,
-0.00243127336975895));
#52019=CARTESIAN_POINT('Ctrl Pts',(-0.034156713001383,0.0039137701019183,
-0.00371122941019911));
#52020=CARTESIAN_POINT('Ctrl Pts',(-0.0280011050394867,3.54363580167864E-5,
-0.00263633501468253));
#52021=CARTESIAN_POINT('Ctrl Pts',(-0.0306106703026876,0.00254828741318223,
-0.00262215176228272));
#52022=CARTESIAN_POINT('Ctrl Pts',(-0.0336756196744561,0.00401973235510397,
-0.00387342560833778));
#52023=CARTESIAN_POINT('Ctrl Pts',(-0.0277045049304437,3.57938454752424E-5,
-0.00281093281213578));
#52024=CARTESIAN_POINT('Ctrl Pts',(-0.0302660225247906,0.0025734969554845,
-0.00277278147548018));
#52025=CARTESIAN_POINT('Ctrl Pts',(-0.0332910571209545,0.00410268222584421,
-0.00400318713095339));
#52026=CARTESIAN_POINT('Ctrl Pts',(-0.0274056655920821,3.61568571396258E-5,
-0.00298686453896102));
#52027=CARTESIAN_POINT('Ctrl Pts',(-0.0299061539411528,0.00259878283369678,
-0.0029329650039485));
#52028=CARTESIAN_POINT('Ctrl Pts',(-0.0328771438690326,0.00418955458028497,
-0.0041435432325896));
#52029=CARTESIAN_POINT('Ctrl Pts',(-0.0271539582111298,3.64666901547067E-5,
-0.00313506846284764));
#52030=CARTESIAN_POINT('Ctrl Pts',(-0.029590063973267,0.00262005567911308,
-0.00307679824266307));
#52031=CARTESIAN_POINT('Ctrl Pts',(-0.0325013306245234,0.00426576503991228,
-0.00427235715587504));
#52032=CARTESIAN_POINT('Ctrl Pts',(-0.0269503393755227,3.6721787310625E-5,
-0.00325497529873103));
#52033=CARTESIAN_POINT('Ctrl Pts',(-0.0293243762770283,0.00263735268991712,
-0.00320018057455909));
#52034=CARTESIAN_POINT('Ctrl Pts',(-0.0321764258442447,0.00432954907901014,
-0.00438539085653449));
#52035=CARTESIAN_POINT('Ctrl Pts',(-0.0267962883207492,3.69178344365261E-5,
-0.00334570310540647));
#52036=CARTESIAN_POINT('Ctrl Pts',(-0.0291176448799536,0.00265052820534663,
-0.00329760173839145));
#52037=CARTESIAN_POINT('Ctrl Pts',(-0.0319185969267873,0.00437899055578669,
-0.0044762214375067));
#52038=CARTESIAN_POINT('Ctrl Pts',(-0.0266665944406192,3.70863136558612E-5,
-0.0034220962932131));
#52039=CARTESIAN_POINT('Ctrl Pts',(-0.0289380157869116,0.00266174944143041,
-0.00338361927320225));
#52040=CARTESIAN_POINT('Ctrl Pts',(-0.03168990188217,0.00442172936806749,
-0.00455806239367165));
#52041=CARTESIAN_POINT('Ctrl Pts',(-0.0265618958214666,3.72251893031226E-5,
-0.00348377426723578));
#52042=CARTESIAN_POINT('Ctrl Pts',(-0.0287890193227952,0.00267093562259292,
-0.0034559335693082));
#52043=CARTESIAN_POINT('Ctrl Pts',(-0.0314969971377745,0.00445701329688577,
-0.00462814357193572));
#52044=CARTESIAN_POINT('Ctrl Pts',(-0.0264828543740696,3.73316761200374E-5,
-0.00353034182108191));
#52045=CARTESIAN_POINT('Ctrl Pts',(-0.028674364485197,0.00267794695681193,
-0.00351209763611023));
#52046=CARTESIAN_POINT('Ctrl Pts',(-0.0313468383591297,0.00448406951464358,
-0.00468329547025618));
#52047=CARTESIAN_POINT('Ctrl Pts',(-0.0264032446328258,3.74410903480025E-5,
-0.00357724898004166));
#52048=CARTESIAN_POINT('Ctrl Pts',(-0.0285564496828184,0.00268512044202649,
-0.00357043197867147));
#52049=CARTESIAN_POINT('Ctrl Pts',(-0.0311905579210017,0.00451181067552851,
-0.00474142017246755));
#52050=CARTESIAN_POINT('Ctrl Pts',(-0.026336381527319,3.75344633438766E-5,
-0.00361664980215379));
#52051=CARTESIAN_POINT('Ctrl Pts',(-0.0284552362796348,0.00269121413078742,
-0.00362099712426088));
#52052=CARTESIAN_POINT('Ctrl Pts',(-0.0310548025406171,0.00453546900121625,
-0.00479255366026566));
#52053=CARTESIAN_POINT('Ctrl Pts',(-0.0262825439416979,3.76122232159902E-5,
-0.00364837848343752));
#52054=CARTESIAN_POINT('Ctrl Pts',(-0.0283720828908489,0.00269628089830896,
-0.00366293169460257));
#52055=CARTESIAN_POINT('Ctrl Pts',(-0.0309420996512683,0.00455497260274855,
-0.00483561125614202));
#52056=CARTESIAN_POINT('Ctrl Pts',(-0.0262419843009898,3.76684800715227E-5,
-0.00367228206963774));
#52057=CARTESIAN_POINT('Ctrl Pts',(-0.0283090423271439,0.00269992121442134,
-0.00369476448950497));
#52058=CARTESIAN_POINT('Ctrl Pts',(-0.0308563295614869,0.00456937467996215,
-0.00486834081427539));
#52059=CARTESIAN_POINT('Ctrl Pts',(-0.026208019901491,3.77262236784257E-5,
-0.00369230473668905));
#52060=CARTESIAN_POINT('Ctrl Pts',(-0.0282542595847076,0.00270371457179228,
-0.00372301745429584));
#52061=CARTESIAN_POINT('Ctrl Pts',(-0.0307805550690652,0.00458299051760416,
-0.00489846967193485));
#52062=CARTESIAN_POINT('Ctrl Pts',(-0.0261808045216819,3.77507625204141E-5,
-0.0037083394051121));
#52063=CARTESIAN_POINT('Ctrl Pts',(-0.0282127768541347,0.00270520608416526,
-0.0037435677573533));
#52064=CARTESIAN_POINT('Ctrl Pts',(-0.0307244920527542,0.00459080952707601,
-0.0049188319945771));
#52065=CARTESIAN_POINT('Ctrl Pts',(-0.0261636656099131,3.781705370848E-5,
-0.00371846090632498));
#52066=CARTESIAN_POINT('Ctrl Pts',(-0.0281799200617113,0.00270975005130535,
-0.00376216305046526));
#52067=CARTESIAN_POINT('Ctrl Pts',(-0.0306760558540184,0.00460301804700601,
-0.00494167931077386));
#52068=CARTESIAN_POINT('Ctrl Pts',(-0.0261518327430556,3.77620276636738E-5,
-0.00372540271260059));
#52069=CARTESIAN_POINT('Ctrl Pts',(-0.0281701564974934,0.0027057343796972,
-0.00376409478037424));
#52070=CARTESIAN_POINT('Ctrl Pts',(-0.0306677672477296,0.0045970237335782,
-0.00493804696372403));
#52071=CARTESIAN_POINT('Ctrl Pts',(-0.026144776878792,3.78895509816586E-5,
-0.00372961580310048));
#52072=CARTESIAN_POINT('Ctrl Pts',(-0.0281436128678637,0.00271471501069469,
-0.00378271465869179));
#52073=CARTESIAN_POINT('Ctrl Pts',(-0.0306224655607035,0.00461639993926548,
-0.00496693774563895));
#52074=CARTESIAN_POINT('Ctrl Pts',(-0.0261374135605129,3.81565997376382E-5,
-0.00373407433410709));
#52075=CARTESIAN_POINT('Ctrl Pts',(-0.0280980043109231,0.00273359669628745,
-0.00381711382495484));
#52076=CARTESIAN_POINT('Ctrl Pts',(-0.0305403726405734,0.00465570696437846,
-0.0050239034882587));
#52077=CARTESIAN_POINT('Ctrl Pts',(-0.0261281640494186,3.84630626987939E-5,
-0.0037396621267139));
#52078=CARTESIAN_POINT('Ctrl Pts',(-0.0280434152443195,0.00275526528829198,
-0.00385782364150545));
#52079=CARTESIAN_POINT('Ctrl Pts',(-0.0304426025519808,0.00470080251139039,
-0.00509131932699353));
#52080=CARTESIAN_POINT('Ctrl Pts',(-0.0261054356644294,3.93073156687108E-5,
-0.00375343659204118));
#52081=CARTESIAN_POINT('Ctrl Pts',(-0.0278926602692761,0.00281505248511113,
-0.00397082959078529));
#52082=CARTESIAN_POINT('Ctrl Pts',(-0.0301707424124219,0.00482364365284629,
-0.00528219616543048));
#52083=CARTESIAN_POINT('Ctrl Pts',(-0.0260771330242492,4.05187705868077E-5,
-0.00377066835420024));
#52084=CARTESIAN_POINT('Ctrl Pts',(-0.0276722875172353,0.00290083210877017,
-0.00413643781579527));
#52085=CARTESIAN_POINT('Ctrl Pts',(-0.0297686688678292,0.00499915145989499,
-0.00556598995984482));
#52086=CARTESIAN_POINT('Ctrl Pts',(-0.0260409078612633,4.28160435087016E-5,
-0.00379308713029676));
#52087=CARTESIAN_POINT('Ctrl Pts',(-0.0272167184552454,0.00306650436760558,
-0.00447832811660013));
#52088=CARTESIAN_POINT('Ctrl Pts',(-0.02894101596812,0.00530184713024665,
-0.00621428296024427));
#52089=CARTESIAN_POINT('Ctrl Pts',(-0.0260043538115754,4.48407708557987E-5,
-0.0038155958698829));
#52090=CARTESIAN_POINT('Ctrl Pts',(-0.0267800050596834,0.00321559967836929,
-0.00480317582103633));
#52091=CARTESIAN_POINT('Ctrl Pts',(-0.0281727309093209,0.00554213262362041,
-0.0068677022049604));
#52092=CARTESIAN_POINT('Ctrl Pts',(-0.0259607701533692,4.61221805003758E-5,
-0.00384194401496335));
#52093=CARTESIAN_POINT('Ctrl Pts',(-0.0264635524308429,0.00331280008633878,
-0.00503500639952359));
#52094=CARTESIAN_POINT('Ctrl Pts',(-0.0276519466871055,0.0056709408313574,
-0.00735233283735931));
#52095=CARTESIAN_POINT('Ctrl Pts',(-0.0259109208809971,4.70910894813173E-5,
-0.00387187549175774));
#52096=CARTESIAN_POINT('Ctrl Pts',(-0.026200151872293,0.00338747640947883,
-0.00522676295442198));
#52097=CARTESIAN_POINT('Ctrl Pts',(-0.027237389066601,0.00575939777742583,
-0.00775104175037189));
#52098=CARTESIAN_POINT('Ctrl Pts',(-0.0258623967014985,4.77672103359955E-5,
-0.00390090483387817));
#52099=CARTESIAN_POINT('Ctrl Pts',(-0.025995917206177,0.00344054815113673,
-0.0053746982282801));
#52100=CARTESIAN_POINT('Ctrl Pts',(-0.026929683601278,0.00581356526299246,
-0.00805724361079941));
#52101=CARTESIAN_POINT('Ctrl Pts',(-0.0258146910606012,4.82892558635125E-5,
-0.0039293909184561));
#52102=CARTESIAN_POINT('Ctrl Pts',(-0.0258238363018331,0.00348207689599807,
-0.00549910882314107));
#52103=CARTESIAN_POINT('Ctrl Pts',(-0.0266786334686938,0.00585101008285789,
-0.00831178973482216));
#52104=CARTESIAN_POINT('Ctrl Pts',(-0.0257518916199959,4.88478750726719E-5,
-0.00396684362353593));
#52105=CARTESIAN_POINT('Ctrl Pts',(-0.0256230629559801,0.00352712041636869,
-0.00564414155165935));
#52106=CARTESIAN_POINT('Ctrl Pts',(-0.0263940947126037,0.00588622677513632,
-0.00860493329766318));
#52107=CARTESIAN_POINT('Ctrl Pts',(-0.0256743693417282,4.9371818595519E-5,
-0.00401302077025589));
#52108=CARTESIAN_POINT('Ctrl Pts',(-0.0254088152555184,0.00357018457708517,
-0.00579897033516915));
#52109=CARTESIAN_POINT('Ctrl Pts',(-0.0261016797480758,0.00591221324371429,
-0.00891170623644723));
#52110=CARTESIAN_POINT('Ctrl Pts',(-0.0255832224951489,4.98366328551321E-5,
-0.00406726790446615));
#52111=CARTESIAN_POINT('Ctrl Pts',(-0.0251877774792792,0.00360923613531693,
-0.00595913824631443));
#52112=CARTESIAN_POINT('Ctrl Pts',(-0.0258107866044053,0.00592748036538003,
-0.0092212190412313));
#52113=CARTESIAN_POINT('Ctrl Pts',(-0.0254936679857824,5.01927210102786E-5,
-0.0041205400118894));
#52114=CARTESIAN_POINT('Ctrl Pts',(-0.0249911997814267,0.00363983237155333,
-0.00610211634548159));
#52115=CARTESIAN_POINT('Ctrl Pts',(-0.0255597507675584,0.00593263301939726,
-0.00949085425259816));
#52116=CARTESIAN_POINT('Ctrl Pts',(-0.0253758720415834,5.05651453544886E-5,
-0.0041905884775542));
#52117=CARTESIAN_POINT('Ctrl Pts',(-0.0247522793478318,0.00367260676775817,
-0.00627664770945765));
#52118=CARTESIAN_POINT('Ctrl Pts',(-0.0252623164499094,0.00593028312395291,
-0.00981230212490256));
#52119=CARTESIAN_POINT('Ctrl Pts',(-0.0252311192315282,5.0888763299654E-5,
-0.00427663842767887));
#52120=CARTESIAN_POINT('Ctrl Pts',(-0.0244864841034371,0.00370231723272169,
-0.00647221927186298));
#52121=CARTESIAN_POINT('Ctrl Pts',(-0.0249420453960832,0.00591497917482241,
-0.010160472132548));
#52122=CARTESIAN_POINT('Ctrl Pts',(-0.0250602889666802,5.11360242616874E-5,
-0.00437816818346445));
#52123=CARTESIAN_POINT('Ctrl Pts',(-0.0242010563876091,0.00372660364023652,
-0.00668426186641994));
#52124=CARTESIAN_POINT('Ctrl Pts',(-0.0246086007077068,0.00588499648903705,
-0.0105235090876737));
#52125=CARTESIAN_POINT('Ctrl Pts',(-0.0248917111638188,5.12844272019451E-5,
-0.00447834690785075));
#52126=CARTESIAN_POINT('Ctrl Pts',(-0.0239395957750621,0.00374282506840123,
-0.00688033142308394));
#52127=CARTESIAN_POINT('Ctrl Pts',(-0.0243106749899636,0.00584724957039815,
-0.0108472856043692));
#52128=CARTESIAN_POINT('Ctrl Pts',(-0.0246693003821806,5.13849543682559E-5,
-0.00461050700441935));
#52129=CARTESIAN_POINT('Ctrl Pts',(-0.0236148624308845,0.00375641825322508,
-0.00712603678614978));
#52130=CARTESIAN_POINT('Ctrl Pts',(-0.0239481818224663,0.00578962008503306,
-0.0112395797881903));
#52131=CARTESIAN_POINT('Ctrl Pts',(-0.0243953711908193,5.13711945846472E-5,
-0.00477327030270521));
#52132=CARTESIAN_POINT('Ctrl Pts',(-0.0232447751136219,0.00376172831682206,
-0.0074096868729248));
#52133=CARTESIAN_POINT('Ctrl Pts',(-0.0235452646130942,0.00570778643045448,
-0.0116715846411793));
#52134=CARTESIAN_POINT('Ctrl Pts',(-0.0240726649027794,5.12118187243539E-5,
-0.00496501010794583));
#52135=CARTESIAN_POINT('Ctrl Pts',(-0.0228405020174707,0.00375586822790691,
-0.00772394722759367));
#52136=CARTESIAN_POINT('Ctrl Pts',(-0.0231148301912106,0.00560105104734249,
-0.0121256226619798));
#52137=CARTESIAN_POINT('Ctrl Pts',(-0.0236480460595398,5.08634391604083E-5,
-0.00521729715840131));
#52138=CARTESIAN_POINT('Ctrl Pts',(-0.0223393718662674,0.00373624599895701,
-0.00811812347554683));
#52139=CARTESIAN_POINT('Ctrl Pts',(-0.022590417361574,0.00545157456564356,
-0.0126684112001716));
#52140=CARTESIAN_POINT('Ctrl Pts',(-0.0231256191168733,5.02401014976624E-5,
-0.0055276861175585));
#52141=CARTESIAN_POINT('Ctrl Pts',(-0.0217671013382464,0.00369518212874887,
-0.0085748562026785));
#52142=CARTESIAN_POINT('Ctrl Pts',(-0.0220027039981841,0.00525666829407956,
-0.0132572883380559));
#52143=CARTESIAN_POINT('Ctrl Pts',(-0.022506802832622,4.93019261157021E-5,
-0.00589531188146266));
#52144=CARTESIAN_POINT('Ctrl Pts',(-0.021134550013562,0.00362896008264994,
-0.00908521441965309));
#52145=CARTESIAN_POINT('Ctrl Pts',(-0.0213625517960801,0.00501846018383101,
-0.0138697797012409));
#52146=CARTESIAN_POINT('Ctrl Pts',(-0.0216884633928667,4.78671456038939E-5,
-0.00638140703944321));
#52147=CARTESIAN_POINT('Ctrl Pts',(-0.0203407251070505,0.00352427154951466,
-0.00972847192511815));
#52148=CARTESIAN_POINT('Ctrl Pts',(-0.0205673942342202,0.0047004754260775,
-0.0145940979045826));
#52149=CARTESIAN_POINT('Ctrl Pts',(-0.0210778116756395,4.66312446128068E-5,
-0.00674404056932037));
#52150=CARTESIAN_POINT('Ctrl Pts',(-0.019783209720137,0.0034317380242369,
-0.0101790687897771));
#52151=CARTESIAN_POINT('Ctrl Pts',(-0.0200147944465283,0.0044649192266308,
-0.0150590894458486));
#52152=CARTESIAN_POINT('Ctrl Pts',(-0.0206712477487095,4.5762457771723E-5,
-0.00698541821209234));
#52153=CARTESIAN_POINT('Ctrl Pts',(-0.0194199829425201,0.00336621201589046,
-0.0104694405421481));
#52154=CARTESIAN_POINT('Ctrl Pts',(-0.0196565859278358,0.00431125424739362,
-0.0153459530959679));
#52155=CARTESIAN_POINT('',(-0.0207149455870811,8.43554850505981E-5,-0.00699117714093166));
#52156=CARTESIAN_POINT('Ctrl Pts',(-0.0327968762032639,0.00420554807594454,
-0.00417120478069329));
#52157=CARTESIAN_POINT('Ctrl Pts',(-0.0317030654778017,0.00424097888210346,
-0.00435540229680534));
#52158=CARTESIAN_POINT('Ctrl Pts',(-0.0295266041626024,0.00414882581713682,
-0.00470177324033703));
#52159=CARTESIAN_POINT('Ctrl Pts',(-0.0264213259365022,0.00288385212068659,
-0.00513303967806249));
#52160=CARTESIAN_POINT('Ctrl Pts',(-0.0236967389144328,0.00113672339326093,
-0.00593058660740073));
#52161=CARTESIAN_POINT('Ctrl Pts',(-0.0217311533549796,0.000374146536090822,
-0.00662175902642767));
#52162=CARTESIAN_POINT('Ctrl Pts',(-0.0207149455884397,8.4355483057549E-5,
-0.00699117714319741));
#52163=CARTESIAN_POINT('',(-0.0263907115489401,0.00012245196838643,-0.00362513812701022));
#52164=CARTESIAN_POINT('Ctrl Pts',(-0.0207149455828892,8.4355490703393E-5,
-0.006991177133933));
#52165=CARTESIAN_POINT('Ctrl Pts',(-0.0210971425310402,8.77204073903474E-5,
-0.00676497304784093));
#52166=CARTESIAN_POINT('Ctrl Pts',(-0.0214863236218676,9.05689834324322E-5,
-0.00653393795875628));
#52167=CARTESIAN_POINT('Ctrl Pts',(-0.0218760532400046,9.32600036074344E-5,
-0.00630236302065223));
#52168=CARTESIAN_POINT('Ctrl Pts',(-0.022080500283299,9.46716774772691E-5,
-0.00618088184705613));
#52169=CARTESIAN_POINT('Ctrl Pts',(-0.0222850980092275,9.60418134407925E-5,
-0.00605925085010957));
#52170=CARTESIAN_POINT('Ctrl Pts',(-0.022489291818599,9.74297572472183E-5,
-0.00593785507351048));
#52171=CARTESIAN_POINT('Ctrl Pts',(-0.0226961163953625,9.8835582875424E-5,
-0.00581489527275426));
#52172=CARTESIAN_POINT('Ctrl Pts',(-0.0229025297706422,0.000100259754044708,
-0.00569217496529666));
#52173=CARTESIAN_POINT('Ctrl Pts',(-0.0231078996179027,0.000101763864891936,
-0.00557011741350745));
#52174=CARTESIAN_POINT('Ctrl Pts',(-0.0233182839071471,0.000103304701074851,
-0.00544507962620509));
#52175=CARTESIAN_POINT('Ctrl Pts',(-0.0235275821357207,0.000104929497605713,
-0.00532073201507991));
#52176=CARTESIAN_POINT('Ctrl Pts',(-0.0237353773562675,0.000106690091906569,
-0.00519735968999793));
#52177=CARTESIAN_POINT('Ctrl Pts',(-0.0238420277422174,0.000107593712601952,
-0.00513403914753832));
#52178=CARTESIAN_POINT('Ctrl Pts',(-0.023948279138249,0.000108533185086646,
-0.00507097714903515));
#52179=CARTESIAN_POINT('Ctrl Pts',(-0.0240540984753581,0.000109511365780083,
-0.00500819657265365));
#52180=CARTESIAN_POINT('Ctrl Pts',(-0.0241623291302322,0.00011051183639281,
-0.00494398540784414));
#52181=CARTESIAN_POINT('Ctrl Pts',(-0.0242701098690006,0.00011155278958794,
-0.00488006741271473));
#52182=CARTESIAN_POINT('Ctrl Pts',(-0.0243775251874332,0.000112632461217019,
-0.00481639370375624));
#52183=CARTESIAN_POINT('Ctrl Pts',(-0.0244878858778078,0.000113741737883529,
-0.00475097403566873));
#52184=CARTESIAN_POINT('Ctrl Pts',(-0.0245978582774167,0.000114891830942718,
-0.00468581373652554));
#52185=CARTESIAN_POINT('Ctrl Pts',(-0.0247073028057999,0.000116066635648145,
-0.00462099409244789));
#52186=CARTESIAN_POINT('Ctrl Pts',(-0.0247633267969307,0.000116668011060599,
-0.00458781330928266));
#52187=CARTESIAN_POINT('Ctrl Pts',(-0.0248192121921035,0.000117275872470403,
-0.00455472194213076));
#52188=CARTESIAN_POINT('Ctrl Pts',(-0.0248749543343892,0.00011788541951887,
-0.00452172172282054));
#52189=CARTESIAN_POINT('Ctrl Pts',(-0.024931690820346,0.0001185058398353,
-0.00448813283651845));
#52190=CARTESIAN_POINT('Ctrl Pts',(-0.0249882794376936,0.00011912799642088,
-0.00445463805534672));
#52191=CARTESIAN_POINT('Ctrl Pts',(-0.0250447742563322,0.000119743657011892,
-0.00442120295626946));
#52192=CARTESIAN_POINT('Ctrl Pts',(-0.0251023743207899,0.000120371362181692,
-0.0043871137440477));
#52193=CARTESIAN_POINT('Ctrl Pts',(-0.0251598771560652,0.000120992292342631,
-0.00435308640225312));
#52194=CARTESIAN_POINT('Ctrl Pts',(-0.0252173636492093,0.000121591559253424,
-0.0043190684232904));
#52195=CARTESIAN_POINT('Ctrl Pts',(-0.0252760858756926,0.00012220370804412,
-0.00428431919167278));
#52196=CARTESIAN_POINT('Ctrl Pts',(-0.0253347920219821,0.000122793183487558,
-0.00424957913155028));
#52197=CARTESIAN_POINT('Ctrl Pts',(-0.0253936652971408,0.000123327091914099,
-0.00421472854072798));
#52198=CARTESIAN_POINT('Ctrl Pts',(-0.0254236140176411,0.000123598690091644,
-0.00419700011299922));
#52199=CARTESIAN_POINT('Ctrl Pts',(-0.0254536056518887,0.000123855923585816,
-0.00417924328455579));
#52200=CARTESIAN_POINT('Ctrl Pts',(-0.025483680306593,0.000124090809101317,
-0.00416143145143432));
#52201=CARTESIAN_POINT('Ctrl Pts',(-0.0255141264866617,0.000124328596260332,
-0.00414339958094724));
#52202=CARTESIAN_POINT('Ctrl Pts',(-0.0255446579384126,0.000124543468298433,
-0.00412531122314441));
#52203=CARTESIAN_POINT('Ctrl Pts',(-0.0255753507891367,0.000124722389861798,
-0.00410711639013784));
#52204=CARTESIAN_POINT('Ctrl Pts',(-0.0256064423089494,0.000124903635435311,
-0.00408868522465257));
#52205=CARTESIAN_POINT('Ctrl Pts',(-0.0256376993502233,0.000125047966296222,
-0.00407014484895584));
#52206=CARTESIAN_POINT('Ctrl Pts',(-0.0256691971115749,0.000125132429964907,
-0.00405144207391461));
#52207=CARTESIAN_POINT('Ctrl Pts',(-0.0256838674422491,0.000125171769584499,
-0.00404273110898868));
#52208=CARTESIAN_POINT('Ctrl Pts',(-0.0256985899060688,0.000125198128355305,
-0.00403398496786023));
#52209=CARTESIAN_POINT('Ctrl Pts',(-0.0257133663180243,0.000125206745692729,
-0.00402520073294849));
#52210=CARTESIAN_POINT('Ctrl Pts',(-0.0257310516727892,0.000125217059473227,
-0.00401468719886324));
#52211=CARTESIAN_POINT('Ctrl Pts',(-0.0257484825402284,0.000125339361806644,
-0.00400438085172023));
#52212=CARTESIAN_POINT('Ctrl Pts',(-0.0257657329491683,0.000125544176069823,
-0.00399422365467317));
#52213=CARTESIAN_POINT('Ctrl Pts',(-0.0257823462027672,0.00012574142538181,
-0.00398444162046256));
#52214=CARTESIAN_POINT('Ctrl Pts',(-0.0257987928730291,0.000126015157500993,
-0.0039747974374639));
#52215=CARTESIAN_POINT('Ctrl Pts',(-0.0258151980186753,0.0001263309593292,
-0.00396520106776497));
#52216=CARTESIAN_POINT('Ctrl Pts',(-0.0258320993572177,0.00012665631295458,
-0.00395531444459447));
#52217=CARTESIAN_POINT('Ctrl Pts',(-0.0258489562467072,0.000127026371687109,
-0.00394547881739026));
#52218=CARTESIAN_POINT('Ctrl Pts',(-0.0258659177543635,0.000127395692270414,
-0.00393558539541793));
#52219=CARTESIAN_POINT('Ctrl Pts',(-0.025883265195321,0.000127773416181702,
-0.0039254668636806));
#52220=CARTESIAN_POINT('Ctrl Pts',(-0.0259007216997102,0.000128150501446182,
-0.00391528815415423));
#52221=CARTESIAN_POINT('Ctrl Pts',(-0.0259185665436356,0.00012843687551344,
-0.00390484414244605));
#52222=CARTESIAN_POINT('Ctrl Pts',(-0.0259366611520451,0.000128727257801305,
-0.00389425395163948));
#52223=CARTESIAN_POINT('Ctrl Pts',(-0.0259551529365133,0.000128925110284922,
-0.00388339255718412));
#52224=CARTESIAN_POINT('Ctrl Pts',(-0.0259745838996711,0.000128865299578265,
-0.00387186678728443));
#52225=CARTESIAN_POINT('Ctrl Pts',(-0.0259941009118485,0.000128805224002974,
-0.00386028997610637));
#52226=CARTESIAN_POINT('Ctrl Pts',(-0.0260145501188438,0.000128491487357182,
-0.0038480546690898));
#52227=CARTESIAN_POINT('Ctrl Pts',(-0.0260374058089729,0.000127165890519034,
-0.00383395735489107));
#52228=CARTESIAN_POINT('Ctrl Pts',(-0.0260488015913114,0.000126504951691511,
-0.00382692847397526));
#52229=CARTESIAN_POINT('Ctrl Pts',(-0.0260608038279689,0.000125589576025012,
-0.00381943053662304));
#52230=CARTESIAN_POINT('Ctrl Pts',(-0.0260729178646133,0.000124548724251656,
-0.00381181917277744));
#52231=CARTESIAN_POINT('Ctrl Pts',(-0.0260849702930928,0.00012351316592173,
-0.00380424651792476));
#52232=CARTESIAN_POINT('Ctrl Pts',(-0.026097136401074,0.000122351777904879,
-0.0037965591434672));
#52233=CARTESIAN_POINT('Ctrl Pts',(-0.0261086052243113,0.000121387047784687,
-0.00378937964865003));
#52234=CARTESIAN_POINT('Ctrl Pts',(-0.026131264223562,0.000119481026685734,
-0.00377519509245661));
#52235=CARTESIAN_POINT('Ctrl Pts',(-0.0261511521497109,0.000118360387665682,
-0.00376303046579071));
#52236=CARTESIAN_POINT('Ctrl Pts',(-0.0261698961696417,0.000117479077949222,
-0.0037516577649883));
#52237=CARTESIAN_POINT('Ctrl Pts',(-0.0261745200568637,0.000117261671184203,
-0.00374885227896585));
#52238=CARTESIAN_POINT('Ctrl Pts',(-0.0261790760477508,0.000117058244254152,
-0.00374609367896718));
#52239=CARTESIAN_POINT('Ctrl Pts',(-0.0261835583029753,0.000116877142890749,
-0.00374338935602184));
#52240=CARTESIAN_POINT('Ctrl Pts',(-0.0261880122804294,0.000116697184064419,
-0.00374070209418065));
#52241=CARTESIAN_POINT('Ctrl Pts',(-0.0261923929005556,0.000116539567001617,
-0.003738068887214));
#52242=CARTESIAN_POINT('Ctrl Pts',(-0.0261967973758367,0.000116354157551165,
-0.0037354094319082));
#52243=CARTESIAN_POINT('Ctrl Pts',(-0.0262011720497276,0.00011617000261096,
-0.00373276797090596));
#52244=CARTESIAN_POINT('Ctrl Pts',(-0.0262054331910358,0.000116028478557896,
-0.00373021344893865));
#52245=CARTESIAN_POINT('Ctrl Pts',(-0.0262092655210476,0.000116119637537204,
-0.00372801812796615));
#52246=CARTESIAN_POINT('Ctrl Pts',(-0.026213070257243,0.000116210140147112,
-0.00372583861390066));
#52247=CARTESIAN_POINT('Ctrl Pts',(-0.0262165886660585,0.000116460366263563,
-0.00372390094085995));
#52248=CARTESIAN_POINT('Ctrl Pts',(-0.0262201693461397,0.000116679298603018,
-0.00372191249859911));
#52249=CARTESIAN_POINT('Ctrl Pts',(-0.0262272477875872,0.000117112093410339,
-0.00371798166093806));
#52250=CARTESIAN_POINT('Ctrl Pts',(-0.0262345801580936,0.000117416809093337,
-0.00371384355418574));
#52251=CARTESIAN_POINT('Ctrl Pts',(-0.0262419010935463,0.000117740035136958,
-0.00370972144139412));
#52252=CARTESIAN_POINT('Ctrl Pts',(-0.0262491002484858,0.000118057884458753,
-0.00370566789811987));
#52253=CARTESIAN_POINT('Ctrl Pts',(-0.0262562845165814,0.000118395727247598,
-0.00370163303098062));
#52254=CARTESIAN_POINT('Ctrl Pts',(-0.0262635258941543,0.000118715228742628,
-0.00369755689516486));
#52255=CARTESIAN_POINT('Ctrl Pts',(-0.0262776136679998,0.000119336804507724,
-0.00368962695656447));
#52256=CARTESIAN_POINT('Ctrl Pts',(-0.0262919220400696,0.000119886589927717,
-0.0036815371309529));
#52257=CARTESIAN_POINT('Ctrl Pts',(-0.0263064318609315,0.000120380521748309,
-0.00367330567369189));
#52258=CARTESIAN_POINT('Ctrl Pts',(-0.0263203695794753,0.000120854978515265,
-0.00366539877149084));
#52259=CARTESIAN_POINT('Ctrl Pts',(-0.0263344916015547,0.000121278768971522,
-0.00365736250963555));
#52260=CARTESIAN_POINT('Ctrl Pts',(-0.0263488388037353,0.000121633145238242,
-0.00364916383368701));
#52261=CARTESIAN_POINT('Ctrl Pts',(-0.026362581742611,0.000121972596185628,
-0.00364131046262522));
#52262=CARTESIAN_POINT('Ctrl Pts',(-0.0263765316258872,0.000122248123640011,
-0.00363330776749834));
#52263=CARTESIAN_POINT('Ctrl Pts',(-0.0263907115489401,0.00012245196838643,
-0.00362513812701022));
#52264=CARTESIAN_POINT('Ctrl Pts',(-0.0263907115489401,0.00012245196838643,
-0.00362513812701022));
#52265=CARTESIAN_POINT('Ctrl Pts',(-0.0264171761508432,0.000122832412627479,
-0.00360989077465136));
#52266=CARTESIAN_POINT('Ctrl Pts',(-0.0264444422376895,0.000122963349712034,
-0.00359406200184561));
#52267=CARTESIAN_POINT('Ctrl Pts',(-0.0264726701882212,0.00012278141785782,
-0.00357752387041932));
#52268=CARTESIAN_POINT('Ctrl Pts',(-0.0264996579116161,0.000122607479386702,
-0.00356171236062163));
#52269=CARTESIAN_POINT('Ctrl Pts',(-0.0265266118581404,0.000122429453145089,
-0.00354592056709213));
#52270=CARTESIAN_POINT('Ctrl Pts',(-0.0265535379300483,0.000122247732016571,
-0.00353014495734327));
#52271=CARTESIAN_POINT('Ctrl Pts',(-0.02658023466759,0.000122067558640728,
-0.00351450371139899));
#52272=CARTESIAN_POINT('Ctrl Pts',(-0.0266069040078998,0.00012188375435418,
-0.00349887837252222));
#52273=CARTESIAN_POINT('Ctrl Pts',(-0.0266335514523883,0.000121696211892216,
-0.00348326543551233));
#52274=CARTESIAN_POINT('Ctrl Pts',(-0.0266600345193917,0.000121509826305098,
-0.00346774880850032));
#52275=CARTESIAN_POINT('Ctrl Pts',(-0.0266864959648013,0.000121319748016962,
-0.00345224442761254));
#52276=CARTESIAN_POINT('Ctrl Pts',(-0.0267129404584668,0.000121126029854152,
-0.00343674936402911));
#52277=CARTESIAN_POINT('Ctrl Pts',(-0.0267653682442451,0.000120741972043495,
-0.00340602947638643));
#52278=CARTESIAN_POINT('Ctrl Pts',(-0.0268177291022766,0.000120343614098467,
-0.00337534639126105));
#52279=CARTESIAN_POINT('Ctrl Pts',(-0.0268700516966129,0.000119931394892243,
-0.00334468198505257));
#52280=CARTESIAN_POINT('Ctrl Pts',(-0.0269218089411547,0.000119523629747338,
-0.00331434891019279));
#52281=CARTESIAN_POINT('Ctrl Pts',(-0.0269735288387845,0.000119102298826571,
-0.00328403405446561));
#52282=CARTESIAN_POINT('Ctrl Pts',(-0.0270252313788013,0.000118668086148498,
-0.00325372470877414));
#52283=CARTESIAN_POINT('Ctrl Pts',(-0.0270764227408043,0.000118238166489188,
-0.00322371502865278));
#52284=CARTESIAN_POINT('Ctrl Pts',(-0.0271275971424334,0.000117795617288825,
-0.00319371071572467));
#52285=CARTESIAN_POINT('Ctrl Pts',(-0.0271787707685532,0.000117341194417889,
-0.00316370145968983));
#52286=CARTESIAN_POINT('Ctrl Pts',(-0.0272797781160699,0.000116444247058001,
-0.00310446869502455));
#52287=CARTESIAN_POINT('Ctrl Pts',(-0.0273807806169518,0.00011550107514636,
-0.00304521774020601));
#52288=CARTESIAN_POINT('Ctrl Pts',(-0.0274818564446264,0.000114518630178686,
-0.00298589831181024));
#52289=CARTESIAN_POINT('Ctrl Pts',(-0.0275814324031909,0.000113550763759545,
-0.00292745912728996));
#52290=CARTESIAN_POINT('Ctrl Pts',(-0.0276810803813479,0.000112544768962472,
-0.00286895296322468));
#52291=CARTESIAN_POINT('Ctrl Pts',(-0.0277808389005263,0.000111508039264204,
-0.00281035472927768));
#52292=CARTESIAN_POINT('Ctrl Pts',(-0.0278794032326279,0.000110483720026896,
-0.00275245796177459));
#52293=CARTESIAN_POINT('Ctrl Pts',(-0.0279780759843496,0.000109429392354947,
-0.00269447100441981));
#52294=CARTESIAN_POINT('Ctrl Pts',(-0.0280768730639752,0.000108352484990015,
-0.0026363834400703));
#52295=CARTESIAN_POINT('Ctrl Pts',(-0.0281747495507818,0.000107285612265689,
-0.0025788371366044));
#52296=CARTESIAN_POINT('Ctrl Pts',(-0.028272748385646,0.000106196576723287,
-0.00252119189380465));
#52297=CARTESIAN_POINT('Ctrl Pts',(-0.0283708734488242,0.000105092655406102,
-0.00246344543367369));
#52298=CARTESIAN_POINT('Ctrl Pts',(-0.028565352107592,0.000102904742041281,
-0.00234899501956838));
#52299=CARTESIAN_POINT('Ctrl Pts',(-0.0287603242758405,0.000100658659497398,
-0.00223414774060621));
#52300=CARTESIAN_POINT('Ctrl Pts',(-0.0289556651769592,9.84109625647153E-5,
-0.00211898938119166));
#52301=CARTESIAN_POINT('Ctrl Pts',(-0.0291501751539627,9.61728266895183E-5,
-0.00200432087237855));
#52302=CARTESIAN_POINT('Ctrl Pts',(-0.0293450551540655,9.39331173919207E-5,
-0.00188934131721124));
#52303=CARTESIAN_POINT('Ctrl Pts',(-0.0295400270379856,9.17454444355415E-5,
-0.00177424100944673));
#52304=CARTESIAN_POINT('Ctrl Pts',(-0.0297359665809972,8.95469139053263E-5,
-0.00165856945080742));
#52305=CARTESIAN_POINT('Ctrl Pts',(-0.0299320019424413,8.74009587179148E-5,
-0.00154277419702442));
#52306=CARTESIAN_POINT('Ctrl Pts',(-0.0301277191821847,8.53581722133113E-5,
-0.00142713864495516));
#52307=CARTESIAN_POINT('Ctrl Pts',(-0.0303262937420681,8.32855626076416E-5,
-0.00130981490337201));
#52308=CARTESIAN_POINT('Ctrl Pts',(-0.0305245431904343,8.13191571505584E-5,
-0.00119265422654581));
#52309=CARTESIAN_POINT('Ctrl Pts',(-0.0307218894713725,7.95072456744465E-5,
-0.0010760502337852));
#52310=CARTESIAN_POINT('Ctrl Pts',(-0.0306647100227538,0.0133817289939493,
0.00107038503556915));
#52311=CARTESIAN_POINT('Ctrl Pts',(-0.0326595892334205,0.0123956391197582,
0.00151856505842931));
#52312=CARTESIAN_POINT('Ctrl Pts',(-0.0347612555974135,0.0120023262382354,
0.0022808544455469));
#52313=CARTESIAN_POINT('Ctrl Pts',(-0.030310636551541,0.0133810659960543,
0.00127926136827211));
#52314=CARTESIAN_POINT('Ctrl Pts',(-0.0323497877072503,0.0123587012333725,
0.00167896524445854));
#52315=CARTESIAN_POINT('Ctrl Pts',(-0.034504793762637,0.0119445902306563,
0.00241834291186082));
#52316=CARTESIAN_POINT('Ctrl Pts',(-0.0297913734877477,0.0133800176106531,
0.00158555997177866));
#52317=CARTESIAN_POINT('Ctrl Pts',(-0.0318905638771274,0.0123002313925209,
0.0019156374684094));
#52318=CARTESIAN_POINT('Ctrl Pts',(-0.0341203946096195,0.0118503203309816,
0.00262684653906666));
#52319=CARTESIAN_POINT('Ctrl Pts',(-0.0291134934790883,0.0133785311643582,
0.00198536147749519));
#52320=CARTESIAN_POINT('Ctrl Pts',(-0.0312684820519487,0.0122173215410984,
0.00223441391922514));
#52321=CARTESIAN_POINT('Ctrl Pts',(-0.0335750408273263,0.011704437060625,
0.00292061820949249));
#52322=CARTESIAN_POINT('Ctrl Pts',(-0.0286118977302727,0.0133773896440105,
0.0022811564471782));
#52323=CARTESIAN_POINT('Ctrl Pts',(-0.0307925845250482,0.01215366539174,
0.00247725318869305));
#52324=CARTESIAN_POINT('Ctrl Pts',(-0.0331409841609045,0.0115848853141045,
0.00315017909741456));
#52325=CARTESIAN_POINT('Ctrl Pts',(-0.0281126430422037,0.0133762319068543,
0.00257552991505409));
#52326=CARTESIAN_POINT('Ctrl Pts',(-0.0302988214468626,0.0120892008773578,
0.00272828796853001));
#52327=CARTESIAN_POINT('Ctrl Pts',(-0.0326684603969548,0.0114545241332851,
0.00339268193636275));
#52328=CARTESIAN_POINT('Ctrl Pts',(-0.0276951505456185,0.0133752613449626,
0.00282166534044536));
#52329=CARTESIAN_POINT('Ctrl Pts',(-0.0298640741459918,0.012035324868911,
0.00294920645759005));
#52330=CARTESIAN_POINT('Ctrl Pts',(-0.032228445307703,0.0113361163108333,
0.00361037592292299));
#52331=CARTESIAN_POINT('Ctrl Pts',(-0.0273575350888643,0.0133744837085808,
0.00302070115664028));
#52332=CARTESIAN_POINT('Ctrl Pts',(-0.029494718935472,0.0119923276822167,
0.00313769691396422));
#52333=CARTESIAN_POINT('Ctrl Pts',(-0.0318356844891301,0.0112346920460384,
0.00379925579609339));
#52334=CARTESIAN_POINT('Ctrl Pts',(-0.0271014943685578,0.0133738994060875,
0.00317164659443028));
#52335=CARTESIAN_POINT('Ctrl Pts',(-0.0292040699863256,0.0119601333248718,
0.00328676937427297));
#52336=CARTESIAN_POINT('Ctrl Pts',(-0.0315157814755496,0.0111548954586693,
0.00395056806280461));
#52337=CARTESIAN_POINT('Ctrl Pts',(-0.0268419576648391,0.0133733140263834,
0.00332465983562304));
#52338=CARTESIAN_POINT('Ctrl Pts',(-0.0288967835006665,0.0119280218878657,
0.00344558010096036));
#52339=CARTESIAN_POINT('Ctrl Pts',(-0.0311649277071802,0.0110710448872296,
0.00411429689112972));
#52340=CARTESIAN_POINT('Ctrl Pts',(-0.0266218956812325,0.0133728240133568,
0.00345441321228898));
#52341=CARTESIAN_POINT('Ctrl Pts',(-0.0286232624088187,0.0119012878231247,
0.00358846874310371));
#52342=CARTESIAN_POINT('Ctrl Pts',(-0.0308402062025501,0.0109973491206113,
0.00426454079291036));
#52343=CARTESIAN_POINT('Ctrl Pts',(-0.0264426154949514,0.013372428117788,
0.00356013525965011));
#52344=CARTESIAN_POINT('Ctrl Pts',(-0.0283904928968428,0.0118797957211661,
0.00371145103963453));
#52345=CARTESIAN_POINT('Ctrl Pts',(-0.0305548268488704,0.0109355978828558,
0.00439649850200783));
#52346=CARTESIAN_POINT('Ctrl Pts',(-0.0263062381182183,0.013372128177494,
0.00364056700768389));
#52347=CARTESIAN_POINT('Ctrl Pts',(-0.0282077567550798,0.0118635729881128,
0.00380883303996754));
#52348=CARTESIAN_POINT('Ctrl Pts',(-0.0303258278247013,0.0108877104255634,
0.00450262867601729));
#52349=CARTESIAN_POINT('Ctrl Pts',(-0.0261675735544255,0.013371823712976,
0.00372236023559422));
#52350=CARTESIAN_POINT('Ctrl Pts',(-0.0280153629006738,0.0118471690739344,
0.00391238329445619));
#52351=CARTESIAN_POINT('Ctrl Pts',(-0.0300792020978235,0.0108380258906879,
0.00461754277182759));
#52352=CARTESIAN_POINT('Ctrl Pts',(-0.0260497293451323,0.013371564385799,
0.00379188598430727));
#52353=CARTESIAN_POINT('Ctrl Pts',(-0.0278453661367971,0.0118332520622813,
0.00400492992782623));
#52354=CARTESIAN_POINT('Ctrl Pts',(-0.0298561034875484,0.010794879939539,
0.0047224470878419));
#52355=CARTESIAN_POINT('Ctrl Pts',(-0.0259537718308825,0.0133713518373242,
0.00384850991985681));
#52356=CARTESIAN_POINT('Ctrl Pts',(-0.0277022450165804,0.0118218790838674,
0.00408363726935057));
#52357=CARTESIAN_POINT('Ctrl Pts',(-0.029664710102224,0.0107591135472417,
0.00481341043608701));
#52358=CARTESIAN_POINT('Ctrl Pts',(-0.0258808773556986,0.0133711892996174,
0.00389153078810256));
#52359=CARTESIAN_POINT('Ctrl Pts',(-0.027590940482112,0.0118131989895311,
0.0041452868158749));
#52360=CARTESIAN_POINT('Ctrl Pts',(-0.0295139672710111,0.0107316023319646,
0.00488565938487552));
#52361=CARTESIAN_POINT('Ctrl Pts',(-0.0258069055623551,0.0133710227826421,
0.00393519478889492));
#52362=CARTESIAN_POINT('Ctrl Pts',(-0.0274751026803282,0.0118043218687226,
0.00420994459989036));
#52363=CARTESIAN_POINT('Ctrl Pts',(-0.0293550500899423,0.0107033104702102,
0.00496259135149595));
#52364=CARTESIAN_POINT('Ctrl Pts',(-0.0257443979892688,0.0133708802766567,
0.00397209877924601));
#52365=CARTESIAN_POINT('Ctrl Pts',(-0.027374523625404,0.0117967361445144,
0.00426655328520934));
#52366=CARTESIAN_POINT('Ctrl Pts',(-0.0292152465893807,0.0106790667286594,
0.00503106627065884));
#52367=CARTESIAN_POINT('Ctrl Pts',(-0.0256938523784136,0.0133707634325717,
0.00400194558902871));
#52368=CARTESIAN_POINT('Ctrl Pts',(-0.0272913586865124,0.0117905218792716,
0.00431368624165812));
#52369=CARTESIAN_POINT('Ctrl Pts',(-0.0290984582809993,0.0106592263497628,
0.00508887994392313));
#52370=CARTESIAN_POINT('Ctrl Pts',(-0.0256556496704833,0.0133706744705477,
0.00402450652784909));
#52371=CARTESIAN_POINT('Ctrl Pts',(-0.0272275704451228,0.0117857934129971,
0.00434999678655546));
#52372=CARTESIAN_POINT('Ctrl Pts',(-0.0290082867014547,0.0106441392730587,
0.0051338276680476));
#52373=CARTESIAN_POINT('Ctrl Pts',(-0.0256171358979087,0.0133705828336653,
0.00404725483162211));
#52374=CARTESIAN_POINT('Ctrl Pts',(-0.0271621083758112,0.0117809230482831,
0.00438748456117196));
#52375=CARTESIAN_POINT('Ctrl Pts',(-0.0289150444880619,0.0106286994218181,
0.00518076920054308));
#52376=CARTESIAN_POINT('Ctrl Pts',(-0.0255847661135387,0.0133705076531511,
0.00406637461446268));
#52377=CARTESIAN_POINT('Ctrl Pts',(-0.0271065553024961,0.011776932871555,
0.00441933156444236));
#52378=CARTESIAN_POINT('Ctrl Pts',(-0.0288355855642515,0.0106159367237068,
0.00522084688296197));
#52379=CARTESIAN_POINT('Ctrl Pts',(-0.025563606220307,0.0133704527601798,
0.00407887856220428));
#52380=CARTESIAN_POINT('Ctrl Pts',(-0.0270690596116852,0.0117740106014142,
0.00444114774412889));
#52381=CARTESIAN_POINT('Ctrl Pts',(-0.0287812858755557,0.010606945392152,
0.00524892446387147));
#52382=CARTESIAN_POINT('Ctrl Pts',(-0.0255538335707082,0.0133704327217964,
0.00408464950974319));
#52383=CARTESIAN_POINT('Ctrl Pts',(-0.0270523837722345,0.0117729523163032,
0.00445062705504254));
#52384=CARTESIAN_POINT('Ctrl Pts',(-0.028757478455657,0.0106034018291441,
0.00526077067671198));
#52385=CARTESIAN_POINT('Ctrl Pts',(-0.0255489142526789,0.0133704125322435,
0.00408756242539133));
#52386=CARTESIAN_POINT('Ctrl Pts',(-0.0270426052424206,0.0117718661395984,
0.00445665226233641));
#52387=CARTESIAN_POINT('Ctrl Pts',(-0.0287427442485597,0.0106004647633864,
0.00526909418370154));
#52388=CARTESIAN_POINT('Ctrl Pts',(-0.0255441020276982,0.0133704317568388,
0.00409038141371926));
#52389=CARTESIAN_POINT('Ctrl Pts',(-0.0270383028643863,0.0117729389486516,
0.00445776637193981));
#52390=CARTESIAN_POINT('Ctrl Pts',(-0.0287387840281493,0.010602043307318,
0.00526823762833236));
#52391=CARTESIAN_POINT('Ctrl Pts',(-0.0255360044973167,0.0133698094337739,
0.00409563689201563));
#52392=CARTESIAN_POINT('Ctrl Pts',(-0.026943593979902,0.0117389370272235,
0.00453928205208165));
#52393=CARTESIAN_POINT('Ctrl Pts',(-0.0285576641821581,0.0105285739785202,
0.00541515896656904));
#52394=CARTESIAN_POINT('Ctrl Pts',(-0.0255261811386256,0.0133692422925823,
0.00410186775774673));
#52395=CARTESIAN_POINT('Ctrl Pts',(-0.0268520852953097,0.0117078800431923,
0.00461653960126812));
#52396=CARTESIAN_POINT('Ctrl Pts',(-0.0283856961685775,0.0104635133099934,
0.00555576112810152));
#52397=CARTESIAN_POINT('Ctrl Pts',(-0.0255098110905591,0.0133682485098969,
0.00411229325548317));
#52398=CARTESIAN_POINT('Ctrl Pts',(-0.0266912899161765,0.0116533146508789,
0.00475265080476696));
#52399=CARTESIAN_POINT('Ctrl Pts',(-0.0280845894254988,0.0103533539204758,
0.00580828361020944));
#52400=CARTESIAN_POINT('Ctrl Pts',(-0.0254891046606487,0.013367200844991,
0.00412532497339551));
#52401=CARTESIAN_POINT('Ctrl Pts',(-0.0265144527206189,0.0115954690261533,
0.00490092637256455));
#52402=CARTESIAN_POINT('Ctrl Pts',(-0.02776023610422,0.0102447515300182,
0.00609008394105348));
#52403=CARTESIAN_POINT('Ctrl Pts',(-0.0254637875134938,0.0133661905625418,
0.00414105842990811));
#52404=CARTESIAN_POINT('Ctrl Pts',(-0.0263361898762663,0.0115393372750296,
0.00504907942993433));
#52405=CARTESIAN_POINT('Ctrl Pts',(-0.0274419161564073,0.0101475295589644,
0.00637658056716358));
#52406=CARTESIAN_POINT('Ctrl Pts',(-0.0254304056952004,0.013365133296662,
0.00416160141825757));
#52407=CARTESIAN_POINT('Ctrl Pts',(-0.0261404664461416,0.0114802432167385,
0.00521024801348284));
#52408=CARTESIAN_POINT('Ctrl Pts',(-0.027101818024583,0.0100526087199924,
0.00669107137676832));
#52409=CARTESIAN_POINT('Ctrl Pts',(-0.0253899454488653,0.0133641801502081,
0.00418626208550774));
#52410=CARTESIAN_POINT('Ctrl Pts',(-0.0259508778950532,0.0114265369067877,
0.00536445592173354));
#52411=CARTESIAN_POINT('Ctrl Pts',(-0.0267848099107839,0.00997513282770083,
0.0069935913376081));
#52412=CARTESIAN_POINT('Ctrl Pts',(-0.0253422237865103,0.0133633257894266,
0.00421515806069016));
#52413=CARTESIAN_POINT('Ctrl Pts',(-0.0257665514661048,0.0113780246677331,
0.00551263965393808));
#52414=CARTESIAN_POINT('Ctrl Pts',(-0.0264880543497171,0.00991229104416078,
0.00728329592444431));
#52415=CARTESIAN_POINT('Ctrl Pts',(-0.0252793983582859,0.0133624308307888,
0.00425304141213368));
#52416=CARTESIAN_POINT('Ctrl Pts',(-0.0255571101937992,0.0113268262759728,
0.00567935548445607));
#52417=CARTESIAN_POINT('Ctrl Pts',(-0.026162067728028,0.00985280585796018,
0.00760685205528419));
#52418=CARTESIAN_POINT('Ctrl Pts',(-0.0252036331342202,0.0133616279597208,
0.00429854296104807));
#52419=CARTESIAN_POINT('Ctrl Pts',(-0.0253443255750142,0.0112804205250411,
0.00584661692384335));
#52420=CARTESIAN_POINT('Ctrl Pts',(-0.025845297677816,0.00980768948825244,
0.00792673396362302));
#52421=CARTESIAN_POINT('Ctrl Pts',(-0.0251151268848991,0.0133609229335648,
0.00435154953715688));
#52422=CARTESIAN_POINT('Ctrl Pts',(-0.0251287969092761,0.0112392273586068,
0.00601421883870184));
#52423=CARTESIAN_POINT('Ctrl Pts',(-0.0255374031427373,0.00977586743792922,
0.00824070313324647));
#52424=CARTESIAN_POINT('Ctrl Pts',(-0.0249995654764944,0.0133602086920511,
0.00442063519669263));
#52425=CARTESIAN_POINT('Ctrl Pts',(-0.0248762138213547,0.0111970186426666,
0.00620898163584995));
#52426=CARTESIAN_POINT('Ctrl Pts',(-0.0251890442037446,0.00975199501094654,
0.00859766578095785));
#52427=CARTESIAN_POINT('Ctrl Pts',(-0.0248582632791613,0.013359600841859,
0.00450495748155972));
#52428=CARTESIAN_POINT('Ctrl Pts',(-0.0246042039362115,0.0111604345286657,
0.00641664815771456));
#52429=CARTESIAN_POINT('Ctrl Pts',(-0.0248301609530199,0.00974444741096367,
0.0089658885633592));
#52430=CARTESIAN_POINT('Ctrl Pts',(-0.0246380149274922,0.0133589809712524,
0.00463621895950101));
#52431=CARTESIAN_POINT('Ctrl Pts',(-0.0242247526957397,0.0111221183806697,
0.00670401640032051));
#52432=CARTESIAN_POINT('Ctrl Pts',(-0.0243497852666751,0.00975742460170551,
0.00945556192448081));
#52433=CARTESIAN_POINT('Ctrl Pts',(-0.0243729338683078,0.0133586358239313,
0.00479400285784582));
#52434=CARTESIAN_POINT('Ctrl Pts',(-0.0238222364174371,0.0110991446822809,
0.007006206123228));
#52435=CARTESIAN_POINT('Ctrl Pts',(-0.023864787508101,0.00980148850514733,
0.0099415894121633));
#52436=CARTESIAN_POINT('Ctrl Pts',(-0.0240639991262786,0.0133585753914925,
0.00497773811248542));
#52437=CARTESIAN_POINT('Ctrl Pts',(-0.023398651500273,0.0110923841763263,
0.00732222080231654));
#52438=CARTESIAN_POINT('Ctrl Pts',(-0.0233741410159405,0.00987436526268883,
0.0104191227673781));
#52439=CARTESIAN_POINT('Ctrl Pts',(-0.0237616794738991,0.0133587454597912,
0.00515743938209382));
#52440=CARTESIAN_POINT('Ctrl Pts',(-0.0230144604738983,0.0110993286290909,
0.00760734303674687));
#52441=CARTESIAN_POINT('Ctrl Pts',(-0.0229421337902909,0.00995878657650268,
0.0108259647819836));
#52442=CARTESIAN_POINT('Ctrl Pts',(-0.0233649946146776,0.0133591848020346,
0.00539313616345824));
#52443=CARTESIAN_POINT('Ctrl Pts',(-0.0225386758600217,0.0111213569246464,
0.00795867594547827));
#52444=CARTESIAN_POINT('Ctrl Pts',(-0.02241894455993,0.0100805004122373,
0.0113016788678717));
#52445=CARTESIAN_POINT('Ctrl Pts',(-0.0228780788425745,0.0133600265415265,
0.00568230081805398));
#52446=CARTESIAN_POINT('Ctrl Pts',(-0.0219945592608549,0.0111665834138114,
0.00835711336133469));
#52447=CARTESIAN_POINT('Ctrl Pts',(-0.0218358028786606,0.0102431535003208,
0.0118023917664635));
#52448=CARTESIAN_POINT('Ctrl Pts',(-0.022305766431248,0.0133613156346166,
0.00602199835405312));
#52449=CARTESIAN_POINT('Ctrl Pts',(-0.0213938782142982,0.0112378915781148,
0.00879089397721249));
#52450=CARTESIAN_POINT('Ctrl Pts',(-0.0212055476440137,0.0104431187383345,
0.0123039181617212));
#52451=CARTESIAN_POINT('Ctrl Pts',(-0.0219292577234598,0.0133623030344497,
0.00624536295715626));
#52452=CARTESIAN_POINT('Ctrl Pts',(-0.0210163471587063,0.0112932429550283,
0.00905875420573385));
#52453=CARTESIAN_POINT('Ctrl Pts',(-0.0208154213726988,0.010576673703214,
0.0125909030789934));
#52454=CARTESIAN_POINT('Ctrl Pts',(-0.0217418465582972,0.013362819665371,
0.00635651709279996));
#52455=CARTESIAN_POINT('Ctrl Pts',(-0.0208314744349912,0.0113223146764728,
0.00918856807479045));
#52456=CARTESIAN_POINT('Ctrl Pts',(-0.0206254586057132,0.010643066208173,
0.0127253928900171));
#52457=CARTESIAN_POINT('',(-0.0217848380421749,0.0133386308183493,0.00635794497981714));
#52458=CARTESIAN_POINT('Ctrl Pts',(-0.0311805491196909,0.0110755203513828,
0.00410667728630412));
#52459=CARTESIAN_POINT('Ctrl Pts',(-0.0303628462213495,0.0110536005240181,
0.00427642982102741));
#52460=CARTESIAN_POINT('Ctrl Pts',(-0.0291450767836391,0.0111156395935359,
0.00451528869049828));
#52461=CARTESIAN_POINT('Ctrl Pts',(-0.0275504601453372,0.0113532710676122,
0.00486779796847178));
#52462=CARTESIAN_POINT('Ctrl Pts',(-0.0259696456997476,0.0118045993808991,
0.00517760956883624));
#52463=CARTESIAN_POINT('Ctrl Pts',(-0.0240886530202461,0.0125793024532316,
0.00570384378960105));
#52464=CARTESIAN_POINT('Ctrl Pts',(-0.0225643752139947,0.0131235232054828,
0.00613182294147269));
#52465=CARTESIAN_POINT('Ctrl Pts',(-0.0217848380421749,0.0133386308183493,
0.00635794497981714));
#52466=CARTESIAN_POINT('',(-0.0227510611416183,0.0133301029619171,0.00578783038319825));
#52467=CARTESIAN_POINT('Ctrl Pts',(-0.0227510611416183,0.0133301029619171,
0.00578783038319825));
#52468=CARTESIAN_POINT('Ctrl Pts',(-0.0225988241462555,0.0133314270627633,
0.00587773671841089));
#52469=CARTESIAN_POINT('Ctrl Pts',(-0.0224468599320209,0.0133327705039863,
0.00596743869532409));
#52470=CARTESIAN_POINT('Ctrl Pts',(-0.0222953888501995,0.0133341234933048,
0.00605680312827367));
#52471=CARTESIAN_POINT('Ctrl Pts',(-0.0221243986305164,0.0133356508339562,
0.00615768340085212));
#52472=CARTESIAN_POINT('Ctrl Pts',(-0.0219540318556272,0.0133371902973775,
0.00625813645800992));
#52473=CARTESIAN_POINT('Ctrl Pts',(-0.0217847944705363,0.0133387336320324,
0.00635785581245878));
#52474=CARTESIAN_POINT('',(-0.0264065477674619,0.0133196469578813,0.0036268963164667));
#52475=CARTESIAN_POINT('Ctrl Pts',(-0.0264065477674619,0.0133196469578813,
0.00362689631646671));
#52476=CARTESIAN_POINT('Ctrl Pts',(-0.026394716629658,0.0133195174636387,
0.00363389128041229));
#52477=CARTESIAN_POINT('Ctrl Pts',(-0.0263834986769066,0.013319395206925,
0.00364052343157509));
#52478=CARTESIAN_POINT('Ctrl Pts',(-0.0263727080949494,0.0133192784627222,
0.00364690234370207));
#52479=CARTESIAN_POINT('Ctrl Pts',(-0.0263512398831163,0.0133190461963545,
0.0036595933957093));
#52480=CARTESIAN_POINT('Ctrl Pts',(-0.0263314663061818,0.0133188357788058,
0.00367128027334653));
#52481=CARTESIAN_POINT('Ctrl Pts',(-0.0263118834379465,0.0133186332101986,
0.00368285016275895));
#52482=CARTESIAN_POINT('Ctrl Pts',(-0.0262971705286196,0.0133184810172965,
0.00369154279816876));
#52483=CARTESIAN_POINT('Ctrl Pts',(-0.0262825684258451,0.0133183333998923,
0.00370016757369084));
#52484=CARTESIAN_POINT('Ctrl Pts',(-0.0262751672873967,0.0133182556390686,
0.00370454166801996));
#52485=CARTESIAN_POINT('Ctrl Pts',(-0.0262677661489483,0.0133181778782449,
0.00370891576234908));
#52486=CARTESIAN_POINT('Ctrl Pts',(-0.0262675658719951,0.0133181696127009,
0.00370903898435915));
#52487=CARTESIAN_POINT('Ctrl Pts',(-0.0262455282347752,0.0133179638674093,
0.00372204245026586));
#52488=CARTESIAN_POINT('Ctrl Pts',(-0.0262418372101996,0.0133179294076838,
0.00372422036579057));
#52489=CARTESIAN_POINT('Ctrl Pts',(-0.026237536410453,0.0133178894691057,
0.00372675793654771));
#52490=CARTESIAN_POINT('Ctrl Pts',(-0.0262327486899822,0.013317845278354,
0.00372958264011147));
#52491=CARTESIAN_POINT('Ctrl Pts',(-0.0262089508389711,0.0133176256237332,
0.00374362311615229));
#52492=CARTESIAN_POINT('Ctrl Pts',(-0.0261730618794819,0.0133173003171878,
0.0037647942828713));
#52493=CARTESIAN_POINT('Ctrl Pts',(-0.0261404843237304,0.0133170230323306,
0.00378400090645341));
#52494=CARTESIAN_POINT('Ctrl Pts',(-0.0261226794117806,0.0133168714852807,
0.00379449807954832));
#52495=CARTESIAN_POINT('Ctrl Pts',(-0.0261058493888371,0.0133167338782244,
0.00380441680035033));
#52496=CARTESIAN_POINT('Ctrl Pts',(-0.0260893950595296,0.0133166044095186,
0.00381411086136281));
#52497=CARTESIAN_POINT('Ctrl Pts',(-0.0260696860942685,0.0133164493321419,
0.00382572238974317));
#52498=CARTESIAN_POINT('Ctrl Pts',(-0.0260505173670805,0.0133163059437924,
0.00383701085155254));
#52499=CARTESIAN_POINT('Ctrl Pts',(-0.0260308178878044,0.0133161638331711,
0.00384860916443173));
#52500=CARTESIAN_POINT('Ctrl Pts',(-0.0260259891081691,0.0133161289987034,
0.00385145216836346));
#52501=CARTESIAN_POINT('Ctrl Pts',(-0.0260211296759531,0.0133160942559615,
0.00385431305907611));
#52502=CARTESIAN_POINT('Ctrl Pts',(-0.0260162408533954,0.0133160596206651,
0.00385719109461294));
#52503=CARTESIAN_POINT('Ctrl Pts',(-0.0259921529245199,0.0133158889675996,
0.00387137158786942));
#52504=CARTESIAN_POINT('Ctrl Pts',(-0.0259673511316601,0.0133157209193171,
0.00388596851921629));
#52505=CARTESIAN_POINT('Ctrl Pts',(-0.0259419782668339,0.0133155572563812,
0.00390089801887217));
#52506=CARTESIAN_POINT('Ctrl Pts',(-0.0259172996240843,0.0133153980713955,
0.00391541903535815));
#52507=CARTESIAN_POINT('Ctrl Pts',(-0.02589208018466,0.0133152430298302,
0.00393025499756256));
#52508=CARTESIAN_POINT('Ctrl Pts',(-0.0258664910751612,0.013315094022236,
0.00394530533415525));
#52509=CARTESIAN_POINT('Ctrl Pts',(-0.0258437895321223,0.0133149618291905,
0.00395865733704245));
#52510=CARTESIAN_POINT('Ctrl Pts',(-0.0258207972354934,0.0133148343859008,
0.00397217795015615));
#52511=CARTESIAN_POINT('Ctrl Pts',(-0.0257976307872261,0.0133147128628802,
0.00398579869902889));
#52512=CARTESIAN_POINT('Ctrl Pts',(-0.0257815941249314,0.0133146287402033,
0.00399522747927838));
#52513=CARTESIAN_POINT('Ctrl Pts',(-0.0257659133899357,0.0133146836001378,
0.00400433856955475));
#52514=CARTESIAN_POINT('Ctrl Pts',(-0.0257505285264267,0.0133148550678093,
0.00401318621280172));
#52515=CARTESIAN_POINT('Ctrl Pts',(-0.0257369531148523,0.013315006368743,
0.00402099326279412));
#52516=CARTESIAN_POINT('Ctrl Pts',(-0.025723607921997,0.0133152484333549,
0.00402859528929107));
#52517=CARTESIAN_POINT('Ctrl Pts',(-0.0257104486655114,0.01331556493994,
0.00403603178733425));
#52518=CARTESIAN_POINT('Ctrl Pts',(-0.02569662428812,0.0133158974440206,
0.00404384415542149));
#52519=CARTESIAN_POINT('Ctrl Pts',(-0.0256830052830809,0.0133163121828292,
0.00405147368002277));
#52520=CARTESIAN_POINT('Ctrl Pts',(-0.0256695407622072,0.0133167925088795,
0.0040589638258519));
#52521=CARTESIAN_POINT('Ctrl Pts',(-0.0256555101539921,0.013317293029224,
0.00406676887904234));
#52522=CARTESIAN_POINT('Ctrl Pts',(-0.0256416470042577,0.0133178645117327,
0.00407442295752445));
#52523=CARTESIAN_POINT('Ctrl Pts',(-0.0256278835755066,0.013318478517641,
0.004081988529265));
#52524=CARTESIAN_POINT('Ctrl Pts',(-0.0256208342766697,0.0133187929967736,
0.00408586343406058));
#52525=CARTESIAN_POINT('Ctrl Pts',(-0.0256138113920498,0.0133191187798247,
0.00408971485050543));
#52526=CARTESIAN_POINT('Ctrl Pts',(-0.025606829280161,0.0133194621940564,
0.00409352939535447));
#52527=CARTESIAN_POINT('Ctrl Pts',(-0.0256033059204389,0.0133196354900292,
0.00409545431633727));
#52528=CARTESIAN_POINT('Ctrl Pts',(-0.025599720549853,0.0133197857610566,
0.00409743396679169));
#52529=CARTESIAN_POINT('Ctrl Pts',(-0.0255962542995072,0.0133199819038571,
0.00409930787760123));
#52530=CARTESIAN_POINT('Ctrl Pts',(-0.0255927708341416,0.0133201790207944,
0.00410119109512799));
#52531=CARTESIAN_POINT('Ctrl Pts',(-0.0255882443720757,0.0133199524295486,
0.00410401805778399));
#52532=CARTESIAN_POINT('Ctrl Pts',(-0.0255828256013243,0.0133193965594662,
0.00410762851133424));
#52533=CARTESIAN_POINT('Ctrl Pts',(-0.0255773850046021,0.0133188384504251,
0.00411125350723321));
#52534=CARTESIAN_POINT('Ctrl Pts',(-0.0255722675677563,0.0133184406762622,
0.0041145654139126));
#52535=CARTESIAN_POINT('Ctrl Pts',(-0.0255670336542669,0.0133180207611486,
0.00411796495422484));
#52536=CARTESIAN_POINT('Ctrl Pts',(-0.0255617837093089,0.0133175995598357,
0.00412137490732359));
#52537=CARTESIAN_POINT('Ctrl Pts',(-0.0255564191556313,0.0133171571293206,
0.00412487069938319));
#52538=CARTESIAN_POINT('Ctrl Pts',(-0.0255511062565089,0.0133167559324299,
0.00412830573725567));
#52539=CARTESIAN_POINT('Ctrl Pts',(-0.0255404526285013,0.0133159514371192,
0.00413519380624443));
#52540=CARTESIAN_POINT('Ctrl Pts',(-0.0255300037364794,0.013315311428736,
0.00414184032636662));
#52541=CARTESIAN_POINT('Ctrl Pts',(-0.0255196915273417,0.0133147951582003,
0.00414831527807117));
#52542=CARTESIAN_POINT('Ctrl Pts',(-0.0255093777785549,0.0133142788105836,
0.00415479119650885));
#52543=CARTESIAN_POINT('Ctrl Pts',(-0.0254992007062769,0.0133138863721156,
0.00416109542777311));
#52544=CARTESIAN_POINT('Ctrl Pts',(-0.0254892398687713,0.0133135951681441,
0.00416719731466131));
#52545=CARTESIAN_POINT('Ctrl Pts',(-0.025479317298874,0.0133133050829218,
0.00417327575928203));
#52546=CARTESIAN_POINT('Ctrl Pts',(-0.0254696091039602,0.0133131154472376,
0.00417915354185311));
#52547=CARTESIAN_POINT('Ctrl Pts',(-0.0254600820614871,0.0133129889108621,
0.00418487821075715));
#52548=CARTESIAN_POINT('Ctrl Pts',(-0.0254412823347847,0.0133127392164493,
0.00419617470819175));
#52549=CARTESIAN_POINT('Ctrl Pts',(-0.0254231884885536,0.0133127349632696,
0.00420687487902349));
#52550=CARTESIAN_POINT('Ctrl Pts',(-0.0254052540728127,0.0133128084471708,
0.00421742822975724));
#52551=CARTESIAN_POINT('Ctrl Pts',(-0.0253878400671775,0.0133128797987603,
0.00422767534969703));
#52552=CARTESIAN_POINT('Ctrl Pts',(-0.0253705767865013,0.0133130248895279,
0.00423778347418303));
#52553=CARTESIAN_POINT('Ctrl Pts',(-0.0253532413158221,0.0133131683409094,
0.00424794200591349));
#52554=CARTESIAN_POINT('Ctrl Pts',(-0.0253365992332474,0.0133133060544899,
0.00425769421437813));
#52555=CARTESIAN_POINT('Ctrl Pts',(-0.0253198883280054,0.0133134423171085,
0.00426749419583593));
#52556=CARTESIAN_POINT('Ctrl Pts',(-0.0253030695365654,0.0133135281161507,
0.00427740269087294));
#52557=CARTESIAN_POINT('Ctrl Pts',(-0.025294225752135,0.0133135732316535,
0.00428261285085673));
#52558=CARTESIAN_POINT('Ctrl Pts',(-0.0252853528909199,0.0133136043649565,
0.00428785259469544));
#52559=CARTESIAN_POINT('Ctrl Pts',(-0.0252764301019966,0.0133136158059306,
0.00429313878769495));
#52560=CARTESIAN_POINT('Ctrl Pts',(-0.0252535722047203,0.0133136451147725,
0.00430668065869561));
#52561=CARTESIAN_POINT('Ctrl Pts',(-0.0252306241532069,0.0133137059755598,
0.00432025962806135));
#52562=CARTESIAN_POINT('Ctrl Pts',(-0.0252074780937085,0.0133137741353841,
0.00433395707742505));
#52563=CARTESIAN_POINT('Ctrl Pts',(-0.0251772875882765,0.0133138630394823,
0.0043518233116083));
#52564=CARTESIAN_POINT('Ctrl Pts',(-0.0251467570318961,0.0133139639258754,
0.00436989333476208));
#52565=CARTESIAN_POINT('Ctrl Pts',(-0.0251158775334444,0.0133140652437999,
0.0043881799678752));
#52566=CARTESIAN_POINT('Ctrl Pts',(-0.0250865312992789,0.0133141615309705,
0.00440555861210011));
#52567=CARTESIAN_POINT('Ctrl Pts',(-0.0250568693955269,0.0133142579509085,
0.00442313337980284));
#52568=CARTESIAN_POINT('Ctrl Pts',(-0.0250268673250634,0.0133143510110433,
0.00444092051686331));
#52569=CARTESIAN_POINT('Ctrl Pts',(-0.0249703190496052,0.0133145264119425,
0.00447444593396187));
#52570=CARTESIAN_POINT('Ctrl Pts',(-0.0249125598664124,0.0133146903323235,
0.00450872724959347));
#52571=CARTESIAN_POINT('Ctrl Pts',(-0.0248539896070711,0.0133148787353483,
0.00454349276756054));
#52572=CARTESIAN_POINT('Ctrl Pts',(-0.0247974986888213,0.013315060449754,
0.00457702405213189));
#52573=CARTESIAN_POINT('Ctrl Pts',(-0.0247402504940931,0.0133152640973943,
0.00461100801798857));
#52574=CARTESIAN_POINT('Ctrl Pts',(-0.024682654870725,0.0133155440084415,
0.00464515093357176));
#52575=CARTESIAN_POINT('Ctrl Pts',(-0.0245787095346326,0.0133160491761292,
0.00470677014398967));
#52576=CARTESIAN_POINT('Ctrl Pts',(-0.0244727850114969,0.0133166393006272,
0.00476954594658457));
#52577=CARTESIAN_POINT('Ctrl Pts',(-0.024358237683565,0.0133173697130724,
0.00483738766158962));
#52578=CARTESIAN_POINT('Ctrl Pts',(-0.0242573494148497,0.0133180130283586,
0.0048971396723708));
#52579=CARTESIAN_POINT('Ctrl Pts',(-0.024149732020381,0.0133187647412866,
0.00496084760167406));
#52580=CARTESIAN_POINT('Ctrl Pts',(-0.0240537247169841,0.013319470739504,
0.00501766384229477));
#52581=CARTESIAN_POINT('Ctrl Pts',(-0.0240407264818175,0.0133195663231787,
0.00502535607851787));
#52582=CARTESIAN_POINT('Ctrl Pts',(-0.0240279382978251,0.0133196609048211,
0.00503292375035051));
#52583=CARTESIAN_POINT('Ctrl Pts',(-0.0240154037824746,0.0133197540155003,
0.00504034113731551));
#52584=CARTESIAN_POINT('Ctrl Pts',(-0.0239174314892982,0.0133204817872973,
0.00509831692576976));
#52585=CARTESIAN_POINT('Ctrl Pts',(-0.0238351585444195,0.0133211275768285,
0.00514698203734017));
#52586=CARTESIAN_POINT('Ctrl Pts',(-0.0237503321966176,0.0133217980683467,
0.00519715584830999));
#52587=CARTESIAN_POINT('Ctrl Pts',(-0.0237441464273266,0.0133218469624221,
0.00520081465983675));
#52588=CARTESIAN_POINT('Ctrl Pts',(-0.0237379476838069,0.0133218960232413,
0.00520448110756548));
#52589=CARTESIAN_POINT('Ctrl Pts',(-0.0237317291711661,0.0133219453089548,
0.00520815920566391));
#52590=CARTESIAN_POINT('Ctrl Pts',(-0.0236402352964382,0.0133226704567771,
0.00526227559427542));
#52591=CARTESIAN_POINT('Ctrl Pts',(-0.0235443118153809,0.0133234371794813,
0.0053190105854227));
#52592=CARTESIAN_POINT('Ctrl Pts',(-0.0234494523212224,0.0133242089308042,
0.0053751038212117));
#52593=CARTESIAN_POINT('Ctrl Pts',(-0.0232597333329052,0.01332575243345,
0.00548729029278969));
#52594=CARTESIAN_POINT('Ctrl Pts',(-0.0230742704576996,0.0133273148826671,
0.0055969100218233));
#52595=CARTESIAN_POINT('Ctrl Pts',(-0.0228890601614922,0.013328908902742,
0.00570632078071611));
#52596=CARTESIAN_POINT('Ctrl Pts',(-0.0228819374396055,0.0133289702047425,
0.00571052844315698));
#52597=CARTESIAN_POINT('Ctrl Pts',(-0.0228748151351252,0.0133290315567097,
0.00571473576617383));
#52598=CARTESIAN_POINT('Ctrl Pts',(-0.0228676932904643,0.0133290929561784,
0.00571894272488699));
#52599=CARTESIAN_POINT('Ctrl Pts',(-0.0228288007996344,0.0133294282595149,
0.00574191698379919));
#52600=CARTESIAN_POINT('Ctrl Pts',(-0.022789922488709,0.0133297649870326,
0.00576488010001121));
#52601=CARTESIAN_POINT('Ctrl Pts',(-0.0227510611416183,0.0133301029619171,
0.00578783038319825));
#52602=CARTESIAN_POINT('',(-0.0307012608623869,0.0133637168977234,0.00107862162231056));
#52603=CARTESIAN_POINT('Ctrl Pts',(-0.0307012608623869,0.0133637168977234,
0.00107862162231056));
#52604=CARTESIAN_POINT('Ctrl Pts',(-0.0303353115612717,0.0133609145128637,
0.00129643444327742));
#52605=CARTESIAN_POINT('Ctrl Pts',(-0.029992089042177,0.0133579810772048,
0.00150062793971989));
#52606=CARTESIAN_POINT('Ctrl Pts',(-0.0296705263034281,0.0133550150323022,
0.00169181816446555));
#52607=CARTESIAN_POINT('Ctrl Pts',(-0.0294963157598973,0.0133534081412282,
0.00179539780525453));
#52608=CARTESIAN_POINT('Ctrl Pts',(-0.0293284943915401,0.0133517923054471,
0.00189514229389304));
#52609=CARTESIAN_POINT('Ctrl Pts',(-0.0291673512431136,0.0133501910488438,
0.00199087949557486));
#52610=CARTESIAN_POINT('Ctrl Pts',(-0.0290793930908137,0.0133493170211637,
0.00204313655675635));
#52611=CARTESIAN_POINT('Ctrl Pts',(-0.0289934229671365,0.0133484473481551,
0.00209420070809991));
#52612=CARTESIAN_POINT('Ctrl Pts',(-0.0289094017947271,0.013347585513257,
0.00214409491897803));
#52613=CARTESIAN_POINT('Ctrl Pts',(-0.0288277133008652,0.0133467476054682,
0.00219260391762897));
#52614=CARTESIAN_POINT('Ctrl Pts',(-0.0287479234814482,0.0133459165378698,
0.00223997497994222));
#52615=CARTESIAN_POINT('Ctrl Pts',(-0.0286699811757669,0.0133450946198445,
0.00228623902273471));
#52616=CARTESIAN_POINT('Ctrl Pts',(-0.0284956456525509,0.0133432562150435,
0.00238971897544866));
#52617=CARTESIAN_POINT('Ctrl Pts',(-0.0283305220174397,0.0133414637385238,
0.00248767895134269));
#52618=CARTESIAN_POINT('Ctrl Pts',(-0.0281744805302891,0.0133397409158217,
0.00258020890118065));
#52619=CARTESIAN_POINT('Ctrl Pts',(-0.0279964830986621,0.0133377756819488,
0.00268575835293535));
#52620=CARTESIAN_POINT('Ctrl Pts',(-0.0278302789703917,0.0133359010791335,
0.00278425701312616));
#52621=CARTESIAN_POINT('Ctrl Pts',(-0.0276761673782987,0.0133341465135724,
0.00287555202195714));
#52622=CARTESIAN_POINT('Ctrl Pts',(-0.0276397484012646,0.0133337318823172,
0.00289712645892705));
#52623=CARTESIAN_POINT('Ctrl Pts',(-0.0276040084430913,0.0133333239399807,
0.00291829640020815));
#52624=CARTESIAN_POINT('Ctrl Pts',(-0.0275689538164303,0.0133329230132978,
0.00293905844958548));
#52625=CARTESIAN_POINT('Ctrl Pts',(-0.0275193315674378,0.0133323554738435,
0.00296844856672347));
#52626=CARTESIAN_POINT('Ctrl Pts',(-0.0274710620702214,0.013331801765515,
0.00299703350333233));
#52627=CARTESIAN_POINT('Ctrl Pts',(-0.0274241340969779,0.0133312624917841,
0.00302482064625548));
#52628=CARTESIAN_POINT('Ctrl Pts',(-0.0273341082830727,0.0133302279583666,
0.00307812702164006));
#52629=CARTESIAN_POINT('Ctrl Pts',(-0.02724901697524,0.0133292465851678,
0.00312849901069747));
#52630=CARTESIAN_POINT('Ctrl Pts',(-0.0271689222567074,0.0133283225186183,
0.00317590502138782));
#52631=CARTESIAN_POINT('Ctrl Pts',(-0.0271344513707912,0.0133279248220762,
0.00319630745510868));
#52632=CARTESIAN_POINT('Ctrl Pts',(-0.027100906699519,0.0133275377318371,
0.0032161600660394));
#52633=CARTESIAN_POINT('Ctrl Pts',(-0.0270682927695371,0.0133271615071192,
0.00323546053550353));
#52634=CARTESIAN_POINT('Ctrl Pts',(-0.0270127281719848,0.0133265205302405,
0.00326834289034221));
#52635=CARTESIAN_POINT('Ctrl Pts',(-0.0269598553070662,0.0133259110090293,
0.00329962843520989));
#52636=CARTESIAN_POINT('Ctrl Pts',(-0.0269096234083803,0.0133253331845922,
0.00332934846738256));
#52637=CARTESIAN_POINT('Ctrl Pts',(-0.0268261533736523,0.0133243730173061,
0.00337873406065028));
#52638=CARTESIAN_POINT('Ctrl Pts',(-0.0267499648859122,0.0133235003201201,
0.00342380352386417));
#52639=CARTESIAN_POINT('Ctrl Pts',(-0.0266808066024393,0.013322714655098,
0.00346470917922637));
#52640=CARTESIAN_POINT('Ctrl Pts',(-0.026668629363042,0.0133225763169181,
0.00347191175761667));
#52641=CARTESIAN_POINT('Ctrl Pts',(-0.0266566706260414,0.0133224406803111,
0.00347898491250738));
#52642=CARTESIAN_POINT('Ctrl Pts',(-0.026644935364075,0.0133223077955545,
0.00348592572439474));
#52643=CARTESIAN_POINT('Ctrl Pts',(-0.0265959129162677,0.0133217526877038,
0.00351492001437869));
#52644=CARTESIAN_POINT('Ctrl Pts',(-0.0265507866300319,0.0133212455758331,
0.00354160707007658));
#52645=CARTESIAN_POINT('Ctrl Pts',(-0.0265099328376447,0.0133207900375879,
0.00356576558784225));
#52646=CARTESIAN_POINT('Ctrl Pts',(-0.02647159868028,0.0133203625944116,
0.00358843414240255));
#52647=CARTESIAN_POINT('Ctrl Pts',(-0.0264370276338154,0.0133199805663026,
0.00360887560115242));
#52648=CARTESIAN_POINT('Ctrl Pts',(-0.0264065477674619,0.0133196469578813,
0.00362689631646671));
#52649=CARTESIAN_POINT('Origin',(-0.0350444526050681,0.0256340492967854,
0.00853352794652652));
#52650=CARTESIAN_POINT('Ctrl Pts',(-0.0346818054102186,0.0119846858024896,
0.00232257533643425));
#52651=CARTESIAN_POINT('Ctrl Pts',(-0.0325963194414617,0.0123976569665182,
0.00153734729870167));
#52652=CARTESIAN_POINT('Ctrl Pts',(-0.03061725147117,0.0133985938507509,
0.00107061716078679));
#52653=CARTESIAN_POINT('Ctrl Pts',(-0.0354361330509732,0.0121509732395146,
0.00193216893213736));
#52654=CARTESIAN_POINT('Ctrl Pts',(-0.0330226689375074,0.0124110180713967,
0.00129825859323519));
#52655=CARTESIAN_POINT('Ctrl Pts',(-0.0307425222934407,0.0133986155780547,
0.000998140594337429));
#52656=CARTESIAN_POINT('Ctrl Pts',(-0.036011215516007,0.0123500627020912,
0.00135104585411375));
#52657=CARTESIAN_POINT('Ctrl Pts',(-0.033395569122503,0.0124397950591077,
0.000973263036901243));
#52658=CARTESIAN_POINT('Ctrl Pts',(-0.0309408025410812,0.0133986581242847,
0.000852236643677883));
#52659=CARTESIAN_POINT('Ctrl Pts',(-0.0363091803430268,0.0124790671617841,
0.000573007463839057));
#52660=CARTESIAN_POINT('Ctrl Pts',(-0.0336656182136692,0.0124888897140569,
0.000449578966366591));
#52661=CARTESIAN_POINT('Ctrl Pts',(-0.0311818867874813,0.0133987267804568,
0.000433853907110055));
#52662=CARTESIAN_POINT('Ctrl Pts',(-0.0363699702965885,0.0125113195748914,
1.02558394175085E-6));
#52663=CARTESIAN_POINT('Ctrl Pts',(-0.0337391428303402,0.0125064594535196,
5.56793826959371E-7));
#52664=CARTESIAN_POINT('Ctrl Pts',(-0.0312650822031905,0.0133987511234855,
1.37775683656485E-7));
#52665=CARTESIAN_POINT('Ctrl Pts',(-0.0363114929505171,0.0124788561197549,
-0.000573062348264479));
#52666=CARTESIAN_POINT('Ctrl Pts',(-0.0336665459476314,0.0124883464178191,
-0.00044988160607198));
#52667=CARTESIAN_POINT('Ctrl Pts',(-0.0311815545155191,0.0133987260406928,
-0.000434839939525983));
#52668=CARTESIAN_POINT('Ctrl Pts',(-0.0360173256313817,0.0123499454800039,
-0.00134821109832071));
#52669=CARTESIAN_POINT('Ctrl Pts',(-0.0333986737828021,0.0124387380183363,
-0.000971258174768614));
#52670=CARTESIAN_POINT('Ctrl Pts',(-0.0309411737711407,0.0133986566920038,
-0.000851300456162731));
#52671=CARTESIAN_POINT('Ctrl Pts',(-0.0354494076621593,0.0121512055067501,
-0.0019289935218175));
#52672=CARTESIAN_POINT('Ctrl Pts',(-0.0330293516321701,0.0124093950736726,
-0.00129574422396878));
#52673=CARTESIAN_POINT('Ctrl Pts',(-0.0307431403215359,0.0133986133925361,
-0.000997812178750743));
#52674=CARTESIAN_POINT('Ctrl Pts',(-0.0346932848386117,0.0119831034613695,
-0.00232183549083736));
#52675=CARTESIAN_POINT('Ctrl Pts',(-0.0326018426404496,0.0123955015963908,
-0.00153607898158788));
#52676=CARTESIAN_POINT('Ctrl Pts',(-0.0306171897688803,0.0133985909035257,
-0.00107065436122431));
#52677=CARTESIAN_POINT('',(-0.0307004248295923,0.0133627434399838,-0.00107761006352919));
#52678=CARTESIAN_POINT('Ctrl Pts',(-0.0307017856734144,0.0133639656227132,
-0.00107885621208017));
#52679=CARTESIAN_POINT('Ctrl Pts',(-0.0309758135796404,0.0133799891925163,
-0.000888980768471492));
#52680=CARTESIAN_POINT('Ctrl Pts',(-0.0311660487382375,0.0133854863143006,
-0.000598005060207441));
#52681=CARTESIAN_POINT('Ctrl Pts',(-0.031235681726719,0.0133876603108539,
-0.00028351370406858));
#52682=CARTESIAN_POINT('Ctrl Pts',(-0.0312563008708948,0.0133883040567185,
-0.000190389126828655));
#52683=CARTESIAN_POINT('Ctrl Pts',(-0.0312666928517517,0.0133886046897988,
-9.52395766237666E-5));
#52684=CARTESIAN_POINT('Ctrl Pts',(-0.031266718265333,0.0133885997848049,
-1.27307345280826E-7));
#52685=CARTESIAN_POINT('Ctrl Pts',(-0.0312668046408911,0.0133885831137349,
0.000323139817202629));
#52686=CARTESIAN_POINT('Ctrl Pts',(-0.0311434100165953,0.0133858216570961,
0.000646644017152718));
#52687=CARTESIAN_POINT('Ctrl Pts',(-0.0309186432993367,0.0133753622687773,
0.000890224316156055));
#52688=CARTESIAN_POINT('Ctrl Pts',(-0.0308539464933894,0.0133723516405818,
0.000960336419626767));
#52689=CARTESIAN_POINT('Ctrl Pts',(-0.0307811557550656,0.0133686447732898,
0.00102384151068166));
#52690=CARTESIAN_POINT('Ctrl Pts',(-0.0307016309076775,0.0133640088280151,
0.00107891472440616));
#52691=CARTESIAN_POINT('Origin',(-0.0350471488028758,0.025630288756216,
-0.00853808901214505));
#52692=CARTESIAN_POINT('Ctrl Pts',(-0.0347727610542622,0.012000956525018,
-0.00227981334747211));
#52693=CARTESIAN_POINT('Ctrl Pts',(-0.0326642925703876,0.01239375001385,
-0.00151682761576582));
#52694=CARTESIAN_POINT('Ctrl Pts',(-0.03066311424583,0.0133825300884908,
-0.00106998024085706));
#52695=CARTESIAN_POINT('Ctrl Pts',(-0.0345175998045572,0.0119430361337218,
-0.00241714021238289));
#52696=CARTESIAN_POINT('Ctrl Pts',(-0.0323553515124146,0.0123566043453443,
-0.00167688730984057));
#52697=CARTESIAN_POINT('Ctrl Pts',(-0.0303095288998628,0.0133818938394319,
-0.00127859035195531));
#52698=CARTESIAN_POINT('Ctrl Pts',(-0.0341371660549221,0.0118489399475177,
-0.00262427032416602));
#52699=CARTESIAN_POINT('Ctrl Pts',(-0.0318999712760361,0.0122981422085741,
-0.00191169889138664));
#52700=CARTESIAN_POINT('Ctrl Pts',(-0.029794006492062,0.0133808935020843,
-0.0015827147044274));
#52701=CARTESIAN_POINT('Ctrl Pts',(-0.03359953982734,0.0117040686094275,
-0.0029149026918325));
#52702=CARTESIAN_POINT('Ctrl Pts',(-0.0312857444835857,0.0122156780731898,
-0.0022266513258499));
#52703=CARTESIAN_POINT('Ctrl Pts',(-0.0291240247977924,0.0133794825587464,
-0.00197790333209557));
#52704=CARTESIAN_POINT('Ctrl Pts',(-0.0331700961547601,0.0115849838518695,
-0.00314276868365366));
#52705=CARTESIAN_POINT('Ctrl Pts',(-0.0308143431151271,0.012152185224641,
-0.00246736253434012));
#52706=CARTESIAN_POINT('Ctrl Pts',(-0.0286267867573773,0.0133783959197543,
-0.00227116412235461));
#52707=CARTESIAN_POINT('Ctrl Pts',(-0.0327013830619387,0.0114548347231496,
-0.0033840386214771));
#52708=CARTESIAN_POINT('Ctrl Pts',(-0.0303243200167066,0.0120877808095269,
-0.00271670426744098));
#52709=CARTESIAN_POINT('Ctrl Pts',(-0.0281311992831569,0.0133772919708067,
-0.002563413094503));
#52710=CARTESIAN_POINT('Ctrl Pts',(-0.0322633022287014,0.0113362370202907,
-0.00360133811397268));
#52711=CARTESIAN_POINT('Ctrl Pts',(-0.0298917430076046,0.0120338445178328,
-0.00293676226773174));
#52712=CARTESIAN_POINT('Ctrl Pts',(-0.0277161181765403,0.0133763644965302,
-0.00280816048294128));
#52713=CARTESIAN_POINT('Ctrl Pts',(-0.0318718490579452,0.0112346016841242,
-0.00379002559821603));
#52714=CARTESIAN_POINT('Ctrl Pts',(-0.0295242954891501,0.0119908397586535,
-0.00312456116268488));
#52715=CARTESIAN_POINT('Ctrl Pts',(-0.0273809764418348,0.013375621969192,
-0.00300576632589705));
#52716=CARTESIAN_POINT('Ctrl Pts',(-0.0315526756063215,0.0111545881961619,
-0.00394133469003171));
#52717=CARTESIAN_POINT('Ctrl Pts',(-0.0292351036521467,0.0119586531268908,
-0.00327316193381772));
#52718=CARTESIAN_POINT('Ctrl Pts',(-0.0271270696533341,0.0133750642031843,
-0.00315547587947468));
#52719=CARTESIAN_POINT('Ctrl Pts',(-0.0312014210942059,0.0110702650311837,
-0.00410563573794732));
#52720=CARTESIAN_POINT('Ctrl Pts',(-0.0289286457521131,0.0119264976660814,
-0.00343191460904337));
#52721=CARTESIAN_POINT('Ctrl Pts',(-0.0268695127905437,0.0133745044065779,
-0.00330734508306625));
#52722=CARTESIAN_POINT('Ctrl Pts',(-0.030874392335899,0.0109957669425451,
-0.00425734882219583));
#52723=CARTESIAN_POINT('Ctrl Pts',(-0.0286546244642002,0.0118996312458295,
-0.00357549439591694));
#52724=CARTESIAN_POINT('Ctrl Pts',(-0.0266506540595016,0.0133740340157121,
-0.00343640952528322));
#52725=CARTESIAN_POINT('Ctrl Pts',(-0.0305849371878325,0.0109329649976957,
-0.00439163244392445));
#52726=CARTESIAN_POINT('Ctrl Pts',(-0.0284201388623915,0.0118779356122285,
-0.00369985556253239));
#52727=CARTESIAN_POINT('Ctrl Pts',(-0.0264718895472516,0.0133736521617784,
-0.00354184514292115));
#52728=CARTESIAN_POINT('Ctrl Pts',(-0.0303517903493002,0.0108841186312876,
-0.00450011332417866));
#52729=CARTESIAN_POINT('Ctrl Pts',(-0.0282355790180237,0.0118615266852309,
-0.00379864860220248));
#52730=CARTESIAN_POINT('Ctrl Pts',(-0.0263358824933711,0.0133733622256437,
-0.00362207257248992));
#52731=CARTESIAN_POINT('Ctrl Pts',(-0.0300997675905012,0.0108332970063754,
-0.00461811904366943));
#52732=CARTESIAN_POINT('Ctrl Pts',(-0.0280408014590061,0.0118449004444461,
-0.00390403183868317));
#52733=CARTESIAN_POINT('Ctrl Pts',(-0.0261976785729545,0.0133730672528979,
-0.003703609311004));
#52734=CARTESIAN_POINT('Ctrl Pts',(-0.0298247967320212,0.0107801243754552,
-0.00474823453246165));
#52735=CARTESIAN_POINT('Ctrl Pts',(-0.0278335547303766,0.0118279104841727,
-0.00401756090056744));
#52736=CARTESIAN_POINT('Ctrl Pts',(-0.0260567792745189,0.0133727645665508,
-0.0037867540289952));
#52737=CARTESIAN_POINT('Ctrl Pts',(-0.0295719930617066,0.0107334368600793,
-0.00486975437016942));
#52738=CARTESIAN_POINT('Ctrl Pts',(-0.0276479485836656,0.0118132632712226,
-0.00412070886673605));
#52739=CARTESIAN_POINT('Ctrl Pts',(-0.0259366131982632,0.0133725025804461,
-0.00385768385443678));
#52740=CARTESIAN_POINT('Ctrl Pts',(-0.0293515712931725,0.0106942893521317,
-0.00497757727446442));
#52741=CARTESIAN_POINT('Ctrl Pts',(-0.0274895265439536,0.0118010629011895,
-0.00420990088068877));
#52742=CARTESIAN_POINT('Ctrl Pts',(-0.0258384047699654,0.01337228380016,
-0.00391566918926073));
#52743=CARTESIAN_POINT('Ctrl Pts',(-0.0291391659279289,0.0106575655708569,
-0.0050828951244524));
#52744=CARTESIAN_POINT('Ctrl Pts',(-0.0273390541578014,0.0117896259521601,
-0.00429540644467852));
#52745=CARTESIAN_POINT('Ctrl Pts',(-0.0257479800864673,0.0133720783997972,
-0.00396907047371278));
#52746=CARTESIAN_POINT('Ctrl Pts',(-0.0289674849020721,0.0106289606342586,
-0.00516976597180735));
#52747=CARTESIAN_POINT('Ctrl Pts',(-0.02721969022651,0.0117806707763832,
-0.0043641191545271));
#52748=CARTESIAN_POINT('Ctrl Pts',(-0.0256793615951877,0.0133719173903702,
-0.00400960740700386));
#52749=CARTESIAN_POINT('Ctrl Pts',(-0.0289147502730564,0.0106122180693434,
-0.00520803367000348));
#52750=CARTESIAN_POINT('Ctrl Pts',(-0.0271378379892791,0.0117745370161908,
-0.00441172434704335));
#52751=CARTESIAN_POINT('Ctrl Pts',(-0.025633907607635,0.0133718071218718,
-0.00403646747319105));
#52752=CARTESIAN_POINT('Ctrl Pts',(-0.0288614479214877,0.0105959306253864,
-0.00524578660432017));
#52753=CARTESIAN_POINT('Ctrl Pts',(-0.0271290244595121,0.0117738703384706,
-0.00441686056377363));
#52754=CARTESIAN_POINT('Ctrl Pts',(-0.0256290366711919,0.0133717951397229,
-0.00403934602138506));
#52755=CARTESIAN_POINT('Ctrl Pts',(-0.0288073858068765,0.0105787676699155,
-0.00528498245870882));
#52756=CARTESIAN_POINT('Ctrl Pts',(-0.0271217175885171,0.0117733370610431,
-0.00442110236585357));
#52757=CARTESIAN_POINT('Ctrl Pts',(-0.0256248590438472,0.0133717159890139,
-0.00404186864921482));
#52758=CARTESIAN_POINT('Ctrl Pts',(-0.028753248636285,0.0105614142183789,
-0.00532451795721782));
#52759=CARTESIAN_POINT('Ctrl Pts',(-0.0271187092444645,0.0117744642076714,
-0.00442049835616301));
#52760=CARTESIAN_POINT('Ctrl Pts',(-0.0256213618193222,0.0133716002169367,
-0.00404401940088713));
#52761=CARTESIAN_POINT('Ctrl Pts',(-0.0286972824510733,0.0105432493465016,
-0.00536565854362216));
#52762=CARTESIAN_POINT('Ctrl Pts',(-0.0271115673024987,0.0117729678320726,
-0.00442531770637433));
#52763=CARTESIAN_POINT('Ctrl Pts',(-0.0256190493030287,0.0133714876905249,
-0.00404547015830714));
#52764=CARTESIAN_POINT('Ctrl Pts',(-0.0286411031923645,0.010524877141472,
-0.00540711703952029));
#52765=CARTESIAN_POINT('Ctrl Pts',(-0.0270915719571781,0.0117662732028744,
-0.00444208328235592));
#52766=CARTESIAN_POINT('Ctrl Pts',(-0.0256171019831343,0.01337135765012,
-0.00404671993903247));
#52767=CARTESIAN_POINT('Ctrl Pts',(-0.0285828830651116,0.0105057502210374,
-0.00544990797483098));
#52768=CARTESIAN_POINT('Ctrl Pts',(-0.0270727421042012,0.0117594675002445,
-0.00445920463210022));
#52769=CARTESIAN_POINT('Ctrl Pts',(-0.0256155327883204,0.0133712308031466,
-0.00404774448896239));
#52770=CARTESIAN_POINT('Ctrl Pts',(-0.0285246450454284,0.0104864150634632,
-0.00549316804071699));
#52771=CARTESIAN_POINT('Ctrl Pts',(-0.0270423634194359,0.0117483911363854,
-0.00448636607666542));
#52772=CARTESIAN_POINT('Ctrl Pts',(-0.0256138793235271,0.0133710771466519,
-0.00404883993594807));
#52773=CARTESIAN_POINT('Ctrl Pts',(-0.028465753619234,0.0104665820148817,
-0.00553745416170548));
#52774=CARTESIAN_POINT('Ctrl Pts',(-0.0269825259250966,0.0117268108665561,
-0.00453842518565841));
#52775=CARTESIAN_POINT('Ctrl Pts',(-0.0256114990915839,0.0133708330482361,
-0.00405043536832266));
#52776=CARTESIAN_POINT('Ctrl Pts',(-0.0284067653367236,0.0104463348507675,
-0.00558277907219412));
#52777=CARTESIAN_POINT('Ctrl Pts',(-0.0269035426341023,0.011698536842693,
-0.00460702967746145));
#52778=CARTESIAN_POINT('Ctrl Pts',(-0.025608425009902,0.0133704800254569,
-0.00405252594601399));
#52779=CARTESIAN_POINT('Ctrl Pts',(-0.0280675604554757,0.0103218692995789,
-0.00587331047521013));
#52780=CARTESIAN_POINT('Ctrl Pts',(-0.0267271007860639,0.0116361165146999,
-0.00475980726027247));
#52781=CARTESIAN_POINT('Ctrl Pts',(-0.0256002489243723,0.0133693958273193,
-0.00405820166310776));
#52782=CARTESIAN_POINT('Ctrl Pts',(-0.0277460264250124,0.0102161009525818,
-0.0061634089554616));
#52783=CARTESIAN_POINT('Ctrl Pts',(-0.0265551296789588,0.011577260405049,
-0.00490730587419467));
#52784=CARTESIAN_POINT('Ctrl Pts',(-0.0255890676586056,0.0133683816772428,
-0.00406559971933516));
#52785=CARTESIAN_POINT('Ctrl Pts',(-0.0274863162998273,0.0101367292540289,
-0.00640461551926327));
#52786=CARTESIAN_POINT('Ctrl Pts',(-0.0264124795131404,0.011529920823339,
-0.0050286097627996));
#52787=CARTESIAN_POINT('Ctrl Pts',(-0.0255757644815469,0.0133675703687158,
-0.00407409533213147));
#52788=CARTESIAN_POINT('Ctrl Pts',(-0.0272914928284565,0.0100812016712519,
-0.00658978567130121));
#52789=CARTESIAN_POINT('Ctrl Pts',(-0.0263030488949675,0.0114946427485996,
-0.00512099352964556));
#52790=CARTESIAN_POINT('Ctrl Pts',(-0.0255630018470322,0.013366968727325,
-0.0040821099818228));
#52791=CARTESIAN_POINT('Ctrl Pts',(-0.0270840414635881,0.0100254412579728,
-0.00679019156849944));
#52792=CARTESIAN_POINT('Ctrl Pts',(-0.0261841898257576,0.0114573548804285,
-0.00522070556443383));
#52793=CARTESIAN_POINT('Ctrl Pts',(-0.0255464591387835,0.0133663353614209,
-0.00409238655333308));
#52794=CARTESIAN_POINT('Ctrl Pts',(-0.0268835994452472,0.00997607256763211,
-0.00698779961283796));
#52795=CARTESIAN_POINT('Ctrl Pts',(-0.0260661813151271,0.0114218163578175,
-0.00531885137188345));
#52796=CARTESIAN_POINT('Ctrl Pts',(-0.0255263021183457,0.0133657349749526,
-0.00410477867652445));
#52797=CARTESIAN_POINT('Ctrl Pts',(-0.0266908179464102,0.00993278896673545,
-0.00718096844533468));
#52798=CARTESIAN_POINT('Ctrl Pts',(-0.0259495729075507,0.0113882771479691,
-0.0054150113612664));
#52799=CARTESIAN_POINT('Ctrl Pts',(-0.0255025273298817,0.0133651713259671,
-0.00411928732511149));
#52800=CARTESIAN_POINT('Ctrl Pts',(-0.0265287433143654,0.00989956116966734,
-0.00734541975738988));
#52801=CARTESIAN_POINT('Ctrl Pts',(-0.0258491621773471,0.0113606579109212,
-0.0054972041668335));
#52802=CARTESIAN_POINT('Ctrl Pts',(-0.0254790717439256,0.0133647093906794,
-0.00413353208185679));
#52803=CARTESIAN_POINT('Ctrl Pts',(-0.0263423809876361,0.00986455026007133,
-0.00753629868729644));
#52804=CARTESIAN_POINT('Ctrl Pts',(-0.0257312574486088,0.0113295756134489,
-0.00559310886750162));
#52805=CARTESIAN_POINT('Ctrl Pts',(-0.0254484295753836,0.0133641918274074,
-0.00415207922632118));
#52806=CARTESIAN_POINT('Ctrl Pts',(-0.0261481867185806,0.00983278279304436,
-0.00773746330827286));
#52807=CARTESIAN_POINT('Ctrl Pts',(-0.0256048170539434,0.0112983188867912,
-0.00569507952915905));
#52808=CARTESIAN_POINT('Ctrl Pts',(-0.0254109127952933,0.0133636745317756,
-0.00417470466049298));
#52809=CARTESIAN_POINT('Ctrl Pts',(-0.0259520714360624,0.00980574636897381,
-0.00794239949141725));
#52810=CARTESIAN_POINT('Ctrl Pts',(-0.0254733159889546,0.0112681849843151,
-0.00580023449269352));
#52811=CARTESIAN_POINT('Ctrl Pts',(-0.0253667807403883,0.0133631791111596,
-0.00420124155186773));
#52812=CARTESIAN_POINT('Ctrl Pts',(-0.025724264374708,0.00977962414268888,
-0.00818184634833232));
#52813=CARTESIAN_POINT('Ctrl Pts',(-0.0253165660483512,0.0112348349148003,
-0.00592469000507303));
#52814=CARTESIAN_POINT('Ctrl Pts',(-0.0253088183986679,0.0133626344216237,
-0.00423602339438577));
#52815=CARTESIAN_POINT('Ctrl Pts',(-0.0254843721584209,0.00975992424360273,
-0.00843536695618243));
#52816=CARTESIAN_POINT('Ctrl Pts',(-0.0251457422557053,0.0112024178504661,
-0.00605907812247795));
#52817=CARTESIAN_POINT('Ctrl Pts',(-0.0252376676352329,0.0133621100169332,
-0.00427862501603976));
#52818=CARTESIAN_POINT('Ctrl Pts',(-0.0252392523779962,0.00974825625449607,
-0.00869475393969651));
#52819=CARTESIAN_POINT('Ctrl Pts',(-0.0249651509091306,0.0111726248652654,
-0.00619993688839688));
#52820=CARTESIAN_POINT('Ctrl Pts',(-0.0251537017368419,0.0133616335190601,
-0.00432881130383831));
#52821=CARTESIAN_POINT('Ctrl Pts',(-0.0250252274687213,0.00974459884238429,
-0.00892086419570641));
#52822=CARTESIAN_POINT('Ctrl Pts',(-0.0248029092461888,0.0111494016223978,
-0.0063256338420981));
#52823=CARTESIAN_POINT('Ctrl Pts',(-0.0250715464480529,0.0133612665548016,
-0.00437785630142376));
#52824=CARTESIAN_POINT('Ctrl Pts',(-0.0248330956640217,0.00974647630868264,
-0.00912309242891329));
#52825=CARTESIAN_POINT('Ctrl Pts',(-0.0246537608279187,0.0111309194011829,
-0.00644057507543671));
#52826=CARTESIAN_POINT('Ctrl Pts',(-0.0249907066455409,0.0133609782590991,
-0.00442607439890494));
#52827=CARTESIAN_POINT('Ctrl Pts',(-0.0245992392867989,0.00975445323702422,
-0.00936798685351651));
#52828=CARTESIAN_POINT('Ctrl Pts',(-0.0244684134772241,0.0111111737434523,
-0.00658279010480466));
#52829=CARTESIAN_POINT('Ctrl Pts',(-0.0248844024824674,0.0133606748224033,
-0.00448943937177968));
#52830=CARTESIAN_POINT('Ctrl Pts',(-0.0243393500301934,0.00977216831379076,
-0.0096375484899141));
#52831=CARTESIAN_POINT('Ctrl Pts',(-0.0242567634085124,0.0110937425586607,
-0.00674428919556468));
#52832=CARTESIAN_POINT('Ctrl Pts',(-0.0247538271850526,0.013360414619455,
-0.00456721181626968));
#52833=CARTESIAN_POINT('Ctrl Pts',(-0.0240619644435389,0.00980124135293209,
-0.00992099818357101));
#52834=CARTESIAN_POINT('Ctrl Pts',(-0.0240246691820906,0.0110807496794517,
-0.00692046297213162));
#52835=CARTESIAN_POINT('Ctrl Pts',(-0.02459988346086,0.0133602315273817,
-0.00465884060783006));
#52836=CARTESIAN_POINT('Ctrl Pts',(-0.0237256093236952,0.00984721700118359,
-0.0102590817514845));
#52837=CARTESIAN_POINT('Ctrl Pts',(-0.0237368086416349,0.0110712816730396,
-0.00713804617400964));
#52838=CARTESIAN_POINT('Ctrl Pts',(-0.0243975472063884,0.0133601146533764,
-0.00477921310507474));
#52839=CARTESIAN_POINT('Ctrl Pts',(-0.0232026024969606,0.00994122487110758,
-0.0107704884933705));
#52840=CARTESIAN_POINT('Ctrl Pts',(-0.0232762649733642,0.011070587387176,
-0.00748425252227681));
#52841=CARTESIAN_POINT('Ctrl Pts',(-0.0240493425813566,0.0133601652903972,
-0.00498624593995807));
#52842=CARTESIAN_POINT('Ctrl Pts',(-0.0225740146247116,0.0100955861323387,
-0.0113494892384633));
#52843=CARTESIAN_POINT('Ctrl Pts',(-0.0227010714720119,0.0110984998660559,
-0.00791268507570289));
#52844=CARTESIAN_POINT('Ctrl Pts',(-0.0235661364076886,0.0133606964400032,
-0.00527333232331995));
#52845=CARTESIAN_POINT('Ctrl Pts',(-0.0219161527424833,0.0102913170500384,
-0.0119097490487537));
#52846=CARTESIAN_POINT('Ctrl Pts',(-0.0220819411571392,0.0111564260647825,
-0.0083679967886967));
#52847=CARTESIAN_POINT('Ctrl Pts',(-0.0230005865620769,0.0133617162333888,
-0.00560913016806318));
#52848=CARTESIAN_POINT('Ctrl Pts',(-0.0213172350541001,0.0104904030844707,
-0.0123799586077945));
#52849=CARTESIAN_POINT('Ctrl Pts',(-0.0215073227281529,0.0112302659879934,
-0.00878379991450101));
#52850=CARTESIAN_POINT('Ctrl Pts',(-0.0224436992424846,0.0133629840096402,
-0.00593960650541536));
#52851=CARTESIAN_POINT('Ctrl Pts',(-0.0209433957024175,0.010622740123274,
-0.0126501240251599));
#52852=CARTESIAN_POINT('Ctrl Pts',(-0.0211438108508993,0.0112868011786277,
-0.00904170165224759));
#52853=CARTESIAN_POINT('Ctrl Pts',(-0.0220761122516573,0.0133639433085236,
-0.006157634856723));
#52854=CARTESIAN_POINT('Ctrl Pts',(-0.0207607720679562,0.0106884755658043,
-0.0127768900671979));
#52855=CARTESIAN_POINT('Ctrl Pts',(-0.0209653293817326,0.0113164079967516,
-0.00916689820331034));
#52856=CARTESIAN_POINT('Ctrl Pts',(-0.0218928511860286,0.0133644439833726,
-0.00626630585176376));
#52857=CARTESIAN_POINT('',(-0.0275862774756162,0.0133330202728796,-0.00292880065737905));
#52858=CARTESIAN_POINT('Ctrl Pts',(-0.0275862774763506,0.013333020272888,
-0.00292880065694408));
#52859=CARTESIAN_POINT('Ctrl Pts',(-0.0276231848556899,0.0133334417442254,
-0.00290694105669624));
#52860=CARTESIAN_POINT('Ctrl Pts',(-0.0276608954101289,0.0133338715013257,
-0.00288460358966488));
#52861=CARTESIAN_POINT('Ctrl Pts',(-0.0276994051609495,0.0133343091774083,
-0.00286179020680056));
#52862=CARTESIAN_POINT('Ctrl Pts',(-0.0278520896348891,0.0133360444870636,
-0.0027713391057887));
#52863=CARTESIAN_POINT('Ctrl Pts',(-0.0280172941783116,0.013337904690857,
-0.00267343260130032));
#52864=CARTESIAN_POINT('Ctrl Pts',(-0.0281945943953082,0.0133398597451922,
-0.00256829614352595));
#52865=CARTESIAN_POINT('Ctrl Pts',(-0.0283492772393959,0.0133415654022411,
-0.00247657145992808));
#52866=CARTESIAN_POINT('Ctrl Pts',(-0.0285131649912883,0.0133433431611263,
-0.00237934434940374));
#52867=CARTESIAN_POINT('Ctrl Pts',(-0.0286864908250938,0.0133451700007234,
-0.00227646351282891));
#52868=CARTESIAN_POINT('Ctrl Pts',(-0.0287602956774135,0.0133459478976111,
-0.00223265524268692));
#52869=CARTESIAN_POINT('Ctrl Pts',(-0.0288358183015014,0.0133467346635766,
-0.00218781802139747));
#52870=CARTESIAN_POINT('Ctrl Pts',(-0.028913095790404,0.0133475282712897,
-0.00214192925684343));
#52871=CARTESIAN_POINT('Ctrl Pts',(-0.028999694532617,0.0133484176044027,
-0.00209050536421288));
#52872=CARTESIAN_POINT('Ctrl Pts',(-0.0290884724255105,0.0133493164175403,
-0.00203777409793986));
#52873=CARTESIAN_POINT('Ctrl Pts',(-0.0291793916664724,0.0133502203639561,
-0.00198375759913417));
#52874=CARTESIAN_POINT('Ctrl Pts',(-0.0293387692148659,0.0133518049434368,
-0.0018890689824962));
#52875=CARTESIAN_POINT('Ctrl Pts',(-0.0295047162972014,0.0133534051942572,
-0.00179043711833477));
#52876=CARTESIAN_POINT('Ctrl Pts',(-0.0296771691003025,0.0133549989591328,
-0.00168790140755359));
#52877=CARTESIAN_POINT('Ctrl Pts',(-0.0299962080745732,0.013357947436061,
-0.00149820957648156));
#52878=CARTESIAN_POINT('Ctrl Pts',(-0.0303374541903357,0.0133608714375898,
-0.00129519073320025));
#52879=CARTESIAN_POINT('Ctrl Pts',(-0.0307014085265843,0.0133636696479055,
-0.00107855839000479));
#52880=CARTESIAN_POINT('',(-0.0235554094661677,0.0133260932704124,-0.0053124061551198));
#52881=CARTESIAN_POINT('Ctrl Pts',(-0.0235554094661677,0.0133260932704124,
-0.0053124061551198));
#52882=CARTESIAN_POINT('Ctrl Pts',(-0.0235658492861846,0.0133260054407238,
-0.00530623551542229));
#52883=CARTESIAN_POINT('Ctrl Pts',(-0.0235762971536648,0.0133259176534734,
-0.00530005997256611));
#52884=CARTESIAN_POINT('Ctrl Pts',(-0.0235867539693412,0.0133258299168732,
-0.00529387898775706));
#52885=CARTESIAN_POINT('Ctrl Pts',(-0.0236783788545834,0.0133250611497673,
-0.0052397198592672));
#52886=CARTESIAN_POINT('Ctrl Pts',(-0.0237706788717137,0.0133242956193828,
-0.00518515084923147));
#52887=CARTESIAN_POINT('Ctrl Pts',(-0.0238578591296201,0.0133235786917102,
-0.00513360507976362));
#52888=CARTESIAN_POINT('Ctrl Pts',(-0.0239450393875266,0.0133228617640375,
-0.00508205931029576));
#52889=CARTESIAN_POINT('Ctrl Pts',(-0.024027099956465,0.0133221920484148,
-0.00503353693195624));
#52890=CARTESIAN_POINT('Ctrl Pts',(-0.0241277543322011,0.0133213953644077,
-0.00497400492496752));
#52891=CARTESIAN_POINT('Ctrl Pts',(-0.0241309185695083,0.0133213703193241,
-0.00497213343755219));
#52892=CARTESIAN_POINT('Ctrl Pts',(-0.0241341009493045,0.0133213451392199,
-0.00497025121882874));
#52893=CARTESIAN_POINT('Ctrl Pts',(-0.0241373005541634,0.0133213198334391,
-0.00496835880990149));
#52894=CARTESIAN_POINT('Ctrl Pts',(-0.0242302889664409,0.0133205843850071,
-0.00491336073692433));
#52895=CARTESIAN_POINT('Ctrl Pts',(-0.0243379925743662,0.0133197521448476,
-0.00484964914926691));
#52896=CARTESIAN_POINT('Ctrl Pts',(-0.0244369717904454,0.013319023633445,
-0.00479108410181297));
#52897=CARTESIAN_POINT('Ctrl Pts',(-0.0244429234182031,0.0133189798279992,
-0.00478756258107495));
#52898=CARTESIAN_POINT('Ctrl Pts',(-0.0244488428242526,0.0133189363515234,
-0.00478406010566338));
#52899=CARTESIAN_POINT('Ctrl Pts',(-0.0244547247477199,0.0133188932322421,
-0.00478057979824662));
#52900=CARTESIAN_POINT('Ctrl Pts',(-0.0245018576318574,0.0133185477098804,
-0.00475269148464483));
#52901=CARTESIAN_POINT('Ctrl Pts',(-0.0245466349835242,0.0133182287644832,
-0.00472619285369439));
#52902=CARTESIAN_POINT('Ctrl Pts',(-0.0245896441130481,0.0133179292759041,
-0.00470073895623896));
#52903=CARTESIAN_POINT('Ctrl Pts',(-0.0246437743023649,0.0133175523472457,
-0.00466870333256173));
#52904=CARTESIAN_POINT('Ctrl Pts',(-0.0246951009569881,0.013317206128952,
-0.00463832423661032));
#52905=CARTESIAN_POINT('Ctrl Pts',(-0.0247448283738734,0.0133168815166838,
-0.00460889008847095));
#52906=CARTESIAN_POINT('Ctrl Pts',(-0.0247993497452306,0.0133165256102819,
-0.00457661835143318));
#52907=CARTESIAN_POINT('Ctrl Pts',(-0.0248519631573275,0.0133161963315964,
-0.00454547346378711));
#52908=CARTESIAN_POINT('Ctrl Pts',(-0.0249032755518165,0.0133158882105585,
-0.00451509898440173));
#52909=CARTESIAN_POINT('Ctrl Pts',(-0.0249305427162006,0.0133157244764924,
-0.00449895812933675));
#52910=CARTESIAN_POINT('Ctrl Pts',(-0.0249574422684759,0.013315566681462,
-0.00448303496590283));
#52911=CARTESIAN_POINT('Ctrl Pts',(-0.0249840788117782,0.0133154157723874,
-0.00446726666635377));
#52912=CARTESIAN_POINT('Ctrl Pts',(-0.0249903076308074,0.0133153804830743,
-0.00446357933038167));
#52913=CARTESIAN_POINT('Ctrl Pts',(-0.0249965220598463,0.013315345569571,
-0.00445990046775898));
#52914=CARTESIAN_POINT('Ctrl Pts',(-0.0250027234833143,0.0133153110639603,
-0.00445622923316655));
#52915=CARTESIAN_POINT('Ctrl Pts',(-0.0250243757433542,0.0133151905876761,
-0.00444341112350606));
#52916=CARTESIAN_POINT('Ctrl Pts',(-0.02504585547353,0.0133150731717387,
-0.00443069599930903));
#52917=CARTESIAN_POINT('Ctrl Pts',(-0.0250662261098503,0.0133149652173997,
-0.0044186370787462));
#52918=CARTESIAN_POINT('Ctrl Pts',(-0.0250845012624421,0.0133148683680924,
-0.00440781863351386));
#52919=CARTESIAN_POINT('Ctrl Pts',(-0.0251018839688812,0.0133147791485272,
-0.00439752819845495));
#52920=CARTESIAN_POINT('Ctrl Pts',(-0.0251176667062615,0.0133146978585057,
-0.00438818677023798));
#52921=CARTESIAN_POINT('Ctrl Pts',(-0.0251289081109167,0.0133146399589155,
-0.00438153324923498));
#52922=CARTESIAN_POINT('Ctrl Pts',(-0.0251393672296564,0.0133145908840516,
-0.00437533966333391));
#52923=CARTESIAN_POINT('Ctrl Pts',(-0.0251500524476353,0.0133145402199908,
-0.00436901342239919));
#52924=CARTESIAN_POINT('Ctrl Pts',(-0.0251710911098042,0.0133144404649778,
-0.00435655736899099));
#52925=CARTESIAN_POINT('Ctrl Pts',(-0.025192958670792,0.0133143251891466,
-0.00434362187228724));
#52926=CARTESIAN_POINT('Ctrl Pts',(-0.0252237910271604,0.013314192950973,
-0.00432536835455965));
#52927=CARTESIAN_POINT('Ctrl Pts',(-0.0252277231277903,0.0133141760864233,
-0.00432304045371105));
#52928=CARTESIAN_POINT('Ctrl Pts',(-0.0252317980417083,0.0133141584760881,
-0.00432062824806579));
#52929=CARTESIAN_POINT('Ctrl Pts',(-0.0252359977075615,0.0133141402882188,
-0.00431814238915245));
#52930=CARTESIAN_POINT('Ctrl Pts',(-0.0252620229300343,0.0133140275784557,
-0.00430273758469499));
#52931=CARTESIAN_POINT('Ctrl Pts',(-0.0252928600872312,0.013313896033216,
-0.00428448956400194));
#52932=CARTESIAN_POINT('Ctrl Pts',(-0.0253242399560579,0.0133137859078515,
-0.00426591395739906));
#52933=CARTESIAN_POINT('Ctrl Pts',(-0.025339382382456,0.0133137327666088,
-0.0042569502565838));
#52934=CARTESIAN_POINT('Ctrl Pts',(-0.025354647350045,0.0133136840671119,
-0.00424791290030452));
#52935=CARTESIAN_POINT('Ctrl Pts',(-0.0253695236850595,0.0133136397773049,
-0.00423910620272196));
#52936=CARTESIAN_POINT('Ctrl Pts',(-0.0253776637620361,0.0133136155426774,
-0.00423428732790086));
#52937=CARTESIAN_POINT('Ctrl Pts',(-0.025385686741189,0.0133135924781677,
-0.00422953805765722));
#52938=CARTESIAN_POINT('Ctrl Pts',(-0.025393504626859,0.0133135696988639,
-0.0042249113754429));
#52939=CARTESIAN_POINT('Ctrl Pts',(-0.0254011519272082,0.0133135474166018,
-0.00422038564687547));
#52940=CARTESIAN_POINT('Ctrl Pts',(-0.0254086164986546,0.0133135303432495,
-0.00421596522967111));
#52941=CARTESIAN_POINT('Ctrl Pts',(-0.0254159159734615,0.0133135158404069,
-0.00421164170555362));
#52942=CARTESIAN_POINT('Ctrl Pts',(-0.0254326936382193,0.013313482505977,
-0.00420170419085085));
#52943=CARTESIAN_POINT('Ctrl Pts',(-0.0254486018479688,0.01331346370787,
-0.00419227621541077));
#52944=CARTESIAN_POINT('Ctrl Pts',(-0.0254638936319852,0.013313440647475,
-0.00418322235340209));
#52945=CARTESIAN_POINT('Ctrl Pts',(-0.0254723457635774,0.013313427901448,
-0.0041782180692039));
#52946=CARTESIAN_POINT('Ctrl Pts',(-0.02548060973331,0.0133134137623807,
-0.00417332804958735));
#52947=CARTESIAN_POINT('Ctrl Pts',(-0.0254887509034164,0.0133133986807665,
-0.0041685132251211));
#52948=CARTESIAN_POINT('Ctrl Pts',(-0.0254974507188984,0.013313382564255,
-0.00416336800841554));
#52949=CARTESIAN_POINT('Ctrl Pts',(-0.0255060083594711,0.0133133653499205,
-0.00415830983005533));
#52950=CARTESIAN_POINT('Ctrl Pts',(-0.0255144520821152,0.0133133487170901,
-0.00415332075634523));
#52951=CARTESIAN_POINT('Ctrl Pts',(-0.0255234397510192,0.0133133310127694,
-0.0041480102855334));
#52952=CARTESIAN_POINT('Ctrl Pts',(-0.0255322998610173,0.0133133140782046,
-0.00414277712651648));
#52953=CARTESIAN_POINT('Ctrl Pts',(-0.025541138662,0.0133133103101731,-0.00413754883754291));
#52954=CARTESIAN_POINT('Ctrl Pts',(-0.0255508709169214,0.013313306161257,
-0.00413179205659573));
#52955=CARTESIAN_POINT('Ctrl Pts',(-0.0255602311446517,0.0133132097520181,
-0.00412633228609686));
#52956=CARTESIAN_POINT('Ctrl Pts',(-0.0255694251152151,0.0133131030788275,
-0.00412098283208935));
#52957=CARTESIAN_POINT('Ctrl Pts',(-0.0255745194584301,0.0133130439716289,
-0.00411801872049696));
#52958=CARTESIAN_POINT('Ctrl Pts',(-0.0255795642442733,0.0133129821416654,
-0.00411508725653711));
#52959=CARTESIAN_POINT('Ctrl Pts',(-0.0255846258569396,0.0133129422693187,
-0.00411212978689285));
#52960=CARTESIAN_POINT('Ctrl Pts',(-0.025590046090682,0.0133128995719705,
-0.00410896277712441));
#52961=CARTESIAN_POINT('Ctrl Pts',(-0.0255954859018437,0.0133128822816128,
-0.00410576560489704));
#52962=CARTESIAN_POINT('Ctrl Pts',(-0.0256010393897212,0.0133129290762867,
-0.00410245246194853));
#52963=CARTESIAN_POINT('Ctrl Pts',(-0.0256069643995486,0.0133129790014703,
-0.00409891767354846));
#52964=CARTESIAN_POINT('Ctrl Pts',(-0.0256130260218243,0.0133131040811672,
-0.00409524488678633));
#52965=CARTESIAN_POINT('Ctrl Pts',(-0.0256196460291501,0.0133134494561625,
-0.00409107144979685));
#52966=CARTESIAN_POINT('Ctrl Pts',(-0.0256266540147968,0.0133138150725268,
-0.00408665342046849));
#52967=CARTESIAN_POINT('Ctrl Pts',(-0.0256342855896086,0.0133144294524892,
-0.00408167416892234));
#52968=CARTESIAN_POINT('Ctrl Pts',(-0.0256432107295599,0.0133156374582877,
-0.00407547308559459));
#52969=CARTESIAN_POINT('Ctrl Pts',(-0.0256476607973974,0.0133162397690392,
-0.00407238123027074));
#52970=CARTESIAN_POINT('Ctrl Pts',(-0.0256524196456054,0.0133169857056992,
-0.00406899627038609));
#52971=CARTESIAN_POINT('Ctrl Pts',(-0.0256571163719194,0.0133177495159941,
-0.00406563648960932));
#52972=CARTESIAN_POINT('Ctrl Pts',(-0.0256599283179211,0.0133182068118128,
-0.0040636249774431));
#52973=CARTESIAN_POINT('Ctrl Pts',(-0.0256624304973125,0.0133185527829313,
-0.00406185835776172));
#52974=CARTESIAN_POINT('Ctrl Pts',(-0.0256652294818525,0.0133190313235768,
-0.00405982373038196));
#52975=CARTESIAN_POINT('Ctrl Pts',(-0.0256670051399155,0.0133193349067312,
-0.00405853297565989));
#52976=CARTESIAN_POINT('Ctrl Pts',(-0.02566733914117,0.0133190911623826,
-0.00405853938508495));
#52977=CARTESIAN_POINT('Ctrl Pts',(-0.0256680603283604,0.0133189950409093,
-0.00405819528840961));
#52978=CARTESIAN_POINT('Ctrl Pts',(-0.0256702238899314,0.0133187066764896,
-0.00405716299838359));
#52979=CARTESIAN_POINT('Ctrl Pts',(-0.0256722642526714,0.0133183852673014,
-0.0040562418071485));
#52980=CARTESIAN_POINT('Ctrl Pts',(-0.0256743451903822,0.0133180897561963,
-0.0040552722719998));
#52981=CARTESIAN_POINT('Ctrl Pts',(-0.0256782135456918,0.0133175404163739,
-0.0040534699564279));
#52982=CARTESIAN_POINT('Ctrl Pts',(-0.0256820420627053,0.0133170010333836,
-0.00405165031151659));
#52983=CARTESIAN_POINT('Ctrl Pts',(-0.0256861152907195,0.0133165612437565,
-0.00404961831687978));
#52984=CARTESIAN_POINT('Ctrl Pts',(-0.025691321013244,0.0133159991778079,
-0.0040470213593283));
#52985=CARTESIAN_POINT('Ctrl Pts',(-0.0256967831203199,0.0133155506355026,
-0.00404418358848677));
#52986=CARTESIAN_POINT('Ctrl Pts',(-0.0257025001964393,0.0133151975592595,
-0.00404112191995521));
#52987=CARTESIAN_POINT('Ctrl Pts',(-0.0257059262049844,0.0133149859751908,
-0.00403928718794668));
#52988=CARTESIAN_POINT('Ctrl Pts',(-0.0257094427183089,0.0133148082117484,
-0.00403737284876931));
#52989=CARTESIAN_POINT('Ctrl Pts',(-0.0257130482103409,0.0133146598176385,
-0.00403538330608558));
#52990=CARTESIAN_POINT('Ctrl Pts',(-0.025716418021914,0.0133145211236172,
-0.00403352381398255));
#52991=CARTESIAN_POINT('Ctrl Pts',(-0.0257198655625725,0.0133144080891559,
-0.00403159862363874));
#52992=CARTESIAN_POINT('Ctrl Pts',(-0.0257233896074754,0.0133143169834006,
-0.00402961139958997));
#52993=CARTESIAN_POINT('Ctrl Pts',(-0.0257298831949792,0.0133141491072214,
-0.00402594963772084));
#52994=CARTESIAN_POINT('Ctrl Pts',(-0.0257366366872511,0.0133140556780819,
-0.00402207716712653));
#52995=CARTESIAN_POINT('Ctrl Pts',(-0.0257436378676088,0.0133140135523751,
-0.0040180194655019));
#52996=CARTESIAN_POINT('Ctrl Pts',(-0.0257500497609761,0.0133139749723748,
-0.00401430329925501));
#52997=CARTESIAN_POINT('Ctrl Pts',(-0.0257566692258838,0.0133139794221993,
-0.00401043187403818));
#52998=CARTESIAN_POINT('Ctrl Pts',(-0.0257634903945885,0.0133140092147305,
-0.00400642269257857));
#52999=CARTESIAN_POINT('Ctrl Pts',(-0.0257698356340983,0.0133140369285657,
-0.00400269324126305));
#53000=CARTESIAN_POINT('Ctrl Pts',(-0.0257763480144088,0.0133140870620743,
-0.00399884850704672));
#53001=CARTESIAN_POINT('Ctrl Pts',(-0.0257831074779253,0.0133141345249859,
-0.00399486191656997));
#53002=CARTESIAN_POINT('Ctrl Pts',(-0.0257954433060206,0.0133142211434457,
-0.0039875865026726));
#53003=CARTESIAN_POINT('Ctrl Pts',(-0.0258085091621843,0.0133143164096352,
-0.00397987888238915));
#53004=CARTESIAN_POINT('Ctrl Pts',(-0.0258219986413289,0.0133144171496422,
-0.00397192062861168));
#53005=CARTESIAN_POINT('Ctrl Pts',(-0.0258467124879595,0.0133146017137055,
-0.00395734044644182));
#53006=CARTESIAN_POINT('Ctrl Pts',(-0.0258728398361485,0.013314804507215,
-0.00394192412456912));
#53007=CARTESIAN_POINT('Ctrl Pts',(-0.0258986042167096,0.0133150081123963,
-0.00392672277812987));
#53008=CARTESIAN_POINT('Ctrl Pts',(-0.0259239054514451,0.0133152080575288,
-0.00391179469423348));
#53009=CARTESIAN_POINT('Ctrl Pts',(-0.025948756672967,0.0133154073743607,
-0.00389713319324261));
#53010=CARTESIAN_POINT('Ctrl Pts',(-0.0259738210178452,0.0133156125864984,
-0.00388234554344445));
#53011=CARTESIAN_POINT('Ctrl Pts',(-0.0259941857584619,0.013315779321036,
-0.00387033060134514));
#53012=CARTESIAN_POINT('Ctrl Pts',(-0.0260146939666128,0.0133159499947089,
-0.00385823074062121));
#53013=CARTESIAN_POINT('Ctrl Pts',(-0.0260356880624994,0.0133161278974167,
-0.00384584354779159));
#53014=CARTESIAN_POINT('Ctrl Pts',(-0.0260635406891899,0.0133163639189026,
-0.00382940960086232));
#53015=CARTESIAN_POINT('Ctrl Pts',(-0.0260922691739588,0.0133166131470457,
-0.00381245761385976));
#53016=CARTESIAN_POINT('Ctrl Pts',(-0.0261207052556074,0.0133168642412803,
-0.00379567757791817));
#53017=CARTESIAN_POINT('Ctrl Pts',(-0.0261391717990104,0.0133170273032183,
-0.00378478053289456));
#53018=CARTESIAN_POINT('Ctrl Pts',(-0.0261575168897512,0.0133171911778366,
-0.00377395487041613));
#53019=CARTESIAN_POINT('Ctrl Pts',(-0.0261754345333995,0.0133173528891302,
-0.00376338113887659));
#53020=CARTESIAN_POINT('Ctrl Pts',(-0.0261981887788342,0.0133175582519858,
-0.00374995318555116));
#53021=CARTESIAN_POINT('Ctrl Pts',(-0.0262202456375072,0.0133177598241401,
-0.00373693616987632));
#53022=CARTESIAN_POINT('Ctrl Pts',(-0.0262472884083519,0.0133180118477269,
-0.00372097482579748));
#53023=CARTESIAN_POINT('Ctrl Pts',(-0.0262526205118232,0.0133180615399662,
-0.00371782768016444));
#53024=CARTESIAN_POINT('Ctrl Pts',(-0.0262581494700475,0.0133181132552533,
-0.00371456427142578));
#53025=CARTESIAN_POINT('Ctrl Pts',(-0.0262636619228426,0.0133181649442378,
-0.00371131058327889));
#53026=CARTESIAN_POINT('Ctrl Pts',(-0.0262861069165848,0.0133183754057108,
-0.003698062576845));
#53027=CARTESIAN_POINT('Ctrl Pts',(-0.0263082508432428,0.0133185851392778,
-0.00368499224816668));
#53028=CARTESIAN_POINT('Ctrl Pts',(-0.0263159809211684,0.0133186588979533,
-0.00368042925426218));
#53029=CARTESIAN_POINT('Ctrl Pts',(-0.0263256094932595,0.0133187507716358,
-0.00367474559671252));
#53030=CARTESIAN_POINT('Ctrl Pts',(-0.0263307395568127,0.0133188000401663,
-0.0036717172746909));
#53031=CARTESIAN_POINT('Ctrl Pts',(-0.0263319848737224,0.0133188134113866,
-0.00367098093719014));
#53032=CARTESIAN_POINT('Ctrl Pts',(-0.026333230190632,0.0133188267826069,
-0.00367024459968939));
#53033=CARTESIAN_POINT('Ctrl Pts',(-0.0263395456796712,0.013318889131422,
-0.00366651502588641));
#53034=CARTESIAN_POINT('Ctrl Pts',(-0.0263453162169995,0.0133189470465933,
-0.00366310656008888));
#53035=CARTESIAN_POINT('Ctrl Pts',(-0.0263568572916562,0.0133190628769359,
-0.00365628962849381));
#53036=CARTESIAN_POINT('Ctrl Pts',(-0.0263662185232684,0.0133191608357306,
-0.00365075706076423));
#53037=CARTESIAN_POINT('Ctrl Pts',(-0.0263774051172533,0.0133192790955712,
-0.00364414486510002));
#53038=CARTESIAN_POINT('Ctrl Pts',(-0.0263852136259227,0.0133193616437527,
-0.0036395293952584));
#53039=CARTESIAN_POINT('Ctrl Pts',(-0.0263939120873735,0.0133194541160037,
-0.00363438756270788));
#53040=CARTESIAN_POINT('Ctrl Pts',(-0.0264033661707149,0.0133195552484065,
-0.00362879869285044));
#53041=CARTESIAN_POINT('Ctrl Pts',(-0.0264210002283535,0.0133197438837884,
-0.00361837415462276));
#53042=CARTESIAN_POINT('Ctrl Pts',(-0.0264412619599893,0.0133199626359746,
-0.00360639506375529));
#53043=CARTESIAN_POINT('Ctrl Pts',(-0.0264632883923973,0.0133202033893144,
-0.00359337083805423));
#53044=CARTESIAN_POINT('Ctrl Pts',(-0.0264868575491462,0.0133204610049418,
-0.00357943439971524));
#53045=CARTESIAN_POINT('Ctrl Pts',(-0.0265124435758176,0.0133207437319668,
-0.00356430348948096));
#53046=CARTESIAN_POINT('Ctrl Pts',(-0.0265403341313379,0.0133210544187678,
-0.00354780836682767));
#53047=CARTESIAN_POINT('Ctrl Pts',(-0.0265524826683329,0.0133211897473773,
-0.00354062343974201));
#53048=CARTESIAN_POINT('Ctrl Pts',(-0.0265650682768647,0.0133213303791844,
-0.00353317977739553));
#53049=CARTESIAN_POINT('Ctrl Pts',(-0.0265781131869612,0.0133214765333346,
-0.0035254642574458));
#53050=CARTESIAN_POINT('Ctrl Pts',(-0.0266080173883094,0.0133218115776625,
-0.00350777717026943));
#53051=CARTESIAN_POINT('Ctrl Pts',(-0.0266403402986276,0.013322175706965,
-0.0034886584880915));
#53052=CARTESIAN_POINT('Ctrl Pts',(-0.0266750102819012,0.0133225682144268,
-0.00346815026368034));
#53053=CARTESIAN_POINT('Ctrl Pts',(-0.0266901854316553,0.0133227400160532,
-0.00345917375584149));
#53054=CARTESIAN_POINT('Ctrl Pts',(-0.0267058101198676,0.013322917254059,
-0.00344993110061026));
#53055=CARTESIAN_POINT('Ctrl Pts',(-0.0267218794657746,0.0133230998692401,
-0.00344042515662456));
#53056=CARTESIAN_POINT('Ctrl Pts',(-0.0267868074182936,0.0133238377231562,
-0.00340201653169836));
#53057=CARTESIAN_POINT('Ctrl Pts',(-0.0268589945355396,0.0133246635634664,
-0.00335930986383769));
#53058=CARTESIAN_POINT('Ctrl Pts',(-0.0269384557012431,0.0133255760705762,
-0.00331229269516491));
#53059=CARTESIAN_POINT('Ctrl Pts',(-0.0269881881929531,0.0133261471829161,
-0.00328286598174403));
#53060=CARTESIAN_POINT('Ctrl Pts',(-0.0270407743232821,0.0133267522722069,
-0.00325174815222461));
#53061=CARTESIAN_POINT('Ctrl Pts',(-0.0270962258102821,0.0133273907515286,
-0.0032189309120574));
#53062=CARTESIAN_POINT('Ctrl Pts',(-0.027128492095011,0.0133277622718738,
-0.00319983511368408));
#53063=CARTESIAN_POINT('Ctrl Pts',(-0.0271617320198951,0.0133281451225746,
-0.00318016186272851));
#53064=CARTESIAN_POINT('Ctrl Pts',(-0.0271959409457542,0.0133285390596639,
-0.00315991352662765));
#53065=CARTESIAN_POINT('Ctrl Pts',(-0.0272751668494086,0.0133294513952926,
-0.00311301954545746));
#53066=CARTESIAN_POINT('Ctrl Pts',(-0.0273595817593857,0.0133304232143139,
-0.00306304608089671));
#53067=CARTESIAN_POINT('Ctrl Pts',(-0.0274491686173471,0.0133314508324888,
-0.00300999805464631));
#53068=CARTESIAN_POINT('Ctrl Pts',(-0.0274935948706356,0.0133319604298378,
-0.00298369146119856));
#53069=CARTESIAN_POINT('Ctrl Pts',(-0.0275392950129729,0.0133324837470758,
-0.00295662755461286));
#53070=CARTESIAN_POINT('Ctrl Pts',(-0.0275862774756162,0.0133330202728796,
-0.00292880065737905));
#53071=CARTESIAN_POINT('',(-0.021934236877081,0.0133389875988728,-0.006269352674027));
#53072=CARTESIAN_POINT('Ctrl Pts',(-0.0219343960410907,0.0133402928895198,
-0.00626914890761956));
#53073=CARTESIAN_POINT('Ctrl Pts',(-0.0221010109600867,0.0133388040944903,
-0.00617097210686397));
#53074=CARTESIAN_POINT('Ctrl Pts',(-0.0222672606248728,0.0133373214146564,
-0.00607295491232374));
#53075=CARTESIAN_POINT('Ctrl Pts',(-0.0224327397694273,0.013335852111634,
-0.00597534331956286));
#53076=CARTESIAN_POINT('Ctrl Pts',(-0.0226194004271091,0.0133341947362031,
-0.00586523733520354));
#53077=CARTESIAN_POINT('Ctrl Pts',(-0.0228050863246761,0.0133325545074323,
-0.00575564406051703));
#53078=CARTESIAN_POINT('Ctrl Pts',(-0.0229892794527548,0.0133309487573771,
-0.00564687592167325));
#53079=CARTESIAN_POINT('Ctrl Pts',(-0.0230064944725306,0.0133307986810999,
-0.00563671025653309));
#53080=CARTESIAN_POINT('Ctrl Pts',(-0.0230236963551825,0.0133306489032939,
-0.00562655185798805));
#53081=CARTESIAN_POINT('Ctrl Pts',(-0.0230408849525679,0.0133304994498391,
-0.00561640081208492));
#53082=CARTESIAN_POINT('Ctrl Pts',(-0.0232125654633601,0.0133290067017762,
-0.00551501169308644));
#53083=CARTESIAN_POINT('Ctrl Pts',(-0.0233828973440132,0.0133275446063501,
-0.00541437248667966));
#53084=CARTESIAN_POINT('Ctrl Pts',(-0.0235554094655405,0.0133260932704177,
-0.00531240615549051));
#53085=CARTESIAN_POINT('Ctrl Pts',(-0.021934236877081,0.0133389875988728,
-0.006269352674027));
#53086=CARTESIAN_POINT('Ctrl Pts',(-0.0221244379879695,0.0132862526669668,
-0.00621537843223214));
#53087=CARTESIAN_POINT('Ctrl Pts',(-0.0223140219160993,0.0132306176275604,
-0.00616200003189472));
#53088=CARTESIAN_POINT('Ctrl Pts',(-0.0225030808082205,0.013172076313167,
-0.00610925172191726));
#53089=CARTESIAN_POINT('Ctrl Pts',(-0.0227866691464023,0.013084264341577,
-0.00603012925695107));
#53090=CARTESIAN_POINT('Ctrl Pts',(-0.0230691000748747,0.0129895128254907,
-0.00595283182554986));
#53091=CARTESIAN_POINT('Ctrl Pts',(-0.0233502330550342,0.012889386081325,
-0.00587583756451714));
#53092=CARTESIAN_POINT('Ctrl Pts',(-0.0234273680673945,0.0128619141082948,
-0.00585471249668248));
#53093=CARTESIAN_POINT('Ctrl Pts',(-0.0235043864468972,0.0128340534807241,
-0.00583360617318919));
#53094=CARTESIAN_POINT('Ctrl Pts',(-0.0235813254974928,0.0128057960779319,
-0.00581250261525141));
#53095=CARTESIAN_POINT('Ctrl Pts',(-0.0236445958273245,0.0127825587858024,
-0.00579514824109406));
#53096=CARTESIAN_POINT('Ctrl Pts',(-0.0237078125907882,0.0127590528916518,
-0.00577779571524744));
#53097=CARTESIAN_POINT('Ctrl Pts',(-0.0237709578668766,0.0127353398478756,
-0.00576044610301269));
#53098=CARTESIAN_POINT('Ctrl Pts',(-0.0239108901236044,0.0126827908697884,
-0.00572199872351335));
#53099=CARTESIAN_POINT('Ctrl Pts',(-0.0240505530379959,0.0126291559746613,
-0.00568358176343615));
#53100=CARTESIAN_POINT('Ctrl Pts',(-0.0241900554418891,0.0125744693256945,
-0.00564565827841772));
#53101=CARTESIAN_POINT('Ctrl Pts',(-0.0243428100869491,0.0125145876360655,
-0.00560413219476783));
#53102=CARTESIAN_POINT('Ctrl Pts',(-0.0244958325837244,0.0124536079758719,
-0.00556270802296106));
#53103=CARTESIAN_POINT('Ctrl Pts',(-0.0246485110185659,0.0123926840260268,
-0.00552149208076619));
#53104=CARTESIAN_POINT('Ctrl Pts',(-0.0248676533978527,0.0123052386750284,
-0.00546233402320219));
#53105=CARTESIAN_POINT('Ctrl Pts',(-0.0250860103864501,0.0122179134029239,
-0.00540356193702577));
#53106=CARTESIAN_POINT('Ctrl Pts',(-0.0253058428404908,0.0121317907564844,
-0.00534636928812283));
#53107=CARTESIAN_POINT('Ctrl Pts',(-0.025409854912204,0.0120910424742679,
-0.00531930901658501));
#53108=CARTESIAN_POINT('Ctrl Pts',(-0.025514105172312,0.0120506121521787,
-0.00529263864486529));
#53109=CARTESIAN_POINT('Ctrl Pts',(-0.0256185902781894,0.0120107696834393,
-0.00526661730777513));
#53110=CARTESIAN_POINT('Ctrl Pts',(-0.0258887931628178,0.0119077353811463,
-0.00519932503406196));
#53111=CARTESIAN_POINT('Ctrl Pts',(-0.0261609591863951,0.0118084686899625,
-0.00513642094242103));
#53112=CARTESIAN_POINT('Ctrl Pts',(-0.026435864555564,0.0117172838915229,
-0.00507630138131902));
#53113=CARTESIAN_POINT('Ctrl Pts',(-0.0267549594990146,0.0116114416222736,
-0.00500651792089364));
#53114=CARTESIAN_POINT('Ctrl Pts',(-0.0270772042033137,0.0115156201751239,
-0.00494196151769574));
#53115=CARTESIAN_POINT('Ctrl Pts',(-0.0274040024921295,0.0114364512905921,
-0.00487608698319497));
#53116=CARTESIAN_POINT('Ctrl Pts',(-0.0274676159407365,0.0114210405435357,
-0.00486326406931082));
#53117=CARTESIAN_POINT('Ctrl Pts',(-0.0275313957257365,0.0114062481348544,
-0.00485039082995094));
#53118=CARTESIAN_POINT('Ctrl Pts',(-0.0275952102983737,0.0113920884570937,
-0.00483746324422098));
#53119=CARTESIAN_POINT('Ctrl Pts',(-0.0276441660591478,0.0113812257690203,
-0.0048275457634916));
#53120=CARTESIAN_POINT('Ctrl Pts',(-0.0276931984743864,0.0113707704701278,
-0.00481753463435697));
#53121=CARTESIAN_POINT('Ctrl Pts',(-0.0277423037157662,0.011360693633868,
-0.00480744239356394));
#53122=CARTESIAN_POINT('Ctrl Pts',(-0.0279359503616762,0.0113209556041127,
-0.00476764361599214));
#53123=CARTESIAN_POINT('Ctrl Pts',(-0.0281307195105546,0.0112867138806755,
-0.0047269782631293));
#53124=CARTESIAN_POINT('Ctrl Pts',(-0.0283264381759335,0.0112568152902019,
-0.00468571290726134));
#53125=CARTESIAN_POINT('Ctrl Pts',(-0.0284781341834278,0.011233641737512,
-0.00465372929588281));
#53126=CARTESIAN_POINT('Ctrl Pts',(-0.0286304059966229,0.0112130804841673,
-0.00462138545453646));
#53127=CARTESIAN_POINT('Ctrl Pts',(-0.0287832375202268,0.0111944774250573,
-0.00458937054336652));
#53128=CARTESIAN_POINT('Ctrl Pts',(-0.0289476373790355,0.0111744662374502,
-0.00455493231523136));
#53129=CARTESIAN_POINT('Ctrl Pts',(-0.0291130260495294,0.0111571002073237,
-0.00452035107554437));
#53130=CARTESIAN_POINT('Ctrl Pts',(-0.0292789073303117,0.0111420264190303,
-0.00448619822421547));
#53131=CARTESIAN_POINT('Ctrl Pts',(-0.0299202700594218,0.0110837451834847,
-0.00435414977467429));
#53132=CARTESIAN_POINT('Ctrl Pts',(-0.0305690256497348,0.0110598368200697,
-0.00422848437704382));
#53133=CARTESIAN_POINT('Ctrl Pts',(-0.0312271855506422,0.0110770582020895,
-0.00409339326150648));
#53134=CARTESIAN_POINT('Ctrl Pts',(-0.0312271855506433,0.0110770582020895,
-0.00409339326150625));
#53135=CARTESIAN_POINT('Ctrl Pts',(-0.0312971725477488,0.0104364367400133,
-0.00488270156062033));
#53136=CARTESIAN_POINT('Ctrl Pts',(-0.0312862115324834,0.00944637453608863,
-0.00512344689700543));
#53137=CARTESIAN_POINT('Ctrl Pts',(-0.0305674031038234,0.0110597943661587,
-0.00422881741200909));
#53138=CARTESIAN_POINT('Ctrl Pts',(-0.0306178286006085,0.0103975205083563,
-0.00501002528531751));
#53139=CARTESIAN_POINT('Ctrl Pts',(-0.0305722734913362,0.00939656088554349,
-0.00522936460674402));
#53140=CARTESIAN_POINT('Ctrl Pts',(-0.0295956996016403,0.0110958118217198,
-0.00441702265247476));
#53141=CARTESIAN_POINT('Ctrl Pts',(-0.0296215818436791,0.0104181961783084,
-0.00517881942381199));
#53142=CARTESIAN_POINT('Ctrl Pts',(-0.0295240270448467,0.00942242940763544,
-0.00537967666314561));
#53143=CARTESIAN_POINT('Ctrl Pts',(-0.0283214216202437,0.0112464614327918,
-0.00468728444716199));
#53144=CARTESIAN_POINT('Ctrl Pts',(-0.028317220896715,0.0105655209977464,
-0.00541669869160581));
#53145=CARTESIAN_POINT('Ctrl Pts',(-0.028165494675058,0.00959724956687946,
-0.00560524719473936));
#53146=CARTESIAN_POINT('Ctrl Pts',(-0.0270873250160756,0.0114863644955833,
-0.00493805869436477));
#53147=CARTESIAN_POINT('Ctrl Pts',(-0.0270485620566154,0.0108042612517661,
-0.00566409311455983));
#53148=CARTESIAN_POINT('Ctrl Pts',(-0.0268298123068287,0.00984882112906849,
-0.00585320069877968));
#53149=CARTESIAN_POINT('Ctrl Pts',(-0.0259522259935078,0.0118716618249161,
-0.00517112075449145));
#53150=CARTESIAN_POINT('Ctrl Pts',(-0.0258585426933969,0.0112088416702644,
-0.00591420339096557));
#53151=CARTESIAN_POINT('Ctrl Pts',(-0.0255382372099837,0.0102851320010729,
-0.00612706727425103));
#53152=CARTESIAN_POINT('Ctrl Pts',(-0.0246675440919105,0.012385309732819,
-0.00551587592937417));
#53153=CARTESIAN_POINT('Ctrl Pts',(-0.0245918920667609,0.0117186747542567,
-0.00623782606164431));
#53154=CARTESIAN_POINT('Ctrl Pts',(-0.0242771565906109,0.0108089452162191,
-0.00644811086918074));
#53155=CARTESIAN_POINT('Ctrl Pts',(-0.0232306431468797,0.0129584151226383,
-0.00590506038327814));
#53156=CARTESIAN_POINT('Ctrl Pts',(-0.0232456059885352,0.0122404369636077,
-0.00664101298772188));
#53157=CARTESIAN_POINT('Ctrl Pts',(-0.0230068651290133,0.0112567720241337,
-0.00682535438580635));
#53158=CARTESIAN_POINT('Ctrl Pts',(-0.0213063980437958,0.0135554252605759,
-0.00644100233681364));
#53159=CARTESIAN_POINT('Ctrl Pts',(-0.0214852275357793,0.0127443835685822,
-0.00728906181719641));
#53160=CARTESIAN_POINT('Ctrl Pts',(-0.0213700943777464,0.0115684868389236,
-0.00741362551099617));
#53161=CARTESIAN_POINT('Ctrl Pts',(-0.0189589293125837,0.0139588978082077,
-0.00714392830883555));
#53162=CARTESIAN_POINT('Ctrl Pts',(-0.0193481840631595,0.0130853604144522,
-0.0081987090774338));
#53163=CARTESIAN_POINT('Ctrl Pts',(-0.0193354807706988,0.0116626127714134,
-0.00825016263078458));
#53164=CARTESIAN_POINT('Ctrl Pts',(-0.0170471348458498,0.0141103532818413,
-0.00776507163445552));
#53165=CARTESIAN_POINT('Ctrl Pts',(-0.0176087403647826,0.0132343476767644,
-0.00899849195367984));
#53166=CARTESIAN_POINT('Ctrl Pts',(-0.0176504495282693,0.0116214653221526,
-0.00900227953763803));
#53167=CARTESIAN_POINT('Ctrl Pts',(-0.0155198771543919,0.0141607759349565,
-0.00827772815388904));
#53168=CARTESIAN_POINT('Ctrl Pts',(-0.0162143626795666,0.0133115262354637,
-0.00966525099856111));
#53169=CARTESIAN_POINT('Ctrl Pts',(-0.0163007154697231,0.0115450617448305,
-0.00963487767203659));
#53170=CARTESIAN_POINT('Ctrl Pts',(-0.0147476420715683,0.0141642785739701,
-0.00853349038223322));
#53171=CARTESIAN_POINT('Ctrl Pts',(-0.0155272812960161,0.0133414507084357,
-0.010003407102025));
#53172=CARTESIAN_POINT('Ctrl Pts',(-0.0156467725429645,0.0114898180989373,
-0.00995062286346207));
#53173=CARTESIAN_POINT('Ctrl Pts',(-0.0143548534745897,0.0141605057808234,
-0.00865910748104471));
#53174=CARTESIAN_POINT('Ctrl Pts',(-0.0151686127038861,0.0133556215237912,
-0.0101803383457646));
#53175=CARTESIAN_POINT('Ctrl Pts',(-0.0153031792648842,0.0114576562027847,
-0.0101186490016487));
#53176=CARTESIAN_POINT('',(-0.0199408189736793,0.0133213265168279,-0.0073387013155759));
#53177=CARTESIAN_POINT('Ctrl Pts',(-0.0219342368770961,0.0133389875988686,
-0.00626935267402273));
#53178=CARTESIAN_POINT('Ctrl Pts',(-0.0217376785013481,0.0133366453122945,
-0.00639030610905115));
#53179=CARTESIAN_POINT('Ctrl Pts',(-0.0215381987658809,0.0133344476531088,
-0.00650627497520774));
#53180=CARTESIAN_POINT('Ctrl Pts',(-0.021336704249506,0.0133323524489406,
-0.00661859857317656));
#53181=CARTESIAN_POINT('Ctrl Pts',(-0.0208796013372672,0.0133275993472472,
-0.00687341168009572));
#53182=CARTESIAN_POINT('Ctrl Pts',(-0.0204118273091042,0.0133241114174165,
-0.00710983367692451));
#53183=CARTESIAN_POINT('Ctrl Pts',(-0.0199408531165797,0.0133213859277168,
-0.00733877226188682));
#53184=CARTESIAN_POINT('',(-0.0179635469613193,0.0125504668006521,-0.00868818357736758));
#53185=CARTESIAN_POINT('Ctrl Pts',(-0.019940832013525,0.013321303084259,
-0.00733866153639121));
#53186=CARTESIAN_POINT('Ctrl Pts',(-0.0199603396185445,0.0132772806325954,
-0.00736654069053705));
#53187=CARTESIAN_POINT('Ctrl Pts',(-0.0199132772454676,0.0132018530803466,
-0.00744866955051636));
#53188=CARTESIAN_POINT('Ctrl Pts',(-0.0197781204736182,0.0131072852390325,
-0.00758075520135114));
#53189=CARTESIAN_POINT('Ctrl Pts',(-0.0195745132232924,0.0130117329433713,
-0.00773781403254475));
#53190=CARTESIAN_POINT('Ctrl Pts',(-0.0193204817770644,0.0129169799429281,
-0.00790952535011119));
#53191=CARTESIAN_POINT('Ctrl Pts',(-0.0189699447034221,0.0128035104283324,
-0.00812880984283259));
#53192=CARTESIAN_POINT('Ctrl Pts',(-0.0185188307304575,0.0126793170927796,
-0.00838884190036944));
#53193=CARTESIAN_POINT('Ctrl Pts',(-0.018149541483532,0.0125918489633789,
-0.00858915670411014));
#53194=CARTESIAN_POINT('Ctrl Pts',(-0.0179635437328199,0.0125504640932136,
-0.00868817638106961));
#53195=CARTESIAN_POINT('Ctrl Pts',(-0.0179635534180534,0.0125504722160869,
-0.00868819796987369));
#53196=CARTESIAN_POINT('Ctrl Pts',(-0.0177344418480487,0.0124994925802867,
-0.00881016396521778));
#53197=CARTESIAN_POINT('Ctrl Pts',(-0.0175066087155722,0.0124440548773491,
-0.00893192475792164));
#53198=CARTESIAN_POINT('Ctrl Pts',(-0.0172802067201601,0.0123833234404231,
-0.00905334530314095));
#53199=CARTESIAN_POINT('Ctrl Pts',(-0.0172702574635162,0.0123806545918061,
-0.00905868114023916));
#53200=CARTESIAN_POINT('Ctrl Pts',(-0.0172603111720795,0.0123779754035313,
-0.00906401620513647));
#53201=CARTESIAN_POINT('Ctrl Pts',(-0.0172503677772368,0.0123752856701961,
-0.00906935054629216));
#53202=CARTESIAN_POINT('Ctrl Pts',(-0.0170340425658767,0.0123167687208602,
-0.00918540270918222));
#53203=CARTESIAN_POINT('Ctrl Pts',(-0.0168190666854423,0.0122533080221976,
-0.00930117599300669));
#53204=CARTESIAN_POINT('Ctrl Pts',(-0.0166061640651018,0.0121821155570041,
-0.00941621999680577));
#53205=CARTESIAN_POINT('Ctrl Pts',(-0.0164948197172596,0.012144883142506,
-0.00947638599925169));
#53206=CARTESIAN_POINT('Ctrl Pts',(-0.016384039145408,0.0121055365709686,
-0.00953635007489573));
#53207=CARTESIAN_POINT('Ctrl Pts',(-0.0162739869952414,0.0120629969620388,
-0.00959602607418241));
#53208=CARTESIAN_POINT('Ctrl Pts',(-0.0162700848817242,0.0120614886372785,
-0.00959814200306811));
#53209=CARTESIAN_POINT('Ctrl Pts',(-0.0162661836345646,0.0120599763009443,
-0.00960025757130618));
#53210=CARTESIAN_POINT('Ctrl Pts',(-0.0162622833351437,0.0120584598728285,
-0.00960237274228974));
#53211=CARTESIAN_POINT('Ctrl Pts',(-0.01615618264775,0.0120172081513313,
-0.00965991219531522));
#53212=CARTESIAN_POINT('Ctrl Pts',(-0.0160507954251391,0.0119729279934615,
-0.00971718141157779));
#53213=CARTESIAN_POINT('Ctrl Pts',(-0.0159468166798295,0.0119240122610053,
-0.0097736976224013));
#53214=CARTESIAN_POINT('Ctrl Pts',(-0.0158390156384532,0.0118732983686345,
-0.00983229138945709));
#53215=CARTESIAN_POINT('Ctrl Pts',(-0.0157327819795801,0.0118176187396,
-0.00989018624054665));
#53216=CARTESIAN_POINT('Ctrl Pts',(-0.0156332637808036,0.0117499022711538,
-0.00994442202611638));
#53217=CARTESIAN_POINT('Ctrl Pts',(-0.0155835046814153,0.0117160440369307,
-0.00997153991890124));
#53218=CARTESIAN_POINT('Ctrl Pts',(-0.0155354394278101,0.0116791790329133,
-0.00999777428168848));
#53219=CARTESIAN_POINT('Ctrl Pts',(-0.0154908483194925,0.0116337739903578,
-0.0100220264279572));
#53220=CARTESIAN_POINT('Ctrl Pts',(-0.0154462572111749,0.0115883689478023,
-0.0100462785742259));
#53221=CARTESIAN_POINT('Ctrl Pts',(-0.015405193404354,0.0115344307061892,
-0.0100686588757623));
#53222=CARTESIAN_POINT('Ctrl Pts',(-0.0153993022433837,0.0114667765373356,
-0.0100716954734325));
#53223=CARTESIAN_POINT('Ctrl Pts',(-0.031227186149515,0.0110770527203336,
-0.00409340001554567));
#53224=CARTESIAN_POINT('Ctrl Pts',(-0.0312640532610597,0.0107214346812047,
-0.00453189580156053));
#53225=CARTESIAN_POINT('Ctrl Pts',(-0.0312844616188089,0.0102385845359009,
-0.00486793065315416));
#53226=CARTESIAN_POINT('Ctrl Pts',(-0.031286535045435,0.00970177877551689,
-0.00504944931744486));
#53227=CARTESIAN_POINT('Ctrl Pts',(-0.0312868594344739,0.00961779514064571,
-0.00507784803882443));
#53228=CARTESIAN_POINT('Ctrl Pts',(-0.0312867487379335,0.00953254752741736,
-0.00510254750827983));
#53229=CARTESIAN_POINT('Ctrl Pts',(-0.031286211601055,0.00944638135331241,
-0.00512344524021589));
#53230=CARTESIAN_POINT('Origin',(-0.0317929661854822,0.00871120572661458,
-0.00213559619862456));
#53231=CARTESIAN_POINT('Ctrl Pts',(-0.0348080115825784,0.00509687525187179,
-0.00461569088578222));
#53232=CARTESIAN_POINT('Ctrl Pts',(-0.0347548891167709,0.00446629142979133,
-0.00433411181330694));
#53233=CARTESIAN_POINT('Ctrl Pts',(-0.0346843926247131,0.00402081228213221,
-0.0038052049414957));
#53234=CARTESIAN_POINT('Ctrl Pts',(-0.0332875621972097,0.00551905813026757,
-0.0048853855816232));
#53235=CARTESIAN_POINT('Ctrl Pts',(-0.0332621390258117,0.00478601213496154,
-0.00466482167991226));
#53236=CARTESIAN_POINT('Ctrl Pts',(-0.0332218425615931,0.00424926308106939,
-0.00412352454144985));
#53237=CARTESIAN_POINT('Ctrl Pts',(-0.0316267399577887,0.00557241894549665,
-0.00506047006495692));
#53238=CARTESIAN_POINT('Ctrl Pts',(-0.0316907003603952,0.00481889725260965,
-0.00486557021719565));
#53239=CARTESIAN_POINT('Ctrl Pts',(-0.0316934649721066,0.00425079470032948,
-0.00433058506958464));
#53240=CARTESIAN_POINT('Ctrl Pts',(-0.0298458444280582,0.00532758970197972,
-0.0052928024035983));
#53241=CARTESIAN_POINT('Ctrl Pts',(-0.0299584793993426,0.00461004696303067,
-0.00511576159414239));
#53242=CARTESIAN_POINT('Ctrl Pts',(-0.0300009414693827,0.00405085754226072,
-0.00462151390208107));
#53243=CARTESIAN_POINT('Ctrl Pts',(-0.0290810914906223,0.00518348075480775,
-0.00539636057852287));
#53244=CARTESIAN_POINT('Ctrl Pts',(-0.0292393121166008,0.00446527121083198,
-0.00521590130342139));
#53245=CARTESIAN_POINT('Ctrl Pts',(-0.0293136858521343,0.00390564420165416,
-0.0047116415943142));
#53246=CARTESIAN_POINT('Ctrl Pts',(-0.0281474033824572,0.00491192722094244,
-0.00552736398019822));
#53247=CARTESIAN_POINT('Ctrl Pts',(-0.0283533171115081,0.00421434854492473,
-0.00534056257578605));
#53248=CARTESIAN_POINT('Ctrl Pts',(-0.0284603778430982,0.00366783441342131,
-0.00483752590032366));
#53249=CARTESIAN_POINT('Ctrl Pts',(-0.0272393145892442,0.00454861707918601,
-0.00567042035975692));
#53250=CARTESIAN_POINT('Ctrl Pts',(-0.0274894758152918,0.00387773041136884,
-0.00547497754196955));
#53251=CARTESIAN_POINT('Ctrl Pts',(-0.0276272202063975,0.00334894460118206,
-0.00497305746395805));
#53252=CARTESIAN_POINT('Ctrl Pts',(-0.0265464409363679,0.00419219894647591,
-0.00578556885600068));
#53253=CARTESIAN_POINT('Ctrl Pts',(-0.0268232619974109,0.00355649862073227,
-0.00558171480714852));
#53254=CARTESIAN_POINT('Ctrl Pts',(-0.0269828211829138,0.00305252022388036,
-0.00508905472630933));
#53255=CARTESIAN_POINT('Ctrl Pts',(-0.025861152465289,0.00386425555365813,
-0.00591958411161263));
#53256=CARTESIAN_POINT('Ctrl Pts',(-0.0261693159050445,0.00323236615942843,
-0.00571374798206362));
#53257=CARTESIAN_POINT('Ctrl Pts',(-0.0263470523169275,0.00272876851477799,
-0.00521258592314838));
#53258=CARTESIAN_POINT('Ctrl Pts',(-0.0250286088285531,0.0034052289470929,
-0.00610437205199126));
#53259=CARTESIAN_POINT('Ctrl Pts',(-0.0253626046700147,0.00278416555730594,
-0.00589816148590217));
#53260=CARTESIAN_POINT('Ctrl Pts',(-0.0255523751777655,0.00228207997173738,
-0.0053963585446636));
#53261=CARTESIAN_POINT('Ctrl Pts',(-0.0237145546648394,0.00263062411308175,
-0.00645442168636818));
#53262=CARTESIAN_POINT('Ctrl Pts',(-0.0240193050878441,0.00200028219795834,
-0.00626378438987051));
#53263=CARTESIAN_POINT('Ctrl Pts',(-0.024174135008249,0.00147561881341623,
-0.00578692718671447));
#53264=CARTESIAN_POINT('Ctrl Pts',(-0.0219731049140079,0.00187183481145798,
-0.0070682386857302));
#53265=CARTESIAN_POINT('Ctrl Pts',(-0.0221573770271123,0.00111225139363262,
-0.00692816079214065));
#53266=CARTESIAN_POINT('Ctrl Pts',(-0.0221889912973933,0.000481700437360768,
-0.00644789501881987));
#53267=CARTESIAN_POINT('Ctrl Pts',(-0.0196577522133193,0.00149257628269449,
-0.00806059618661361));
#53268=CARTESIAN_POINT('Ctrl Pts',(-0.01973610478976,0.00050921641839706,
-0.00798804692450031));
#53269=CARTESIAN_POINT('Ctrl Pts',(-0.0195902622436619,-0.000263255730683529,
-0.00738835747518616));
#53270=CARTESIAN_POINT('Ctrl Pts',(-0.0173546263616046,0.00138324422282633,
-0.00913020895521079));
#53271=CARTESIAN_POINT('Ctrl Pts',(-0.0173769785163834,0.000198590709853074,
-0.00910811698131738));
#53272=CARTESIAN_POINT('Ctrl Pts',(-0.0170772860700991,-0.00066260666126077,
-0.00835060388230459));
#53273=CARTESIAN_POINT('Ctrl Pts',(-0.0158446688321696,0.00138690879226211,
-0.00986871486838659));
#53274=CARTESIAN_POINT('Ctrl Pts',(-0.0158406071373422,8.7294300466045E-5,
-0.00987123115306857));
#53275=CARTESIAN_POINT('Ctrl Pts',(-0.0154232695854763,-0.000803047871763627,
-0.0090213459552702));
#53276=CARTESIAN_POINT('Ctrl Pts',(-0.0150619153852245,0.00140071328882223,
-0.0102593577757051));
#53277=CARTESIAN_POINT('Ctrl Pts',(-0.0150568244437027,4.45394858915551E-5,
-0.0102669524250396));
#53278=CARTESIAN_POINT('Ctrl Pts',(-0.0145987801442292,-0.000854777680999614,
-0.00936101918622224));
#53279=CARTESIAN_POINT('',(-0.0168559418075085,0.000684768142416315,-0.00927936853839009));
#53280=CARTESIAN_POINT('Ctrl Pts',(-0.0151728897383989,0.00139471190135993,
-0.0102040357394328));
#53281=CARTESIAN_POINT('Ctrl Pts',(-0.0151702322536255,0.00130488215101023,
-0.0102055148167351));
#53282=CARTESIAN_POINT('Ctrl Pts',(-0.015239223527948,0.00124141684161519,
-0.0101673535957409));
#53283=CARTESIAN_POINT('Ctrl Pts',(-0.015307419695405,0.00119164723569968,
-0.0101297968191818));
#53284=CARTESIAN_POINT('Ctrl Pts',(-0.0153756158628621,0.00114187762978418,
-0.0100922400426227));
#53285=CARTESIAN_POINT('Ctrl Pts',(-0.0154428915182541,0.0011058242963998,
-0.0100550351968635));
#53286=CARTESIAN_POINT('Ctrl Pts',(-0.0155132948332529,0.00107284990167657,
-0.0100162560632439));
#53287=CARTESIAN_POINT('Ctrl Pts',(-0.0155836981482517,0.00103987550695335,
-0.00997747692962429));
#53288=CARTESIAN_POINT('Ctrl Pts',(-0.0156571625546665,0.00100999302216499,
-0.00993698931508581));
#53289=CARTESIAN_POINT('Ctrl Pts',(-0.0157307971901185,0.000982771995278683,
-0.0098964483681575));
#53290=CARTESIAN_POINT('Ctrl Pts',(-0.0158044318255704,0.00095555096839237,
-0.00985590742122919));
#53291=CARTESIAN_POINT('Ctrl Pts',(-0.0158782380885874,0.000930990288587306,
-0.00981531602417939));
#53292=CARTESIAN_POINT('Ctrl Pts',(-0.0159524436492681,0.000907913501193525,
-0.00977452964654521));
#53293=CARTESIAN_POINT('Ctrl Pts',(-0.0161008547706294,0.000861759926405962,
-0.00969295689127685));
#53294=CARTESIAN_POINT('Ctrl Pts',(-0.0162508630387447,0.000821543067736549,
-0.00961060403861727));
#53295=CARTESIAN_POINT('Ctrl Pts',(-0.0164016269412466,0.000784896664753995,
-0.00952797982903137));
#53296=CARTESIAN_POINT('Ctrl Pts',(-0.0165523908437485,0.000748250261771441,
-0.00944535561944546));
#53297=CARTESIAN_POINT('Ctrl Pts',(-0.0167038987539332,0.000715179656409445,
-0.00936243640413805));
#53298=CARTESIAN_POINT('Ctrl Pts',(-0.0168559418075085,0.000684768142416308,
-0.00927936853839006));
#53299=CARTESIAN_POINT('',(-0.0184101558320655,0.000106937857928987,-0.00826148684386422));
#53300=CARTESIAN_POINT('Ctrl Pts',(-0.0168559106004127,0.000684785839446314,
-0.00927930493960189));
#53301=CARTESIAN_POINT('Ctrl Pts',(-0.0169994384641672,0.000656074616975346,
-0.00920091587798125));
#53302=CARTESIAN_POINT('Ctrl Pts',(-0.0171422855111684,0.000625624189261452,
-0.00912181819303145));
#53303=CARTESIAN_POINT('Ctrl Pts',(-0.0172838503930251,0.000592876796398921,
-0.00904172279456659));
#53304=CARTESIAN_POINT('Ctrl Pts',(-0.0172953475013133,0.000590217236224398,
-0.00903521789407531));
#53305=CARTESIAN_POINT('Ctrl Pts',(-0.0173068366582681,0.000587541830465944,
-0.00902870590106529));
#53306=CARTESIAN_POINT('Ctrl Pts',(-0.0173183167955872,0.000584850350612705,
-0.00902218702064899));
#53307=CARTESIAN_POINT('Ctrl Pts',(-0.0174481925751245,0.000554401407857755,
-0.0089484383665829));
#53308=CARTESIAN_POINT('Ctrl Pts',(-0.0175769158543567,0.000521907202193238,
-0.00887381668562478));
#53309=CARTESIAN_POINT('Ctrl Pts',(-0.0177038524404219,0.000486178880005269,
-0.00879763432014667));
#53310=CARTESIAN_POINT('Ctrl Pts',(-0.0177226207864461,0.000480896230341577,
-0.00878637029422195));
#53311=CARTESIAN_POINT('Ctrl Pts',(-0.0177413352367826,0.000475534680172062,
-0.00877507626560524));
#53312=CARTESIAN_POINT('Ctrl Pts',(-0.017760009234808,0.000470092158801244,
-0.00876374276261054));
#53313=CARTESIAN_POINT('Ctrl Pts',(-0.0178100664404382,0.000455503027377121,
-0.00873336236473615));
#53314=CARTESIAN_POINT('Ctrl Pts',(-0.0178598386157251,0.000440337954000094,
-0.00870269839544443));
#53315=CARTESIAN_POINT('Ctrl Pts',(-0.017909104476756,0.000424382586793304,
-0.00867169456780072));
#53316=CARTESIAN_POINT('Ctrl Pts',(-0.0179767491222203,0.000402475019659202,
-0.00862912466472574));
#53317=CARTESIAN_POINT('Ctrl Pts',(-0.0180435462459668,0.000379119629529094,
-0.00858589778545374));
#53318=CARTESIAN_POINT('Ctrl Pts',(-0.0181099233481851,0.000352507988189935,
-0.00854072977249054));
#53319=CARTESIAN_POINT('Ctrl Pts',(-0.0181289719923642,0.000344871082239675,
-0.008527767630751));
#53320=CARTESIAN_POINT('Ctrl Pts',(-0.0181478033724562,0.000337023540513838,
-0.00851476104835145));
#53321=CARTESIAN_POINT('Ctrl Pts',(-0.0181663678145007,0.00032895373681883,
-0.00850172329166989));
#53322=CARTESIAN_POINT('Ctrl Pts',(-0.0182124932189159,0.000308903419222881,
-0.00846932954678046));
#53323=CARTESIAN_POINT('Ctrl Pts',(-0.0182569831984907,0.000287497097208199,
-0.00843674620973055));
#53324=CARTESIAN_POINT('Ctrl Pts',(-0.0182974687017753,0.000262756868223345,
-0.00840386569127419));
#53325=CARTESIAN_POINT('Ctrl Pts',(-0.0183104033003802,0.00025485268264208,
-0.00839336078770008));
#53326=CARTESIAN_POINT('Ctrl Pts',(-0.0183233624796087,0.000246284839621537,
-0.00838244445279732));
#53327=CARTESIAN_POINT('Ctrl Pts',(-0.0183361960489214,0.000236921585224982,
-0.00837109800055212));
#53328=CARTESIAN_POINT('Ctrl Pts',(-0.0183515307372761,0.000225733537328151,
-0.00835754025173936));
#53329=CARTESIAN_POINT('Ctrl Pts',(-0.0183667534635429,0.000213411283286992,
-0.00834333641976299));
#53330=CARTESIAN_POINT('Ctrl Pts',(-0.0183798354311663,0.000199713718176209,
-0.00832931041010002));
#53331=CARTESIAN_POINT('Ctrl Pts',(-0.0184038656707308,0.000174552688846439,
-0.00830354606164427));
#53332=CARTESIAN_POINT('Ctrl Pts',(-0.0184222097745657,0.000144872070237118,
-0.00827771743599519));
#53333=CARTESIAN_POINT('Ctrl Pts',(-0.0184101558320613,0.000106937857930527,
-0.00826148684386729));
#53334=CARTESIAN_POINT('Ctrl Pts',(-0.0184101558320655,0.000106937857928987,
-0.00826148684386422));
#53335=CARTESIAN_POINT('Ctrl Pts',(-0.0191899749903914,0.00010230128487336,
-0.00785918081542734));
#53336=CARTESIAN_POINT('Ctrl Pts',(-0.0199660898324893,9.51225642974071E-5,
-0.00744873103086231));
#53337=CARTESIAN_POINT('Ctrl Pts',(-0.0207149455884367,8.43554830514994E-5,
-0.00699117714319491));
#53338=CARTESIAN_POINT('Ctrl Pts',(-0.0328171226457405,0.00544959479189026,
-0.00491819444776802));
#53339=CARTESIAN_POINT('Ctrl Pts',(-0.0328195640571706,0.00498233590672909,
-0.00477513152938287));
#53340=CARTESIAN_POINT('Ctrl Pts',(-0.0328127292790594,0.00455105192850437,
-0.00451607286816002));
#53341=CARTESIAN_POINT('Ctrl Pts',(-0.0327968763129483,0.00420555010966588,
-0.0041712068084503));
#53342=CARTESIAN_POINT('Origin',(-0.034273100524039,0.0063892955694362,
-0.00193093091927896));
#53343=CARTESIAN_POINT('Ctrl Pts',(-0.0337145948616341,0.00415833566999661,
0.00401503462776478));
#53344=CARTESIAN_POINT('Ctrl Pts',(-0.0337504898950536,0.00448210638016595,
0.00435737005883901));
#53345=CARTESIAN_POINT('Ctrl Pts',(-0.0337798713312579,0.00488841094225288,
0.00462212049130278));
#53346=CARTESIAN_POINT('Ctrl Pts',(-0.0337993965723764,0.00533366251113205,
0.00478061601362495));
#53347=CARTESIAN_POINT('Ctrl Pts',(-0.0326387926265156,0.00424057900937983,
0.00419929895082685));
#53348=CARTESIAN_POINT('Ctrl Pts',(-0.0326521120878623,0.00459856815265706,
0.0045522680694765));
#53349=CARTESIAN_POINT('Ctrl Pts',(-0.0326523815453445,0.00504644076338797,
0.00481398643458415));
#53350=CARTESIAN_POINT('Ctrl Pts',(-0.0326395047684778,0.00552995296452442,
0.00495256740652356));
#53351=CARTESIAN_POINT('Ctrl Pts',(-0.0307995994291534,0.00425190175201537,
0.004505296988018));
#53352=CARTESIAN_POINT('Ctrl Pts',(-0.0307898334715919,0.00462109727731803,
0.00482527566892104));
#53353=CARTESIAN_POINT('Ctrl Pts',(-0.0307597745982798,0.00506856871463487,
0.00505436659406124));
#53354=CARTESIAN_POINT('Ctrl Pts',(-0.0307129201916643,0.00554291348277156,
0.00516623054628213));
#53355=CARTESIAN_POINT('Ctrl Pts',(-0.0284413845216665,0.00372335549694271,
0.00483605952326099));
#53356=CARTESIAN_POINT('Ctrl Pts',(-0.0283698180551898,0.00408268647934982,
0.00516184559608916));
#53357=CARTESIAN_POINT('Ctrl Pts',(-0.0282601549337502,0.00451602599614115,
0.00539830518908961));
#53358=CARTESIAN_POINT('Ctrl Pts',(-0.0281250818282017,0.00497353878031065,
0.00551806473009416));
#53359=CARTESIAN_POINT('Ctrl Pts',(-0.026503416926424,0.00285775025295423,
0.00515034561794722));
#53360=CARTESIAN_POINT('Ctrl Pts',(-0.0263806195395379,0.00317751670560064,
0.00547519490900795));
#53361=CARTESIAN_POINT('Ctrl Pts',(-0.0262066562740293,0.0035592412880712,
0.00571951320274019));
#53362=CARTESIAN_POINT('Ctrl Pts',(-0.0260003497552778,0.0039618848035107,
0.00585689946815495));
#53363=CARTESIAN_POINT('Ctrl Pts',(-0.0245731919014548,0.00166880228110552,
0.00564722242151088));
#53364=CARTESIAN_POINT('Ctrl Pts',(-0.0244513567483743,0.00199858974938907,
0.0059608556267388));
#53365=CARTESIAN_POINT('Ctrl Pts',(-0.0242720553711055,0.00238236582209498,
0.00619499515250578));
#53366=CARTESIAN_POINT('Ctrl Pts',(-0.0240543129347437,0.00277916645442249,
0.00632454923114672));
#53367=CARTESIAN_POINT('Ctrl Pts',(-0.0221706253086404,0.00046612601988525,
0.00645018290437898));
#53368=CARTESIAN_POINT('Ctrl Pts',(-0.0221581341038569,0.000880257985322814,
0.00675728529047529));
#53369=CARTESIAN_POINT('Ctrl Pts',(-0.0220849415751972,0.00136253175593733,
0.00696991151781838));
#53370=CARTESIAN_POINT('Ctrl Pts',(-0.0219616170038293,0.00185499085047183,
0.00706158768923822));
#53371=CARTESIAN_POINT('Ctrl Pts',(-0.0195701738987167,-0.000266550805092657,
0.00739523959835644));
#53372=CARTESIAN_POINT('Ctrl Pts',(-0.0196760856193404,0.000234542108405088,
0.00777465949313878));
#53373=CARTESIAN_POINT('Ctrl Pts',(-0.0197001203513376,0.000858128190769441,
0.00801082445085077));
#53374=CARTESIAN_POINT('Ctrl Pts',(-0.0196397060603481,0.0014900587499245,
0.00805989029189566));
#53375=CARTESIAN_POINT('Ctrl Pts',(-0.0167705697451759,-0.000704592537367574,
0.00847417313657492));
#53376=CARTESIAN_POINT('Ctrl Pts',(-0.0169829836419465,-0.000149778270697148,
0.00895736442962707));
#53377=CARTESIAN_POINT('Ctrl Pts',(-0.0170929548817286,0.000609089429017907,
0.00924272341216823));
#53378=CARTESIAN_POINT('Ctrl Pts',(-0.0170734273265382,0.00137323317849824,
0.00925507608132262));
#53379=CARTESIAN_POINT('Ctrl Pts',(-0.0148407380900652,-0.000839331357905782,
0.00927002324422269));
#53380=CARTESIAN_POINT('Ctrl Pts',(-0.015129397707141,-0.000273240055481486,
0.00981783425117302));
#53381=CARTESIAN_POINT('Ctrl Pts',(-0.0153048081511204,0.000560629512514839,
0.0101375931190703));
#53382=CARTESIAN_POINT('Ctrl Pts',(-0.015311716611075,0.00139891690278659,
0.0101278799490686));
#53383=CARTESIAN_POINT('Ctrl Pts',(-0.0137268720321833,-0.000892677918735118,
0.00973665336335839));
#53384=CARTESIAN_POINT('Ctrl Pts',(-0.0140290905698997,-0.000325814591128036,
0.0103371273983254));
#53385=CARTESIAN_POINT('Ctrl Pts',(-0.0142143926766274,0.000548607912082809,
0.0106939538304117));
#53386=CARTESIAN_POINT('Ctrl Pts',(-0.0142179384615059,0.00142799346296082,
0.0106828353729555));
#53387=CARTESIAN_POINT('',(-0.0184512676916217,0.000107246345742279,0.00823734004344498));
#53388=CARTESIAN_POINT('Ctrl Pts',(-0.0207569019187454,8.46249604678063E-5,
0.00696635255655076));
#53389=CARTESIAN_POINT('Ctrl Pts',(-0.0200077628358915,9.54352636376166E-5,
0.00742407896483524));
#53390=CARTESIAN_POINT('Ctrl Pts',(-0.0192312828839955,0.000102624232462172,
0.00783467988302133));
#53391=CARTESIAN_POINT('Ctrl Pts',(-0.0184512581841375,0.000107246022242465,
0.0082373457726289));
#53392=CARTESIAN_POINT('',(-0.0168949674403344,0.000683552764475077,0.00925478469399231));
#53393=CARTESIAN_POINT('Ctrl Pts',(-0.0184512676916217,0.000107246345742279,
0.00823734004344498));
#53394=CARTESIAN_POINT('Ctrl Pts',(-0.0184622301433659,0.000141599751249758,
0.00825191867407648));
#53395=CARTESIAN_POINT('Ctrl Pts',(-0.0184456858101158,0.000172716967409295,
0.00827767057001621));
#53396=CARTESIAN_POINT('Ctrl Pts',(-0.018421873317597,0.000198254458454251,
0.00830351846934873));
#53397=CARTESIAN_POINT('Ctrl Pts',(-0.0184104929975665,0.00021045917917544,
0.0083158715384904));
#53398=CARTESIAN_POINT('Ctrl Pts',(-0.0183975628351906,0.000221439064276058,
0.00832822607534285));
#53399=CARTESIAN_POINT('Ctrl Pts',(-0.0183844216172855,0.000231486145171871,
0.00834010980452181));
#53400=CARTESIAN_POINT('Ctrl Pts',(-0.0183700657918549,0.000242461850808103,
0.00835309191491602));
#53401=CARTESIAN_POINT('Ctrl Pts',(-0.01835540146337,0.000252330125039528,
0.00836554321037133));
#53402=CARTESIAN_POINT('Ctrl Pts',(-0.0183404924684894,0.000261530264194091,
0.00837769350203077));
#53403=CARTESIAN_POINT('Ctrl Pts',(-0.0183019237969097,0.000285330469934476,
0.00840912557457252));
#53404=CARTESIAN_POINT('Ctrl Pts',(-0.0182596528414629,0.000305730744391114,
0.00844011593411856));
#53405=CARTESIAN_POINT('Ctrl Pts',(-0.0182160609702212,0.000324884503226279,
0.00847085444561481));
#53406=CARTESIAN_POINT('Ctrl Pts',(-0.0181951012398468,0.000334093963829995,
0.00848563405692127));
#53407=CARTESIAN_POINT('Ctrl Pts',(-0.0181738267201503,0.000343006968918949,
0.00850035502957633));
#53408=CARTESIAN_POINT('Ctrl Pts',(-0.0181522729621096,0.000351651856950548,
0.00851502182610127));
#53409=CARTESIAN_POINT('Ctrl Pts',(-0.018085891879075,0.000378276310522332,
0.00856019250288709));
#53410=CARTESIAN_POINT('Ctrl Pts',(-0.0180189689159113,0.000401641369382736,
0.00860349488247737));
#53411=CARTESIAN_POINT('Ctrl Pts',(-0.0179511291677144,0.000423553630764221,
0.00864618006740678));
#53412=CARTESIAN_POINT('Ctrl Pts',(-0.0179036725263837,0.000438882141803327,
0.00867604007669589));
#53413=CARTESIAN_POINT('Ctrl Pts',(-0.0178557140104046,0.000453480053782304,
0.00870560687033));
#53414=CARTESIAN_POINT('Ctrl Pts',(-0.017807482880896,0.000467540968088816,
0.00873491305520521));
#53415=CARTESIAN_POINT('Ctrl Pts',(-0.0177867671235334,0.000473580272829081,
0.0087475003576649));
#53416=CARTESIAN_POINT('Ctrl Pts',(-0.0177660002240907,0.000479519756530131,
0.0087600396106193));
#53417=CARTESIAN_POINT('Ctrl Pts',(-0.0177451711391999,0.000485363451470148,
0.00877254070523275));
#53418=CARTESIAN_POINT('Ctrl Pts',(-0.0176186513664753,0.000520859151812222,
0.00884847470125778));
#53419=CARTESIAN_POINT('Ctrl Pts',(-0.0174903687188125,0.000553070032504836,
0.00892284009755575));
#53420=CARTESIAN_POINT('Ctrl Pts',(-0.0173611017027544,0.000583240788244276,
0.00899628311459254));
#53421=CARTESIAN_POINT('Ctrl Pts',(-0.017348709986102,0.000586132999016321,
0.0090033234647528));
#53422=CARTESIAN_POINT('Ctrl Pts',(-0.0173363090600306,0.000589006309522193,
0.00901035529404749));
#53423=CARTESIAN_POINT('Ctrl Pts',(-0.0173238992320563,0.000591861210441433,
0.00901737890518302));
#53424=CARTESIAN_POINT('Ctrl Pts',(-0.017182033455642,0.000624497660868489,
0.00909767091640441));
#53425=CARTESIAN_POINT('Ctrl Pts',(-0.0170390390744304,0.000654793151863181,
0.00917689686737658));
#53426=CARTESIAN_POINT('Ctrl Pts',(-0.0168953032845727,0.000683360688020473,
0.00925546810437223));
#53427=CARTESIAN_POINT('Ctrl Pts',(-0.0168945268806226,0.000683804758467406,
0.00925388800048686));
#53428=CARTESIAN_POINT('Ctrl Pts',(-0.0167416908614446,0.000714147179609983,
0.00933751330057378));
#53429=CARTESIAN_POINT('Ctrl Pts',(-0.0165893391680148,0.000747133161909586,
0.00942105041880093));
#53430=CARTESIAN_POINT('Ctrl Pts',(-0.0164377067953043,0.000783648753803687,
0.00950434172638755));
#53431=CARTESIAN_POINT('Ctrl Pts',(-0.0162860744225938,0.000820164345697787,
0.00958763303397418));
#53432=CARTESIAN_POINT('Ctrl Pts',(-0.016135172427679,0.000860204085166195,
0.00967070099051174));
#53433=CARTESIAN_POINT('Ctrl Pts',(-0.0159861906776217,0.00090600098099338,
0.0097528594815456));
#53434=CARTESIAN_POINT('Ctrl Pts',(-0.015911699802593,0.000928899428906973,
0.00979393872706254));
#53435=CARTESIAN_POINT('Ctrl Pts',(-0.0158376888222992,0.000953237109203088,
0.00983479027696665));
#53436=CARTESIAN_POINT('Ctrl Pts',(-0.0157637840768862,0.000980108361912485,
0.0098756285401895));
#53437=CARTESIAN_POINT('Ctrl Pts',(-0.0156898793314732,0.00100697961462188,
0.00991646680341235));
#53438=CARTESIAN_POINT('Ctrl Pts',(-0.0156160814995489,0.0010363844824535,
0.00995729312691053));
#53439=CARTESIAN_POINT('Ctrl Pts',(-0.0155451624184428,0.00106910118935474,
0.00999654935387522));
#53440=CARTESIAN_POINT('Ctrl Pts',(-0.0154742433373368,0.00110181789625599,
0.0100358055808399));
#53441=CARTESIAN_POINT('Ctrl Pts',(-0.0154062607310772,0.00113783598555345,
0.0100736076277172));
#53442=CARTESIAN_POINT('Ctrl Pts',(-0.0153367057996425,0.0011864783152364,
0.0101120703301702));
#53443=CARTESIAN_POINT('Ctrl Pts',(-0.0152671508682078,0.00123512064491935,
0.0101505330326231));
#53444=CARTESIAN_POINT('Ctrl Pts',(-0.0151962210891276,0.00129636052306388,
0.010190052413572));
#53445=CARTESIAN_POINT('Ctrl Pts',(-0.0151955011741265,0.00138726386004148,
0.010190435150715));
#53446=CARTESIAN_POINT('Ctrl Pts',(-0.0328029017533461,0.00420876907691088,
0.00416971954492692));
#53447=CARTESIAN_POINT('Ctrl Pts',(-0.0328178241773457,0.00455258395424896,
0.00451249633250882));
#53448=CARTESIAN_POINT('Ctrl Pts',(-0.032824617798705,0.00498124122173345,
0.00477032439575802));
#53449=CARTESIAN_POINT('Ctrl Pts',(-0.0328230352836128,0.00544566811076568,
0.00491342087848278));
#53450=CARTESIAN_POINT('Origin',(-0.034735005000479,0.00640255695754379,
0.00190578554004708));
#53451=CARTESIAN_POINT('Origin',(-0.0319546402921759,0.00870364387463654,
0.00212141796726865));
#53452=CARTESIAN_POINT('Ctrl Pts',(-0.0312397316818193,0.00944581611174232,
0.00513213161553135));
#53453=CARTESIAN_POINT('Ctrl Pts',(-0.0312427451291909,0.0099961712863933,
0.00499938556413842));
#53454=CARTESIAN_POINT('Ctrl Pts',(-0.0312280639560642,0.0105069403051091,
0.0047080293508316));
#53455=CARTESIAN_POINT('Ctrl Pts',(-0.0311964657406625,0.0109004375755286,
0.00430330249027805));
#53456=CARTESIAN_POINT('Ctrl Pts',(-0.0311915498707958,0.0109616556332477,
0.00424033739706811));
#53457=CARTESIAN_POINT('Ctrl Pts',(-0.0311862383752956,0.0110200907724982,
0.00417471052484215));
#53458=CARTESIAN_POINT('Ctrl Pts',(-0.0311805498203867,0.0110755139672511,
0.00410668511418156));
#53459=CARTESIAN_POINT('Ctrl Pts',(-0.0323289055074392,0.00956463425415454,
0.00496775823408284));
#53460=CARTESIAN_POINT('Ctrl Pts',(-0.0322835345259748,0.0105323987449126,
0.00469073673727539));
#53461=CARTESIAN_POINT('Ctrl Pts',(-0.0321832620259936,0.0111351594703581,
0.0038896157471382));
#53462=CARTESIAN_POINT('Ctrl Pts',(-0.0312200346161952,0.00937861982895493,
0.005143320519133));
#53463=CARTESIAN_POINT('Ctrl Pts',(-0.0312346609291161,0.010392145765573,
0.00491292268688717));
#53464=CARTESIAN_POINT('Ctrl Pts',(-0.0311666295055617,0.0110485670062122,
0.00411075495197673));
#53465=CARTESIAN_POINT('Ctrl Pts',(-0.0297913603172275,0.00936877543822054,
0.00533931757967592));
#53466=CARTESIAN_POINT('Ctrl Pts',(-0.0298729635552801,0.010373653877553,
0.00514091880759088));
#53467=CARTESIAN_POINT('Ctrl Pts',(-0.0298366841122876,0.0110548585358543,
0.00437421338280484));
#53468=CARTESIAN_POINT('Ctrl Pts',(-0.0282450431755874,0.00956902209544001,
0.00560006763975001));
#53469=CARTESIAN_POINT('Ctrl Pts',(-0.0283949818456436,0.0105482847054643,
0.00541290036078366));
#53470=CARTESIAN_POINT('Ctrl Pts',(-0.028395990827051,0.0112342387571675,
0.00467417110487153));
#53471=CARTESIAN_POINT('Ctrl Pts',(-0.0275655213410194,0.00968883811290509,
0.00572471869657096));
#53472=CARTESIAN_POINT('Ctrl Pts',(-0.0277376631422493,0.0106490933625841,
0.00554219914270759));
#53473=CARTESIAN_POINT('Ctrl Pts',(-0.0277512049297973,0.0113334753293838,
0.00482364841791884));
#53474=CARTESIAN_POINT('Ctrl Pts',(-0.0265559503873459,0.00990413801644446,
0.00591995560007617));
#53475=CARTESIAN_POINT('Ctrl Pts',(-0.0267967998478078,0.0108655812357791,
0.00572891428999259));
#53476=CARTESIAN_POINT('Ctrl Pts',(-0.0268463635570509,0.0115505484415826,
0.0049905610344629));
#53477=CARTESIAN_POINT('Ctrl Pts',(-0.0254134410921188,0.0102924262124582,
0.00616699453409525));
#53478=CARTESIAN_POINT('Ctrl Pts',(-0.0257285874563407,0.0112136516860456,
0.00595948028213227));
#53479=CARTESIAN_POINT('Ctrl Pts',(-0.0258174256338695,0.0118799491673231,
0.0052256231497365));
#53480=CARTESIAN_POINT('Ctrl Pts',(-0.0241333918107377,0.0108163472585975,
0.0065002849396036));
#53481=CARTESIAN_POINT('Ctrl Pts',(-0.0244436384112718,0.0117250628952979,
0.00629519856091718));
#53482=CARTESIAN_POINT('Ctrl Pts',(-0.0245157153622336,0.012395142022738,
0.00558085893470258));
#53483=CARTESIAN_POINT('Ctrl Pts',(-0.0228483409677525,0.0112659510356338,
0.00688891895195866));
#53484=CARTESIAN_POINT('Ctrl Pts',(-0.0230856742818988,0.0122441558971299,
0.00670982953098516));
#53485=CARTESIAN_POINT('Ctrl Pts',(-0.0230700961407223,0.0129638411427807,
0.00598451454320165));
#53486=CARTESIAN_POINT('Ctrl Pts',(-0.0212004840786695,0.0115773550466138,
0.00748986583980058));
#53487=CARTESIAN_POINT('Ctrl Pts',(-0.0213153046899869,0.0127481902765968,
0.0073719420427496));
#53488=CARTESIAN_POINT('Ctrl Pts',(-0.021136532193506,0.0135629220950769,
0.00653554204472973));
#53489=CARTESIAN_POINT('Ctrl Pts',(-0.019167042709017,0.0116660893942,0.0083356198639276));
#53490=CARTESIAN_POINT('Ctrl Pts',(-0.0191804598076967,0.0130869110402204,
0.00829326114742038));
#53491=CARTESIAN_POINT('Ctrl Pts',(-0.0187900587222371,0.0139677007175143,
0.00724790416315883));
#53492=CARTESIAN_POINT('Ctrl Pts',(-0.0174670465709295,0.0116196738300899,
0.00910191951123781));
#53493=CARTESIAN_POINT('Ctrl Pts',(-0.0174262819740025,0.0132365547392771,
0.00910993735381814));
#53494=CARTESIAN_POINT('Ctrl Pts',(-0.0168589854819659,0.0141212857391936,
0.00788011740047476));
#53495=CARTESIAN_POINT('Ctrl Pts',(-0.0158059579855905,0.0115214530689453,
0.00988765845793635));
#53496=CARTESIAN_POINT('Ctrl Pts',(-0.0157056048103155,0.0133294903173838,
0.00994296969637082));
#53497=CARTESIAN_POINT('Ctrl Pts',(-0.0149832859165724,0.0141820295951835,
0.00851735457057802));
#53498=CARTESIAN_POINT('Ctrl Pts',(-0.0148654266643081,0.0114297302076929,
0.010351940251372));
#53499=CARTESIAN_POINT('Ctrl Pts',(-0.0147095818741422,0.013367376733051,
0.0104450157835826));
#53500=CARTESIAN_POINT('Ctrl Pts',(-0.0138532836292959,0.0141734567758274,
0.0088943488081759));
#53501=CARTESIAN_POINT('Ctrl Pts',(-0.0141214309450543,0.0113497268442424,
0.010725020327289));
#53502=CARTESIAN_POINT('Ctrl Pts',(-0.013953871480134,0.0133905329094632,
0.0108226494532548));
#53503=CARTESIAN_POINT('Ctrl Pts',(-0.0130838251198689,0.0141473730896605,
0.00912716600625515));
#53504=CARTESIAN_POINT('',(-0.0177980642249198,0.0125583362975071,0.00878211032055315));
#53505=CARTESIAN_POINT('Ctrl Pts',(-0.0152016054147685,0.0114763663362328,
0.0101879079879127));
#53506=CARTESIAN_POINT('Ctrl Pts',(-0.0152050402282475,0.0115448524639896,
0.0101862046141003));
#53507=CARTESIAN_POINT('Ctrl Pts',(-0.015246578657923,0.0115988404990711,
0.01016347688237));
#53508=CARTESIAN_POINT('Ctrl Pts',(-0.0152916884420663,0.0116441867557964,
0.0101388600044451));
#53509=CARTESIAN_POINT('Ctrl Pts',(-0.0153367982262096,0.0116895330125218,
0.0101142431265201));
#53510=CARTESIAN_POINT('Ctrl Pts',(-0.01538541673375,0.0117262297566457,
0.0100876082435883));
#53511=CARTESIAN_POINT('Ctrl Pts',(-0.0154357715420465,0.0117599086203434,
0.0100600660888032));
#53512=CARTESIAN_POINT('Ctrl Pts',(-0.0155364811586393,0.0118272663477389,
0.0100049817792332));
#53513=CARTESIAN_POINT('Ctrl Pts',(-0.0156440742586175,0.0118825435032204,
0.0099461410209836));
#53514=CARTESIAN_POINT('Ctrl Pts',(-0.0157531598918773,0.0119329055094452,
0.00988663924228184));
#53515=CARTESIAN_POINT('Ctrl Pts',(-0.015857875517086,0.0119812499963496,
0.00982952112533473));
#53516=CARTESIAN_POINT('Ctrl Pts',(-0.0159639163376693,0.0120250494639677,
0.00977169149544583));
#53517=CARTESIAN_POINT('Ctrl Pts',(-0.0160709107474822,0.0120659590805672,
0.00971346327977728));
#53518=CARTESIAN_POINT('Ctrl Pts',(-0.0160753758541115,0.0120676663267738,
0.00971103329121761));
#53519=CARTESIAN_POINT('Ctrl Pts',(-0.0160798426028328,0.012069368537373,
0.00970860256749819));
#53520=CARTESIAN_POINT('Ctrl Pts',(-0.0160843109022008,0.0120710658302876,
0.00970617114887469));
#53521=CARTESIAN_POINT('Ctrl Pts',(-0.0161958501168776,0.012113434235619,
0.00964547724690497));
#53522=CARTESIAN_POINT('Ctrl Pts',(-0.0163083952064916,0.0121527396216367,
0.00958434693869943));
#53523=CARTESIAN_POINT('Ctrl Pts',(-0.0164214891938709,0.012189946046317,
0.00952302377047061));
#53524=CARTESIAN_POINT('Ctrl Pts',(-0.0166343834177911,0.0122599854276378,
0.00940758572985573));
#53525=CARTESIAN_POINT('Ctrl Pts',(-0.0168492373888548,0.0123225837024365,
0.00929147343309498));
#53526=CARTESIAN_POINT('Ctrl Pts',(-0.0170652210318034,0.0123803691306557,
0.00917518725110595));
#53527=CARTESIAN_POINT('Ctrl Pts',(-0.0170787076951882,0.0123839774252853,
0.00916792599478407));
#53528=CARTESIAN_POINT('Ctrl Pts',(-0.0170921988550825,0.0123875667820013,
0.00916066382123329));
#53529=CARTESIAN_POINT('Ctrl Pts',(-0.0171056945549107,0.0123911377037813,
0.0091534006632344));
#53530=CARTESIAN_POINT('Ctrl Pts',(-0.0173353186127975,0.0124518955422013,
0.00902982086863233));
#53531=CARTESIAN_POINT('Ctrl Pts',(-0.0175661531830874,0.0125073758986016,
0.00890601385220129));
#53532=CARTESIAN_POINT('Ctrl Pts',(-0.0177980683695447,0.0125583397025061,
0.0087821194794289));
#53533=CARTESIAN_POINT('',(-0.0197685317455456,0.0133197512836476,0.00744191810867941));
#53534=CARTESIAN_POINT('Ctrl Pts',(-0.0177980642249198,0.0125583362975071,
0.00878211032055315));
#53535=CARTESIAN_POINT('Ctrl Pts',(-0.0179830006717361,0.0125989757247538,
0.00868331054782076));
#53536=CARTESIAN_POINT('Ctrl Pts',(-0.0181668800802558,0.0126419851714326,
0.00858330934992592));
#53537=CARTESIAN_POINT('Ctrl Pts',(-0.0183486946939373,0.0126879577019625,
0.00848144524952353));
#53538=CARTESIAN_POINT('Ctrl Pts',(-0.0183653017055318,0.0126921568492812,
0.00847214094629841));
#53539=CARTESIAN_POINT('Ctrl Pts',(-0.0183818925050772,0.0126963819437408,
0.00846281999090755));
#53540=CARTESIAN_POINT('Ctrl Pts',(-0.0183984647163266,0.0127006332497774,
0.00845348258635921));
#53541=CARTESIAN_POINT('Ctrl Pts',(-0.0185633261223776,0.0127429255112143,
0.00836059349512425));
#53542=CARTESIAN_POINT('Ctrl Pts',(-0.0187263554908639,0.0127877966895147,
0.00826609507339865));
#53543=CARTESIAN_POINT('Ctrl Pts',(-0.0188865527000641,0.0128364005614957,
0.00816870025540869));
#53544=CARTESIAN_POINT('Ctrl Pts',(-0.0189126820926947,0.0128443282255337,
0.00815281441412496));
#53545=CARTESIAN_POINT('Ctrl Pts',(-0.0189387119608945,0.0128523658573526,
0.00813685671555506));
#53546=CARTESIAN_POINT('Ctrl Pts',(-0.0189646627927476,0.0128605170269426,
0.00812081022830822));
#53547=CARTESIAN_POINT('Ctrl Pts',(-0.0190262598499789,0.0128798646941995,
0.00808272218554736));
#53548=CARTESIAN_POINT('Ctrl Pts',(-0.0190874192852412,0.0128998465199453,
0.00804413453101425));
#53549=CARTESIAN_POINT('Ctrl Pts',(-0.0191478356195508,0.0129206632446099,
0.00800493934770974));
#53550=CARTESIAN_POINT('Ctrl Pts',(-0.0192337053473069,0.0129502500525509,
0.0079492312389976));
#53551=CARTESIAN_POINT('Ctrl Pts',(-0.0193182418693047,0.0129814734970053,
0.0078922852084602));
#53552=CARTESIAN_POINT('Ctrl Pts',(-0.0194019483291107,0.0130164329880073,
0.0078320587920224));
#53553=CARTESIAN_POINT('Ctrl Pts',(-0.0194269273356376,0.0130268653173155,
0.00781408651063836));
#53554=CARTESIAN_POINT('Ctrl Pts',(-0.0194515537016336,0.0130375426930232,
0.00779600101439142));
#53555=CARTESIAN_POINT('Ctrl Pts',(-0.019475745499314,0.0130484770573286,
0.00777781862192818));
#53556=CARTESIAN_POINT('Ctrl Pts',(-0.0195326221675865,0.0130741845396575,
0.00773507050051131));
#53557=CARTESIAN_POINT('Ctrl Pts',(-0.0195871070281101,0.0131012997696144,
0.00769179228940438));
#53558=CARTESIAN_POINT('Ctrl Pts',(-0.0196364499341613,0.0131318484117174,
0.00764734735079382));
#53559=CARTESIAN_POINT('Ctrl Pts',(-0.0196529910828398,0.0131420891873707,
0.00763244814042303));
#53560=CARTESIAN_POINT('Ctrl Pts',(-0.019668874008655,0.0131526812624034,
0.00761748454393024));
#53561=CARTESIAN_POINT('Ctrl Pts',(-0.0196847074254495,0.0131642647987755,
0.00760167899627938));
#53562=CARTESIAN_POINT('Ctrl Pts',(-0.0197025345823486,0.0131773069313128,
0.00758388321779995));
#53563=CARTESIAN_POINT('Ctrl Pts',(-0.0197204841177018,0.0131915916001444,
0.00756495057568836));
#53564=CARTESIAN_POINT('Ctrl Pts',(-0.0197365286335694,0.013208312962062,
0.00754479399121415));
#53565=CARTESIAN_POINT('Ctrl Pts',(-0.0197668232558055,0.0132398855783219,
0.00750673512317151));
#53566=CARTESIAN_POINT('Ctrl Pts',(-0.0197875780156799,0.0132754871342319,
0.00746915089349625));
#53567=CARTESIAN_POINT('Ctrl Pts',(-0.0197684666960677,0.0133196392804432,
0.00744178318769348));
#53568=CARTESIAN_POINT('Ctrl Pts',(-0.0197685329350908,0.0133197531415193,
0.00744192027110921));
#53569=CARTESIAN_POINT('Ctrl Pts',(-0.0202415101381015,0.0133224462394573,
0.00721107381044522));
#53570=CARTESIAN_POINT('Ctrl Pts',(-0.0207109595596229,0.0133260249537321,
0.00697296703985871));
#53571=CARTESIAN_POINT('Ctrl Pts',(-0.0211704028999606,0.0133306505564277,
0.00671687894543797));
#53572=CARTESIAN_POINT('Ctrl Pts',(-0.0213774769702589,0.0133327353453313,
0.00660145839319391));
#53573=CARTESIAN_POINT('Ctrl Pts',(-0.0215825720015505,0.0133348962657808,
0.0064823124554158));
#53574=CARTESIAN_POINT('Ctrl Pts',(-0.0217846042317191,0.0133372723154647,
0.0063580695368299));
#53575=CARTESIAN_POINT('Origin',(0.,0.0012,0.));
#53576=CARTESIAN_POINT('Origin',(0.00625,0.0012,-0.0110556546617557));
#53577=CARTESIAN_POINT('Origin',(-0.000371408500209017,0.0012,-0.0126945679613751));
#53578=CARTESIAN_POINT('Origin',(-0.000359710594690623,0.0012,-0.0122947390492059));
#53579=CARTESIAN_POINT('Origin',(-0.000359710594690623,0.0012,-0.0122947390492059));
#53580=CARTESIAN_POINT('Origin',(-0.000492372526715892,0.0012,-0.0126720993701079));
#53581=CARTESIAN_POINT('Origin',(-0.000359710594690623,0.013,-0.0122947390492059));
#53582=CARTESIAN_POINT('Origin',(-0.000359710594690623,0.0128,-0.0122947390492059));
#53583=CARTESIAN_POINT('Origin',(0.00396253460616978,0.0012,0.));
#53584=CARTESIAN_POINT('Ctrl Pts',(-0.00872901544041542,0.001,-0.00439918826870922));
#53585=CARTESIAN_POINT('Ctrl Pts',(-0.0087111501862006,0.000999999999999996,
-0.00439284638245222));
#53586=CARTESIAN_POINT('Ctrl Pts',(-0.00869279015334147,0.00100269294713495,
-0.00438918614424969));
#53587=CARTESIAN_POINT('Ctrl Pts',(-0.00865158834960436,0.00101409730914674,
-0.00438662535591686));
#53588=CARTESIAN_POINT('Ctrl Pts',(-0.00862973231641669,0.00102389408403334,
-0.00438921693392455));
#53589=CARTESIAN_POINT('Ctrl Pts',(-0.00858288340936395,0.00105172009043307,
-0.00440193254517403));
#53590=CARTESIAN_POINT('Ctrl Pts',(-0.00855789795273511,0.00107226428316071,
-0.00441469677569042));
#53591=CARTESIAN_POINT('Ctrl Pts',(-0.00850849314601994,0.00112697168989658,
-0.00445471537180711));
#53592=CARTESIAN_POINT('Ctrl Pts',(-0.00848731866338639,0.00116211739589943,
-0.00448414297043919));
#53593=CARTESIAN_POINT('Ctrl Pts',(-0.00847459052587701,0.00119866682631849,
-0.00451811498504207));
#53594=CARTESIAN_POINT('Ctrl Pts',(-0.00847436147598704,0.00119933341534008,
-0.00451873568775905));
#53595=CARTESIAN_POINT('Ctrl Pts',(-0.00847413551305999,0.0012,-0.00451935750764786));
#53596=CARTESIAN_POINT('Origin',(0.00396253460616978,0.0128,0.));
#53597=CARTESIAN_POINT('Origin',(-0.000359710594690623,0.0128,-0.0122947390492059));
#53598=CARTESIAN_POINT('Origin',(-0.00828616193994173,0.0128,-0.00445104985208033));
#53599=CARTESIAN_POINT('Origin',(-0.00866210908617835,0.0172426406871193,
-0.00458766516321543));
#53600=CARTESIAN_POINT('Origin',(-0.00866210908617835,0.0128,-0.00458766516321543));
#53601=CARTESIAN_POINT('Origin',(-0.00866210908617835,0.0128,-0.00458766516321543));
#53602=CARTESIAN_POINT('Origin',(-0.00880510120094866,0.0128,-0.00421409688951767));
#53603=CARTESIAN_POINT('Origin',(-0.00926982557395217,0.0128,-0.003));
#53604=CARTESIAN_POINT('Ctrl Pts',(-0.00918425288415917,0.0128,-0.00150244288430738));
#53605=CARTESIAN_POINT('Ctrl Pts',(-0.00918425288415917,0.0128170824847327,
-0.00150244288430738));
#53606=CARTESIAN_POINT('Ctrl Pts',(-0.00918178381291453,0.012833758703744,
-0.00150477127744238));
#53607=CARTESIAN_POINT('Ctrl Pts',(-0.00917185354020169,0.0128680675590347,
-0.00151419537016038));
#53608=CARTESIAN_POINT('Ctrl Pts',(-0.00916385928771597,0.0128847555751617,
-0.00152180700263329));
#53609=CARTESIAN_POINT('Ctrl Pts',(-0.00914084612141564,0.0129201248655613,
-0.00154396884133387));
#53610=CARTESIAN_POINT('Ctrl Pts',(-0.00912437900625805,0.0129369061311702,
-0.00156000826915972));
#53611=CARTESIAN_POINT('Ctrl Pts',(-0.00908494519633725,0.0129671782156686,
-0.00159920014865634));
#53612=CARTESIAN_POINT('Ctrl Pts',(-0.00906084370069278,0.0129790454674433,
-0.00162368238643171));
#53613=CARTESIAN_POINT('Ctrl Pts',(-0.00900991177359934,0.0129957386317182,
-0.00167693589417492));
#53614=CARTESIAN_POINT('Ctrl Pts',(-0.0089823266678177,0.0129997703556913,
-0.00170667450021843));
#53615=CARTESIAN_POINT('Ctrl Pts',(-0.00895480987854902,0.012999996823628,
-0.00173740215050066));
#53616=CARTESIAN_POINT('Ctrl Pts',(-0.00895403629968172,0.013,-0.00173826686170102));
#53617=CARTESIAN_POINT('Ctrl Pts',(-0.00895326315945257,0.013,-0.00173913195070767));
#53618=CARTESIAN_POINT('Origin',(0.00396253460616978,0.0128,0.));
#53619=CARTESIAN_POINT('Ctrl Pts',(-0.00918425288415917,0.0128,0.00150244288430739));
#53620=CARTESIAN_POINT('Ctrl Pts',(-0.00918425288415917,0.0128170859338975,
0.00150244288430739));
#53621=CARTESIAN_POINT('Ctrl Pts',(-0.00918178281693229,0.0128337653687318,
0.0015047722151673));
#53622=CARTESIAN_POINT('Ctrl Pts',(-0.00917184364876475,0.0128680979862759,
0.00151420476610174));
#53623=CARTESIAN_POINT('Ctrl Pts',(-0.00916383629565585,0.0128848026420203,
0.00152182891425387));
#53624=CARTESIAN_POINT('Ctrl Pts',(-0.00914076136990567,0.0129202386542352,
0.00154405078036908));
#53625=CARTESIAN_POINT('Ctrl Pts',(-0.00912423199790756,0.0129370521043853,
0.00156015189581716));
#53626=CARTESIAN_POINT('Ctrl Pts',(-0.00908485146689577,0.0129672080432688,
0.00159929645791205));
#53627=CARTESIAN_POINT('Ctrl Pts',(-0.00906089667755369,0.0129790067173995,
0.00162363067642026));
#53628=CARTESIAN_POINT('Ctrl Pts',(-0.00901006148627273,0.0129957136180202,
0.00167677521626035));
#53629=CARTESIAN_POINT('Ctrl Pts',(-0.00898242682592675,0.0129997643999604,
0.0017065640468175));
#53630=CARTESIAN_POINT('Ctrl Pts',(-0.00895484578996856,0.0129999966744636,
0.00173736200896392));
#53631=CARTESIAN_POINT('Ctrl Pts',(-0.00895405424500949,0.013,0.00173824678215373));
#53632=CARTESIAN_POINT('Ctrl Pts',(-0.00895326315945257,0.013,0.00173913195070767));
#53633=CARTESIAN_POINT('Origin',(-0.00926982557395217,0.0128,0.003));
#53634=CARTESIAN_POINT('Origin',(-0.00880510120094866,0.0128,0.00421409688951767));
#53635=CARTESIAN_POINT('Origin',(-0.00866210908617835,0.0128,0.00458766516321543));
#53636=CARTESIAN_POINT('Origin',(-0.00828616193994173,0.0128,0.00445104985208033));
#53637=CARTESIAN_POINT('Origin',(-0.00866210908617835,0.0128,0.00458766516321543));
#53638=CARTESIAN_POINT('Origin',(0.00396253460616978,0.0128,0.));
#53639=CARTESIAN_POINT('Origin',(-0.000358432971552437,0.0127995376138349,
0.0122885638920572));
#53640=CARTESIAN_POINT('Origin',(-0.00866210908617835,0.0172426406871193,
0.00458766516321543));
#53641=CARTESIAN_POINT('Ctrl Pts',(-0.00872901544041542,0.001,0.00439918826870923));
#53642=CARTESIAN_POINT('Ctrl Pts',(-0.00871115018620075,0.000999999999999995,
0.00439284638245227));
#53643=CARTESIAN_POINT('Ctrl Pts',(-0.00869279015334176,0.0010026929471349,
0.00438918614424975));
#53644=CARTESIAN_POINT('Ctrl Pts',(-0.00865158834960484,0.00101409730914656,
0.00438662535591684));
#53645=CARTESIAN_POINT('Ctrl Pts',(-0.0086297323164172,0.0010238940840331,
0.00438921693392447));
#53646=CARTESIAN_POINT('Ctrl Pts',(-0.0085828834093646,0.00105172009043261,
0.00440193254517378));
#53647=CARTESIAN_POINT('Ctrl Pts',(-0.00855789795273577,0.0010722642831601,
0.00441469677569001));
#53648=CARTESIAN_POINT('Ctrl Pts',(-0.00850849314601959,0.00112697168989682,
0.00445471537180723));
#53649=CARTESIAN_POINT('Ctrl Pts',(-0.00848731866338683,0.00116211739590194,
0.00448414297043797));
#53650=CARTESIAN_POINT('Ctrl Pts',(-0.008474590525877,0.00119866682631824,
0.00451811498504211));
#53651=CARTESIAN_POINT('Ctrl Pts',(-0.00847436147598702,0.00119933341534014,
0.00451873568775911));
#53652=CARTESIAN_POINT('Ctrl Pts',(-0.00847413551305999,0.0012,0.00451935750764786));
#53653=CARTESIAN_POINT('Origin',(-0.000359710594690623,-0.0267643850402721,
0.0122947390492058));
#53654=CARTESIAN_POINT('Origin',(-0.000359710594690623,0.0012,0.0122947390492058));
#53655=CARTESIAN_POINT('Origin',(0.00396253460616978,0.0012,0.));
#53656=CARTESIAN_POINT('Origin',(-0.000492372526715893,0.0012,0.0126720993701079));
#53657=CARTESIAN_POINT('Origin',(-0.000359710594690623,0.0012,0.0122947390492058));
#53658=CARTESIAN_POINT('Origin',(-0.000371408500209017,0.0012,0.0126945679613751));
#53659=CARTESIAN_POINT('Origin',(0.,0.0012,0.));
#53660=CARTESIAN_POINT('Origin',(0.00625,0.0012,0.0110556546617557));
#53661=CARTESIAN_POINT('Ctrl Pts',(-0.0217851806760967,0.0133379298455257,
0.00635852171619724));
#53662=CARTESIAN_POINT('Ctrl Pts',(-0.0217547869618247,0.0134,0.00630782040048327));
#53663=CARTESIAN_POINT('Ctrl Pts',(-0.0217107156962388,0.0134,0.00623430285898128));
#53664=CARTESIAN_POINT('Ctrl Pts',(-0.0211059273377224,0.0133284526427957,
0.00677623426358248));
#53665=CARTESIAN_POINT('Ctrl Pts',(-0.0210679711108307,0.0133999999999989,
0.00672870310400759));
#53666=CARTESIAN_POINT('Ctrl Pts',(-0.0210335277181246,0.0134,0.00664025400640994));
#53667=CARTESIAN_POINT('Ctrl Pts',(-0.0204008307143018,0.0133220811407593,
0.00713526585043071));
#53668=CARTESIAN_POINT('Ctrl Pts',(-0.0203697574984378,0.0134000000000006,
0.00708353647612649));
#53669=CARTESIAN_POINT('Ctrl Pts',(-0.0203298528305533,0.0134,0.00699354067580272));
#53670=CARTESIAN_POINT('Ctrl Pts',(-0.0196903594652534,0.0133183218342735,
0.0074805711203105));
#53671=CARTESIAN_POINT('Ctrl Pts',(-0.0196643483248125,0.0134,0.00742657395762507));
#53672=CARTESIAN_POINT('Ctrl Pts',(-0.0196203815614496,0.0134,0.00733530227811308));
#53673=CARTESIAN_POINT('Ctrl Pts',(-0.0196330752852868,0.0134,0.00732918600636585));
#53674=CARTESIAN_POINT('Ctrl Pts',(-0.0196818597813691,0.0134,0.00736910397047182));
#53675=CARTESIAN_POINT('Ctrl Pts',(-0.0197202603260748,0.0133753834465396,
0.00740233387196754));
#53676=CARTESIAN_POINT('Ctrl Pts',(-0.0197452145249671,0.0133494224881884,
0.00742268581627776));
#53677=CARTESIAN_POINT('Ctrl Pts',(-0.0197546009360699,0.0133396573889856,
0.00743034110975611));
#53678=CARTESIAN_POINT('Ctrl Pts',(-0.0197622739680707,0.0133295676857738,
0.00743656499904525));
#53679=CARTESIAN_POINT('Ctrl Pts',(-0.0197684494911197,0.013319646237248,
0.00744180675098383));
#53680=CARTESIAN_POINT('Origin',(-0.0217118521071243,0.0132000091012597,
0.00623362616163613));
#53681=CARTESIAN_POINT('Origin',(0.,0.0148,0.));
#53682=CARTESIAN_POINT('Origin',(-0.00829461958536103,0.0148,0.0140317242680344));
#53683=CARTESIAN_POINT('Origin',(-5.55111512312578E-20,0.0148,0.0163));
#53684=CARTESIAN_POINT('Origin',(0.000968491838391537,0.0132,0.0195074579675537));
#53685=CARTESIAN_POINT('',(-0.0196508596780355,0.0133196394337182,0.00750485043938584));
#53686=CARTESIAN_POINT('Ctrl Pts',(-0.0196330752852202,0.0133999065795009,
0.00732918623248855));
#53687=CARTESIAN_POINT('Ctrl Pts',(-0.01964049658091,0.0134002169462812,
0.00740499113020126));
#53688=CARTESIAN_POINT('Ctrl Pts',(-0.019646536705005,0.0133653010300346,
0.00746003419317941));
#53689=CARTESIAN_POINT('Ctrl Pts',(-0.0196493113876324,0.0133341571395498,
0.00749087942416069));
#53690=CARTESIAN_POINT('Ctrl Pts',(-0.0196497622599861,0.013329096409697,
0.00749589162330514));
#53691=CARTESIAN_POINT('Ctrl Pts',(-0.0196501721052253,0.0133240756827054,
0.007500349096231));
#53692=CARTESIAN_POINT('Ctrl Pts',(-0.0196505706684233,0.01331918635986,
0.00750430757167277));
#53693=CARTESIAN_POINT('Ctrl Pts',(-0.0196508596780355,0.0133196394337182,
0.00750485043938584));
#53694=CARTESIAN_POINT('Ctrl Pts',(-0.0196517301463747,0.0133094372306776,
0.00751318281902652));
#53695=CARTESIAN_POINT('Ctrl Pts',(-0.0196359506058628,0.0133103209938461,
0.00752127600829986));
#53696=CARTESIAN_POINT('Ctrl Pts',(-0.0196236297821887,0.0133096914985585,
0.00752903889497462));
#53697=CARTESIAN_POINT('Ctrl Pts',(-0.0196113089585145,0.0133090620032709,
0.00753680178164939));
#53698=CARTESIAN_POINT('Ctrl Pts',(-0.0196022669562798,0.0133066853648818,
0.00754393004283313));
#53699=CARTESIAN_POINT('Ctrl Pts',(-0.0195925258808658,0.0133048042394914,
0.00755103279544104));
#53700=CARTESIAN_POINT('Ctrl Pts',(-0.0195730437300377,0.0133010419887106,
0.00756523830065686));
#53701=CARTESIAN_POINT('Ctrl Pts',(-0.0195508365550145,0.0132993344156868,
0.00757946233409064));
#53702=CARTESIAN_POINT('Ctrl Pts',(-0.0195289992545459,0.013297538858661,
0.00759353629382882));
#53703=CARTESIAN_POINT('Ctrl Pts',(-0.0194853246536087,0.0132939477446093,
0.0076216842133052));
#53704=CARTESIAN_POINT('Ctrl Pts',(-0.0194430435141633,0.0132899297432538,
0.00764908629261058));
#53705=CARTESIAN_POINT('Ctrl Pts',(-0.0194001542186181,0.013286475558855,
0.00767636368086573));
#53706=CARTESIAN_POINT('Ctrl Pts',(-0.0193572649230729,0.0132830213744561,
0.00770364106912088));
#53707=CARTESIAN_POINT('Ctrl Pts',(-0.0193137841852262,0.013280139625784,
0.00773082204048671));
#53708=CARTESIAN_POINT('Ctrl Pts',(-0.019270341051663,0.0132773369080536,
0.00775786787866913));
#53709=CARTESIAN_POINT('Ctrl Pts',(-0.0192268979180997,0.0132745341903232,
0.00778491371685154));
#53710=CARTESIAN_POINT('Ctrl Pts',(-0.0191834870690465,0.013271808031535,
0.00781181542257173));
#53711=CARTESIAN_POINT('Ctrl Pts',(-0.0191399980595519,0.013269199341757,
0.00783864075413296));
#53712=CARTESIAN_POINT('Ctrl Pts',(-0.0190530200405629,0.013263981962201,
0.00789229141725542));
#53713=CARTESIAN_POINT('Ctrl Pts',(-0.0189657348924197,0.0132592362260527,
0.0079456459092374));
#53714=CARTESIAN_POINT('Ctrl Pts',(-0.0188783451923207,0.0132547235819708,
0.0079987961202624));
#53715=CARTESIAN_POINT('Ctrl Pts',(-0.0187909554922218,0.013250210937889,
0.0080519463312874));
#53716=CARTESIAN_POINT('Ctrl Pts',(-0.018703457929881,0.0132459303061245,
0.00810488666145772));
#53717=CARTESIAN_POINT('Ctrl Pts',(-0.0186158618349587,0.0132418368276672,
0.0081576848485452));
#53718=CARTESIAN_POINT('Ctrl Pts',(-0.018440669645114,0.0132336498707526,
0.00826328122272014));
#53719=CARTESIAN_POINT('Ctrl Pts',(-0.0182650877987147,0.013226212373642,
0.0083683165926902));
#53720=CARTESIAN_POINT('Ctrl Pts',(-0.0180892882551675,0.0132192925299878,
0.00847301660256035));
#53721=CARTESIAN_POINT('Ctrl Pts',(-0.0179134887116204,0.0132123726863335,
0.00857771661243049));
#53722=CARTESIAN_POINT('Ctrl Pts',(-0.0177374668317145,0.0132059702596472,
0.00868207341420632));
#53723=CARTESIAN_POINT('Ctrl Pts',(-0.0175612941370432,0.0131999999999863,
0.00878621496200948));
#53724=CARTESIAN_POINT('Origin',(-0.0170139362062251,0.0132,0.00887744578929155));
#53725=CARTESIAN_POINT('Origin',(-0.0315929984201515,0.0132338047728166,
0.000421641309267139));
#53726=CARTESIAN_POINT('Origin',(-0.0306447771669106,0.0131997021086423,
0.00097908882428757));
#53727=CARTESIAN_POINT('Origin',(0.0125,0.0148,0.0163));
#53728=CARTESIAN_POINT('Origin',(0.0125000000000002,0.0148,0.0163));
#53729=CARTESIAN_POINT('Origin',(0.000968491838391537,0.0148,0.0195074579675537));
#53730=CARTESIAN_POINT('Origin',(-0.0166089107357433,0.0148,0.00911686983553521));
#53731=CARTESIAN_POINT('Origin',(-0.0166089107357433,-0.0233872477181734,
0.00911686983553521));
#53732=CARTESIAN_POINT('Origin',(-0.0166089107357433,0.0136,0.00911686983553521));
#53733=CARTESIAN_POINT('Origin',(-0.0166089107357433,0.0148,0.00911686983553521));
#53734=CARTESIAN_POINT('Ctrl Pts',(-0.016701694953409,0.0136,0.00893969452982875));
#53735=CARTESIAN_POINT('Ctrl Pts',(-0.0170198255739522,0.0136,0.00910629506495907));
#53736=CARTESIAN_POINT('Ctrl Pts',(-0.0167106852091834,0.0136,0.00928903823146202));
#53737=CARTESIAN_POINT('Ctrl Pts',(-0.0167016949536332,0.0135476400133573,
0.00893969452994618));
#53738=CARTESIAN_POINT('Ctrl Pts',(-0.0170198255700888,0.013605866918945,
0.00910629506724286));
#53739=CARTESIAN_POINT('Ctrl Pts',(-0.0167106852095972,0.0134952800267145,
0.00928903823121737));
#53740=CARTESIAN_POINT('Ctrl Pts',(-0.0167693533640173,0.0134433372808467,
0.00892620607872109));
#53741=CARTESIAN_POINT('Ctrl Pts',(-0.0169535261534895,0.0135821048236451,
0.00914548686070417));
#53742=CARTESIAN_POINT('Ctrl Pts',(-0.0167984486911777,0.0132866745615678,
0.00923715831401753));
#53743=CARTESIAN_POINT('Ctrl Pts',(-0.0169321915143027,0.0134,0.00889374249599453));
#53744=CARTESIAN_POINT('Ctrl Pts',(-0.0170429823123482,0.0134296096361944,
0.0090926063455859));
#53745=CARTESIAN_POINT('Ctrl Pts',(-0.0170096750997843,0.0132000000002514,
0.00911229534833304));
#53746=CARTESIAN_POINT('Ctrl Pts',(-0.0170139362062252,0.0134,0.00887744578929154));
#53747=CARTESIAN_POINT('Ctrl Pts',(-0.0171157106796652,0.0134,0.00904961418521835));
#53748=CARTESIAN_POINT('Ctrl Pts',(-0.0171157106796652,0.0132,0.00904961418521835));
#53749=CARTESIAN_POINT('Origin',(-0.0170139362062251,0.0136,0.00887744578929155));
#53750=CARTESIAN_POINT('Origin',(-0.0300600678275123,0.0132000279471769,
2.05249395217151E-8));
#53751=CARTESIAN_POINT('Origin',(-0.0306415836854525,0.0132275415761495,
-0.000977259614057599));
#53752=CARTESIAN_POINT('Origin',(0.0125,0.0148,-4.59242549680257E-18));
#53753=CARTESIAN_POINT('Origin',(0.0125,0.0148,-0.0163));
#53754=CARTESIAN_POINT('Origin',(-0.0166089107357433,0.0148,0.00911686983553521));
#53755=CARTESIAN_POINT('Origin',(-0.0166089107357433,0.0148,0.00911686983553521));
#53756=CARTESIAN_POINT('Origin',(-0.0171126097916178,0.0136,0.0089291197592526));
#53757=CARTESIAN_POINT('Origin',(-0.00395280707079757,0.0136,0.00203751601562436));
#53758=CARTESIAN_POINT('Origin',(-0.031417620514871,0.0132317057944348,
-0.000523328499505522));
#53759=CARTESIAN_POINT('Origin',(-0.0218622149050354,0.0132000088155134,
-0.00614623259346473));
#53760=CARTESIAN_POINT('Origin',(-5.75539309396805E-17,0.0148,-0.0163));
#53761=CARTESIAN_POINT('Origin',(-5.5913058681838E-17,0.0148,-0.0163));
#53762=CARTESIAN_POINT('Origin',(-0.0169270413562866,0.0148,0.00928347037066553));
#53763=CARTESIAN_POINT('Origin',(-0.00376723863546634,0.0148,0.00239186662703728));
#53764=CARTESIAN_POINT('Origin',(-0.00501982557395217,0.0136,-2.16840434497101E-19));
#53765=CARTESIAN_POINT('Origin',(-0.00395280707079757,0.0136,-0.00203751601562436));
#53766=CARTESIAN_POINT('Ctrl Pts',(-0.0218610959359586,0.0134,-0.00614689907887383));
#53767=CARTESIAN_POINT('Ctrl Pts',(-0.0219044727354385,0.0134,-0.00621925440718493));
#53768=CARTESIAN_POINT('Ctrl Pts',(-0.0219347456955486,0.0133395813452038,
-0.00626975167747655));
#53769=CARTESIAN_POINT('Ctrl Pts',(-0.0211908357465453,0.0134,-0.00654871801303158));
#53770=CARTESIAN_POINT('Ctrl Pts',(-0.0212247955992385,0.0134,-0.00663581415013928));
#53771=CARTESIAN_POINT('Ctrl Pts',(-0.0212623782205978,0.0133302265401987,
-0.0066834625777092));
#53772=CARTESIAN_POINT('Ctrl Pts',(-0.0204946261712406,0.0134,-0.00689690575881084));
#53773=CARTESIAN_POINT('Ctrl Pts',(-0.020533789466998,0.0134000000000018,
-0.00698567815694382));
#53774=CARTESIAN_POINT('Ctrl Pts',(-0.0205647582082835,0.0133238888195004,
-0.00703748207612315));
#53775=CARTESIAN_POINT('Ctrl Pts',(-0.0197927551089427,0.0134,-0.00723339256190528));
#53776=CARTESIAN_POINT('Ctrl Pts',(-0.0198359543513604,0.0134,-0.00732350099258878));
#53777=CARTESIAN_POINT('Ctrl Pts',(-0.019861893665148,0.0133200915216836,
-0.00737760728537532));
#53778=CARTESIAN_POINT('Ctrl Pts',(-0.0199408118980957,0.0133213184223535,
-0.00733868056421511));
#53779=CARTESIAN_POINT('Ctrl Pts',(-0.019922092925456,0.0133504885578351,
-0.00732298807146352));
#53780=CARTESIAN_POINT('Ctrl Pts',(-0.0198891712274851,0.0133836292280226,
-0.00729672973567592));
#53781=CARTESIAN_POINT('Ctrl Pts',(-0.0198402998718966,0.01339574276528,
-0.00725610951526527));
#53782=CARTESIAN_POINT('Ctrl Pts',(-0.0198293072782953,0.0133984674531988,
-0.00724697284267681));
#53783=CARTESIAN_POINT('Ctrl Pts',(-0.019817587588659,0.0134,-0.00723727462473279));
#53784=CARTESIAN_POINT('Ctrl Pts',(-0.0198053128358601,0.0134,-0.00722737066271768));
#53785=CARTESIAN_POINT('Origin',(0.,0.0148,0.));
#53786=CARTESIAN_POINT('Origin',(-0.00829461958536102,0.0148,-0.0140317242680344));
#53787=CARTESIAN_POINT('Origin',(-0.00501982557395217,0.0148,-2.16840434497101E-19));
#53788=CARTESIAN_POINT('Origin',(-0.00376723863546634,0.0148,-0.00239186662703728));
#53789=CARTESIAN_POINT('Origin',(-0.0171126097916178,0.0136,-0.0089291197592526));
#53790=CARTESIAN_POINT('Origin',(-0.0170139362062251,0.0136,-0.00887744578929154));
#53791=CARTESIAN_POINT('Origin',(0.00096849183839154,0.0132,-0.0195074579675537));
#53792=CARTESIAN_POINT('',(-0.0198215803223295,0.013321303084244,-0.00740247338649423));
#53793=CARTESIAN_POINT('Ctrl Pts',(-0.0177200739051678,0.0132,-0.00869235495241354));
#53794=CARTESIAN_POINT('Ctrl Pts',(-0.0178972982560502,0.0132061003755682,
-0.00858759173559485));
#53795=CARTESIAN_POINT('Ctrl Pts',(-0.0180743645746548,0.0132126395146285,
-0.00848260398841626));
#53796=CARTESIAN_POINT('Ctrl Pts',(-0.0182511976186223,0.0132197008401163,
-0.00837726012578567));
#53797=CARTESIAN_POINT('Ctrl Pts',(-0.0184280306625898,0.0132267621656041,
-0.00827191626315508));
#53798=CARTESIAN_POINT('Ctrl Pts',(-0.0186046351512701,0.0132343459282969,
-0.00816622426863558));
#53799=CARTESIAN_POINT('Ctrl Pts',(-0.018780836856243,0.0132426797505751,
-0.00805995094578348));
#53800=CARTESIAN_POINT('Ctrl Pts',(-0.0188689377087295,0.0132468466617142,
-0.00800681428435743));
#53801=CARTESIAN_POINT('Ctrl Pts',(-0.0189569367254928,0.0132512008628788,
-0.0079535303626938));
#53802=CARTESIAN_POINT('Ctrl Pts',(-0.0190448205904563,0.0132557864815963,
-0.00790003202857749));
#53803=CARTESIAN_POINT('Ctrl Pts',(-0.0191327044554197,0.0132603721003139,
-0.00784653369446118));
#53804=CARTESIAN_POINT('Ctrl Pts',(-0.0192204765343328,0.0132651902745664,
-0.00779282664161546));
#53805=CARTESIAN_POINT('Ctrl Pts',(-0.0193079453907042,0.0132704778764169,
-0.0077388080222866));
#53806=CARTESIAN_POINT('Ctrl Pts',(-0.0193516798188899,0.0132731216773421,
-0.00771179871262217));
#53807=CARTESIAN_POINT('Ctrl Pts',(-0.019395337056506,0.0132758823759434,
-0.00768470916849096));
#53808=CARTESIAN_POINT('Ctrl Pts',(-0.0194390290153232,0.013278720806396,
-0.00765746961801436));
#53809=CARTESIAN_POINT('Ctrl Pts',(-0.0194827209741404,0.0132815592368486,
-0.00763023006753776));
#53810=CARTESIAN_POINT('Ctrl Pts',(-0.0195264529796914,0.013284477938968,
-0.00760284951973719));
#53811=CARTESIAN_POINT('Ctrl Pts',(-0.0195695851804412,0.013287962453304,
-0.00757537035271812));
#53812=CARTESIAN_POINT('Ctrl Pts',(-0.0196127173811911,0.0132914469676401,
-0.00754789118569905));
#53813=CARTESIAN_POINT('Ctrl Pts',(-0.0196552331874147,0.0132954885780045,
-0.00752028533519109));
#53814=CARTESIAN_POINT('Ctrl Pts',(-0.0196991269521685,0.0132991224730883,
-0.00749192947659815));
#53815=CARTESIAN_POINT('Ctrl Pts',(-0.0197210738345454,0.0133009394206302,
-0.00747775154730168));
#53816=CARTESIAN_POINT('Ctrl Pts',(-0.0197433866480824,0.0133026735298679,
-0.00746342238788288));
#53817=CARTESIAN_POINT('Ctrl Pts',(-0.0197629783330933,0.0133064335087228,
-0.00744909564974968));
#53818=CARTESIAN_POINT('Ctrl Pts',(-0.0197727741755988,0.0133083134981502,
-0.00744193228068309));
#53819=CARTESIAN_POINT('Ctrl Pts',(-0.0197818720451141,0.0133106815439565,
-0.00743473958991742));
#53820=CARTESIAN_POINT('Ctrl Pts',(-0.0197942328454585,0.0133113429113141,
-0.00742691782953974));
#53821=CARTESIAN_POINT('Ctrl Pts',(-0.0198065936458028,0.0133120042786716,
-0.00741909606916207));
#53822=CARTESIAN_POINT('Ctrl Pts',(-0.0198223960209913,0.0133111962794624,
-0.00741094744514287));
#53823=CARTESIAN_POINT('Ctrl Pts',(-0.0198215803223295,0.013321303084244,
-0.00740247338649423));
#53824=CARTESIAN_POINT('Ctrl Pts',(-0.0198213244982509,0.0133208884971597,
-0.00740199237898985));
#53825=CARTESIAN_POINT('Ctrl Pts',(-0.0198186243540202,0.0133553313782365,
-0.00737322845529448));
#53826=CARTESIAN_POINT('Ctrl Pts',(-0.0198153027363176,0.0133810561537279,
-0.0073370106567662));
#53827=CARTESIAN_POINT('Ctrl Pts',(-0.0198101938602386,0.0133939472752386,
-0.0072809710310928));
#53828=CARTESIAN_POINT('Ctrl Pts',(-0.0198087235859192,0.0133976571880671,
-0.00726484348733972));
#53829=CARTESIAN_POINT('Ctrl Pts',(-0.0198070715857852,0.0134000059680804,
-0.00724701116723406));
#53830=CARTESIAN_POINT('Ctrl Pts',(-0.0198053126720851,0.0133999709244785,
-0.00722737055260438));
#53831=CARTESIAN_POINT('Origin',(-0.0170139362062251,0.0132,-0.00887744578929154));
#53832=CARTESIAN_POINT('Origin',(0.00096849183839154,0.0148,-0.0195074579675537));
#53833=CARTESIAN_POINT('Origin',(-0.0166089107357434,0.0148,-0.00911686983553521));
#53834=CARTESIAN_POINT('Origin',(-0.0169270413562866,0.0148,-0.00928347037066553));
#53835=CARTESIAN_POINT('Origin',(-0.0166089107357433,0.0148,-0.0091168698355352));
#53836=CARTESIAN_POINT('Ctrl Pts',(-0.0170139362062251,0.0134,-0.00887744578929154));
#53837=CARTESIAN_POINT('Ctrl Pts',(-0.0171157106796652,0.0134,-0.00904961418521834));
#53838=CARTESIAN_POINT('Ctrl Pts',(-0.0171157106796652,0.0132,-0.00904961418521834));
#53839=CARTESIAN_POINT('Ctrl Pts',(-0.0169321915143036,0.0134,-0.00889374249599441));
#53840=CARTESIAN_POINT('Ctrl Pts',(-0.017042982312349,0.0134296096361945,
-0.00909260634558574));
#53841=CARTESIAN_POINT('Ctrl Pts',(-0.0170096750997843,0.0132000000002514,
-0.00911229534833303));
#53842=CARTESIAN_POINT('Ctrl Pts',(-0.0167693533640169,0.0134433372808467,
-0.00892620607872114));
#53843=CARTESIAN_POINT('Ctrl Pts',(-0.0169535261534889,0.0135821048236453,
-0.00914548686070429));
#53844=CARTESIAN_POINT('Ctrl Pts',(-0.0167984486911777,0.0132866745615676,
-0.00923715831401752));
#53845=CARTESIAN_POINT('Ctrl Pts',(-0.0167016949536332,0.0135476400133573,
-0.00893969452994617));
#53846=CARTESIAN_POINT('Ctrl Pts',(-0.0170198255700888,0.0136058669189446,
-0.00910629506724285));
#53847=CARTESIAN_POINT('Ctrl Pts',(-0.0167106852095972,0.0134952800267149,
-0.00928903823121736));
#53848=CARTESIAN_POINT('Ctrl Pts',(-0.016701694953409,0.0136,-0.00893969452982874));
#53849=CARTESIAN_POINT('Ctrl Pts',(-0.0170198255739522,0.0136,-0.00910629506495906));
#53850=CARTESIAN_POINT('Ctrl Pts',(-0.0167106852091834,0.0136,-0.00928903823146201));
#53851=CARTESIAN_POINT('Origin',(-0.0166089107357433,0.0136,-0.0091168698355352));
#53852=CARTESIAN_POINT('Origin',(-0.0166089107357433,0.0148,-0.00911686983553521));
#53853=CARTESIAN_POINT('Origin',(-0.0166089107357433,0.0148,-0.00911686983553521));
#53854=CARTESIAN_POINT('Origin',(-0.0166089107357433,0.015,-0.00911686983553521));
#53855=CARTESIAN_POINT('Origin',(0.0125,0.0132,-4.59242549680257E-18));
#53856=CARTESIAN_POINT('Origin',(0.0125,0.0132,-4.59242549680257E-18));
#53857=CARTESIAN_POINT('Origin',(0.0125,0.0132,-0.0123));
#53858=CARTESIAN_POINT('Origin',(0.0125,0.0136,-4.59242549680257E-18));
#53859=CARTESIAN_POINT('Origin',(0.0125,0.0136,-0.0092));
#53860=CARTESIAN_POINT('Ctrl Pts',(-0.0206729454446971,0.,0.00682621009066018));
#53861=CARTESIAN_POINT('Ctrl Pts',(-0.0207261905924628,0.,0.00691508186067457));
#53862=CARTESIAN_POINT('Ctrl Pts',(-0.0207569064148775,8.46248955869717E-5,
0.00696634980939847));
#53863=CARTESIAN_POINT('Ctrl Pts',(-0.0199012495314622,0.,0.00728855107959443));
#53864=CARTESIAN_POINT('Ctrl Pts',(-0.0199411001596944,3.10281366133179E-17,
0.00739573685041475));
#53865=CARTESIAN_POINT('Ctrl Pts',(-0.0199830342135227,9.5792117705873E-5,
0.00743918849379106));
#53866=CARTESIAN_POINT('Ctrl Pts',(-0.0191043571886283,0.,0.00770407151128956));
#53867=CARTESIAN_POINT('Ctrl Pts',(-0.0191527383496395,-4.83326594045924E-17,
0.00781167719406153));
#53868=CARTESIAN_POINT('Ctrl Pts',(-0.0191854693058945,0.000103035383687346,
0.00785914556601559));
#53869=CARTESIAN_POINT('Ctrl Pts',(-0.0183042279408874,0.,0.0081135770554014));
#53870=CARTESIAN_POINT('Ctrl Pts',(-0.0183595141901171,1.35525271560688E-20,
0.00822160036715122));
#53871=CARTESIAN_POINT('Ctrl Pts',(-0.0183850475118973,0.000107632287825602,
0.00827148969799038));
#53872=CARTESIAN_POINT('Ctrl Pts',(-0.018451268973799,0.000107232892182658,
0.00823734560780459));
#53873=CARTESIAN_POINT('Ctrl Pts',(-0.01843973701703,7.76784087736853E-5,
0.0082258681813287));
#53874=CARTESIAN_POINT('Ctrl Pts',(-0.018417431856287,4.69122920424372E-5,
0.00820537292668292));
#53875=CARTESIAN_POINT('Ctrl Pts',(-0.0183963224542028,2.89310499208856E-5,
0.0081828289210615));
#53876=CARTESIAN_POINT('Ctrl Pts',(-0.0183752130521186,1.09498077993341E-5,
0.00816028491544008));
#53877=CARTESIAN_POINT('Ctrl Pts',(-0.0183568899610538,-3.23379581101954E-19,
0.00813879781574077));
#53878=CARTESIAN_POINT('Ctrl Pts',(-0.0183185440104958,0.,0.00810624927208572));
#53879=CARTESIAN_POINT('Origin',(-0.0206729454446971,0.0002,0.0068262100906602));
#53880=CARTESIAN_POINT('Origin',(-0.00829461958536102,0.0002,0.0140317242680344));
#53881=CARTESIAN_POINT('',(-0.0183580519175386,0.000107246172780706,0.00828872892562513));
#53882=CARTESIAN_POINT('Ctrl Pts',(-0.0167335787825944,0.0002,0.0092755050776766));
#53883=CARTESIAN_POINT('Ctrl Pts',(-0.016870203120021,0.00019553998556168,
0.00919474188112224));
#53884=CARTESIAN_POINT('Ctrl Pts',(-0.017006750934428,0.000190796366481944,
0.00911385415689994));
#53885=CARTESIAN_POINT('Ctrl Pts',(-0.0171431642092931,0.000185672027589209,
0.00903278828563277));
#53886=CARTESIAN_POINT('Ctrl Pts',(-0.0171601411622557,0.000185034291559247,
0.00902269944725));
#53887=CARTESIAN_POINT('Ctrl Pts',(-0.0171771158819337,0.000184390696478422,
0.00901260792396832));
#53888=CARTESIAN_POINT('Ctrl Pts',(-0.017194088540261,0.000183741048692459,
0.00900251343072304));
#53889=CARTESIAN_POINT('Ctrl Pts',(-0.0173134946485287,0.000179170644200067,
0.00893149661472916));
#53890=CARTESIAN_POINT('Ctrl Pts',(-0.0174328055967938,0.000174302961947506,
0.00886033035739381));
#53891=CARTESIAN_POINT('Ctrl Pts',(-0.0175519749817655,0.000168986864193267,
0.00878891407725371));
#53892=CARTESIAN_POINT('Ctrl Pts',(-0.0175826051732513,0.00016762046381948,
0.00877055790014992));
#53893=CARTESIAN_POINT('Ctrl Pts',(-0.0176132055874596,0.000166226880574114,
0.00875219768570016));
#53894=CARTESIAN_POINT('Ctrl Pts',(-0.0176438103849298,0.000164798089442301,
0.00873380982018834));
#53895=CARTESIAN_POINT('Ctrl Pts',(-0.0176812033644573,0.000163052390664412,
0.00871134350328783));
#53896=CARTESIAN_POINT('Ctrl Pts',(-0.0177186037909279,0.000161254130880076,
0.00868883543588592));
#53897=CARTESIAN_POINT('Ctrl Pts',(-0.0177559384513345,0.000159383309477981,
0.00866631559980144));
#53898=CARTESIAN_POINT('Ctrl Pts',(-0.017823830177126,0.000155981288614457,
0.00862536409469426));
#53899=CARTESIAN_POINT('Ctrl Pts',(-0.017891627135883,0.000152374921470389,
0.00858431261540693));
#53900=CARTESIAN_POINT('Ctrl Pts',(-0.017959730776856,0.000148368781047435,
0.00854280759069639));
#53901=CARTESIAN_POINT('Ctrl Pts',(-0.0179937825973424,0.000146365710835958,
0.00852205507834112));
#53902=CARTESIAN_POINT('Ctrl Pts',(-0.0180276481757308,0.000144276554852942,
0.00850134808399079));
#53903=CARTESIAN_POINT('Ctrl Pts',(-0.0180610836837602,0.000142090071389666,
0.00848081907584841));
#53904=CARTESIAN_POINT('Ctrl Pts',(-0.0180641279310168,0.000141890995716018,
0.00847894994388656));
#53905=CARTESIAN_POINT('Ctrl Pts',(-0.0180671802477625,0.000141690388311206,
0.00847707515616403));
#53906=CARTESIAN_POINT('Ctrl Pts',(-0.0180702400274756,0.000141488245959845,
0.00847519505648417));
#53907=CARTESIAN_POINT('Ctrl Pts',(-0.0181007863515196,0.000139470222982215,
0.00845642568762774));
#53908=CARTESIAN_POINT('Ctrl Pts',(-0.0181320898039847,0.000137301614487281,
0.00843712071736009));
#53909=CARTESIAN_POINT('Ctrl Pts',(-0.0181631255264992,0.0001348977973457,
0.00841781421912194));
#53910=CARTESIAN_POINT('Ctrl Pts',(-0.0181951710770037,0.000132415765758458,
0.00839787953372627));
#53911=CARTESIAN_POINT('Ctrl Pts',(-0.0182269603831239,0.000129687237058521,
0.0083779292554878));
#53912=CARTESIAN_POINT('Ctrl Pts',(-0.018257910967522,0.000126502915985151,
0.00835816520630279));
#53913=CARTESIAN_POINT('Ctrl Pts',(-0.0182764271408461,0.000124597897321993,
0.00834634137268504));
#53914=CARTESIAN_POINT('Ctrl Pts',(-0.0182955815663513,0.000122537179335476,
0.00833401545302579));
#53915=CARTESIAN_POINT('Ctrl Pts',(-0.0183155463531549,0.000121053263352702,
0.00832148692383736));
#53916=CARTESIAN_POINT('Ctrl Pts',(-0.0183280943035645,0.000120120616069915,
0.00831361269184541));
#53917=CARTESIAN_POINT('Ctrl Pts',(-0.0183424285341103,0.000119559534132814,
0.00830491130196657));
#53918=CARTESIAN_POINT('Ctrl Pts',(-0.018352680267871,0.000117343276337867,
0.00829769431201892));
#53919=CARTESIAN_POINT('Ctrl Pts',(-0.0183569540028375,0.000116419364475319,
0.0082946856987431));
#53920=CARTESIAN_POINT('Ctrl Pts',(-0.0183619411006891,0.00011063305116798,
0.00828848899624926));
#53921=CARTESIAN_POINT('Ctrl Pts',(-0.0183580519175386,0.000107246172780706,
0.00828872892562513));
#53922=CARTESIAN_POINT('Ctrl Pts',(-0.0183580389868516,0.000107244345009705,
0.00828873553226112));
#53923=CARTESIAN_POINT('Ctrl Pts',(-0.0183545804956432,7.77877261786513E-5,
0.00827286717337471));
#53924=CARTESIAN_POINT('Ctrl Pts',(-0.0183484379957968,4.67935037000903E-5,
0.00824319447998794));
#53925=CARTESIAN_POINT('Ctrl Pts',(-0.0183415805299276,2.89354452288591E-5,
0.0082130004877248));
#53926=CARTESIAN_POINT('Ctrl Pts',(-0.0183347229526445,1.10770966161947E-5,
0.00818280600489723));
#53927=CARTESIAN_POINT('Ctrl Pts',(-0.0183291093400749,4.59203235844747E-11,
0.00815540410168465));
#53928=CARTESIAN_POINT('Ctrl Pts',(-0.0183185438351041,2.1987620058006E-16,
0.00810624911031649));
#53929=CARTESIAN_POINT('Origin',(-0.00829461958536103,0.0002,0.0140317242680344));
#53930=CARTESIAN_POINT('Ctrl Pts',(-0.0309032482137635,5.85734536233529E-23,
0.000785457753406084));
#53931=CARTESIAN_POINT('Ctrl Pts',(-0.0309559999151988,-1.50815768680036E-17,
0.000872145039779753));
#53932=CARTESIAN_POINT('Ctrl Pts',(-0.0309844293408926,8.18824655704908E-5,
0.000924893432060964));
#53933=CARTESIAN_POINT('Ctrl Pts',(-0.029149510808606,-7.4625993722284E-22,
0.00180911851837678));
#53934=CARTESIAN_POINT('Ctrl Pts',(-0.0291437117667778,1.04850129722553E-16,
0.00194412775273983));
#53935=CARTESIAN_POINT('Ctrl Pts',(-0.0292400312363699,9.70131778003069E-5,
0.00195671427143983));
#53936=CARTESIAN_POINT('Ctrl Pts',(-0.025627466945566,1.50079397457481E-20,
0.00383185361080478));
#53937=CARTESIAN_POINT('Ctrl Pts',(-0.0256979250879764,-3.97855078320796E-16,
0.00398301591764444));
#53938=CARTESIAN_POINT('Ctrl Pts',(-0.0257319678794474,0.000164701302145256,
0.00400469466052874));
#53939=CARTESIAN_POINT('Ctrl Pts',(-0.0221555720892475,-2.92696195542735E-20,
0.00593921914836097));
#53940=CARTESIAN_POINT('Ctrl Pts',(-0.0222772613022354,5.99710111691989E-16,
0.00600319472741784));
#53941=CARTESIAN_POINT('Ctrl Pts',(-0.0222424088775952,0.000101917892232826,
0.00609197690023176));
#53942=CARTESIAN_POINT('Ctrl Pts',(-0.0204130553218997,-2.6933217319899E-20,
0.00698181563372554));
#53943=CARTESIAN_POINT('Ctrl Pts',(-0.0204657712517479,-9.3070861245427E-17,
0.00707344620791871));
#53944=CARTESIAN_POINT('Ctrl Pts',(-0.0204980517498235,8.73388957981665E-5,
0.00712348788289622));
#53945=CARTESIAN_POINT('Origin',(-0.030641586298985,0.000200000000000081,
0.00093807325632101));
#53946=CARTESIAN_POINT('Origin',(0.,0.0002,0.));
#53947=CARTESIAN_POINT('Origin',(0.,0.0002,0.0163));
#53948=CARTESIAN_POINT('Origin',(-0.0300842090696186,0.000199852455921088,
8.94993350727811E-8));
#53949=CARTESIAN_POINT('Origin',(-0.0306415078682799,0.000199999999999959,
-0.000938136151693087));
#53950=CARTESIAN_POINT('Origin',(1.72772815121504E-16,0.0002,0.0163));
#53951=CARTESIAN_POINT('Origin',(0.0125000000000002,0.0002,0.0163));
#53952=CARTESIAN_POINT('Ctrl Pts',(-0.0317225298040676,7.50059049772727E-5,
-0.000485888810412572));
#53953=CARTESIAN_POINT('Ctrl Pts',(-0.0317230373664694,9.08601866987305E-17,
-0.000416899367108417));
#53954=CARTESIAN_POINT('Ctrl Pts',(-0.0316451978945082,3.68628738645122E-21,
-0.000351300671161231));
#53955=CARTESIAN_POINT('Ctrl Pts',(-0.0297282606927244,8.49471121739984E-5,
-0.0016703560700287));
#53956=CARTESIAN_POINT('Ctrl Pts',(-0.0295579817604276,-1.51798941380492E-16,
-0.00169727441023402));
#53957=CARTESIAN_POINT('Ctrl Pts',(-0.0296397149165271,-1.19262238973414E-20,
-0.001528175376318));
#53958=CARTESIAN_POINT('Ctrl Pts',(-0.0257089904949931,0.00017109120157702,
-0.00401385795055467));
#53959=CARTESIAN_POINT('Ctrl Pts',(-0.0256722463681587,1.57875331656574E-16,
-0.0039952472777838));
#53960=CARTESIAN_POINT('Ctrl Pts',(-0.0256027281016292,6.6136332521626E-20,
-0.00383798124397724));
#53961=CARTESIAN_POINT('Ctrl Pts',(-0.0217137335921404,9.01571409957985E-5,
-0.00640668094362288));
#53962=CARTESIAN_POINT('Ctrl Pts',(-0.0218192026594173,-1.19741391585379E-16,
-0.0062719224035291));
#53963=CARTESIAN_POINT('Ctrl Pts',(-0.0216309143172447,-1.19262238973602E-20,
-0.00625785011357261));
#53964=CARTESIAN_POINT('Ctrl Pts',(-0.0197159421381394,8.02117903232503E-5,
-0.007583667403771));
#53965=CARTESIAN_POINT('Ctrl Pts',(-0.019655679728747,6.9889437387932E-17,
-0.00755045068836614));
#53966=CARTESIAN_POINT('Ctrl Pts',(-0.0196329910336286,3.68628738646249E-21,
-0.00744749148838045));
#53967=CARTESIAN_POINT('Origin',(-0.0206310823726759,0.0002,-0.00685120104972884));
#53968=CARTESIAN_POINT('Origin',(0.0125,0.0002,-4.59242549680257E-18));
#53969=CARTESIAN_POINT('Origin',(0.0125,0.0002,-0.0163));
#53970=CARTESIAN_POINT('Ctrl Pts',(-0.0207149455884366,8.43554830515145E-5,
-0.00699117714319487));
#53971=CARTESIAN_POINT('Ctrl Pts',(-0.0206842201344661,2.71050543121376E-20,
-0.00693989328795921));
#53972=CARTESIAN_POINT('Ctrl Pts',(-0.0206310823726745,0.,-0.00685120104972968));
#53973=CARTESIAN_POINT('Ctrl Pts',(-0.0199409189296865,9.54844683703659E-5,
-0.00746411055047154));
#53974=CARTESIAN_POINT('Ctrl Pts',(-0.0198990171876475,-1.98578856459192E-16,
-0.00742058444715366));
#53975=CARTESIAN_POINT('Ctrl Pts',(-0.0198592188402909,0.,-0.00731364399254252));
#53976=CARTESIAN_POINT('Ctrl Pts',(-0.0191437777603039,0.000102714870596185,
-0.00788384498404907));
#53977=CARTESIAN_POINT('Ctrl Pts',(-0.0191110107219842,-9.66541334231093E-17,
-0.00783631487172919));
#53978=CARTESIAN_POINT('Ctrl Pts',(-0.0190627669411057,0.,-0.00772891778103133));
#53979=CARTESIAN_POINT('Ctrl Pts',(-0.0183437447309265,0.000107326685769658,
-0.00829571182140303));
#53980=CARTESIAN_POINT('Ctrl Pts',(-0.018318191433809,-2.71050543121376E-20,
-0.00824574709711051));
#53981=CARTESIAN_POINT('Ctrl Pts',(-0.0182630443888809,0.,-0.00813791729797689));
#53982=CARTESIAN_POINT('Ctrl Pts',(-0.0182773531951025,0.,-0.00813059853245909));
#53983=CARTESIAN_POINT('Ctrl Pts',(-0.0183237401938969,-8.98673656062578E-19,
-0.00817597996129781));
#53984=CARTESIAN_POINT('Ctrl Pts',(-0.0183607091081757,2.90441480504016E-5,
-0.00821410741789105));
#53985=CARTESIAN_POINT('Ctrl Pts',(-0.0183837110698202,5.95874444262312E-5,
-0.00823616086343279));
#53986=CARTESIAN_POINT('Ctrl Pts',(-0.0183954716764099,7.52038382876884E-5,
-0.00824743650596148));
#53987=CARTESIAN_POINT('Ctrl Pts',(-0.0184040580625986,9.13930728185299E-5,
-0.00825544127361943));
#53988=CARTESIAN_POINT('Ctrl Pts',(-0.0184101483244441,0.000106933920730451,
-0.00826150146239095));
#53989=CARTESIAN_POINT('Origin',(0.0125,0.0002,-0.0163));
#53990=CARTESIAN_POINT('Origin',(-5.65435973303839E-17,0.0002,-0.0163));
#53991=CARTESIAN_POINT('Origin',(-0.00829461958536102,0.0002,-0.0140317242680344));
#53992=CARTESIAN_POINT('',(-0.0183165728615313,0.000106937857928121,-0.00831306077174831));
#53993=CARTESIAN_POINT('Ctrl Pts',(-0.0182773531237792,7.17402004746925E-8,
-0.00813059857217221));
#53994=CARTESIAN_POINT('Ctrl Pts',(-0.0182932596990271,-1.52680597115539E-7,
-0.00820516392882934));
#53995=CARTESIAN_POINT('Ctrl Pts',(-0.0183058695106016,3.83262775878502E-5,
-0.00826053175246635));
#53996=CARTESIAN_POINT('Ctrl Pts',(-0.0183119352413553,7.48753524682983E-5,
-0.00829084006900245));
#53997=CARTESIAN_POINT('Ctrl Pts',(-0.0183137536871268,8.58324017288368E-5,
-0.00829992620095999));
#53998=CARTESIAN_POINT('Ctrl Pts',(-0.01831515966709,9.67863519129567E-5,
-0.00830707883474611));
#53999=CARTESIAN_POINT('Ctrl Pts',(-0.0183163613629249,0.000107167142621255,
-0.00831267637528232));
#54000=CARTESIAN_POINT('Ctrl Pts',(-0.0183165728615313,0.000106937857928121,
-0.00831306077174831));
#54001=CARTESIAN_POINT('Ctrl Pts',(-0.0183176231313522,0.000115898484335213,
-0.00831791187551959));
#54002=CARTESIAN_POINT('Ctrl Pts',(-0.0183111189228912,0.000119376381868073,
-0.00832325866390957));
#54003=CARTESIAN_POINT('Ctrl Pts',(-0.0183019709395841,0.000120385225192318,
-0.00832917488410512));
#54004=CARTESIAN_POINT('Ctrl Pts',(-0.018292822956277,0.000121394068516563,
-0.00833509110430068));
#54005=CARTESIAN_POINT('Ctrl Pts',(-0.0182809403413241,0.000120021160600134,
-0.00834142305696103));
#54006=CARTESIAN_POINT('Ctrl Pts',(-0.0182706958539365,0.000119737357772785,
-0.00834733446742616));
#54007=CARTESIAN_POINT('Ctrl Pts',(-0.0182502068791613,0.000119169752118088,
-0.00835915728835641));
#54008=CARTESIAN_POINT('Ctrl Pts',(-0.018236279580929,0.000122970334818699,
-0.00836931344679148));
#54009=CARTESIAN_POINT('Ctrl Pts',(-0.0182210301194234,0.000125744392548628,
-0.00837961645538245));
#54010=CARTESIAN_POINT('Ctrl Pts',(-0.018190531196412,0.000131292508008485,
-0.0084002224725644));
#54011=CARTESIAN_POINT('Ctrl Pts',(-0.0181549294123503,0.000132620974976354,
-0.00842173018841584));
#54012=CARTESIAN_POINT('Ctrl Pts',(-0.0181205693182617,0.000134659993822246,
-0.00844286034392449));
#54013=CARTESIAN_POINT('Ctrl Pts',(-0.0180862092241731,0.000136699012668137,
-0.00846399049943315));
#54014=CARTESIAN_POINT('Ctrl Pts',(-0.0180530376061649,0.00013947305191,
-0.00848465307447684));
#54015=CARTESIAN_POINT('Ctrl Pts',(-0.0180194763349309,0.000141851554879295,
-0.00850533184841774));
#54016=CARTESIAN_POINT('Ctrl Pts',(-0.0179859150636969,0.00014423005784859,
-0.00852601062235864));
#54017=CARTESIAN_POINT('Ctrl Pts',(-0.0179519742820119,0.000146210446335367,
-0.00854672275338189));
#54018=CARTESIAN_POINT('Ctrl Pts',(-0.0179180631172835,0.000148146545055578,
-0.0085673725291748));
#54019=CARTESIAN_POINT('Ctrl Pts',(-0.0178502407878267,0.000152018742496001,
-0.00860867208076062));
#54020=CARTESIAN_POINT('Ctrl Pts',(-0.0177825274511162,0.00015571476862617,
-0.00864970618275563));
#54021=CARTESIAN_POINT('Ctrl Pts',(-0.0177146741348683,0.000159152003925665,
-0.00869064960328432));
#54022=CARTESIAN_POINT('Ctrl Pts',(-0.0176468208186205,0.000162589239225159,
-0.00873159302381301));
#54023=CARTESIAN_POINT('Ctrl Pts',(-0.0175788293634593,0.000165768310811214,
-0.00877244887659585));
#54024=CARTESIAN_POINT('Ctrl Pts',(-0.0175107954445577,0.000168810309252196,
-0.00881322390054543));
#54025=CARTESIAN_POINT('Ctrl Pts',(-0.0173747276067545,0.00017489430613416,
-0.00889477394844459));
#54026=CARTESIAN_POINT('Ctrl Pts',(-0.0172384887971941,0.000180428777406025,
-0.00897599879176508));
#54027=CARTESIAN_POINT('Ctrl Pts',(-0.0171021151044633,0.00018558234577026,
-0.00905704651762882));
#54028=CARTESIAN_POINT('Ctrl Pts',(-0.0169657414117325,0.000190735914134494,
-0.00913809424349255));
#54029=CARTESIAN_POINT('Ctrl Pts',(-0.0168292310524291,0.000195509330278561,
-0.00921896183497885));
#54030=CARTESIAN_POINT('Ctrl Pts',(-0.0166926437830518,0.0002,-0.00929970311937459));
#54031=CARTESIAN_POINT('Origin',(-0.00829461958536102,0.0002,-0.0140317242680344));
#54032=CARTESIAN_POINT('Origin',(0.,0.0002,0.));
#54033=CARTESIAN_POINT('Origin',(0.,0.0002,0.));
#54034=CARTESIAN_POINT('Ctrl Pts',(0.00624999999999999,0.0002,-0.0119660979437743));
#54035=CARTESIAN_POINT('Ctrl Pts',(0.00624999999999999,0.000198767450384323,
-0.0119660979437743));
#54036=CARTESIAN_POINT('Ctrl Pts',(0.00625000000000002,0.000197533969384649,
-0.011966110798073));
#54037=CARTESIAN_POINT('Ctrl Pts',(0.00625000000000002,0.000173042294632174,
-0.0119666221033105));
#54038=CARTESIAN_POINT('Ctrl Pts',(0.00624999999999949,0.000150239173956967,
-0.0119716741195774));
#54039=CARTESIAN_POINT('Ctrl Pts',(0.00624999999999945,0.000106108800044296,
-0.0119906202070117));
#54040=CARTESIAN_POINT('Ctrl Pts',(0.00624999999984408,8.55756873717683E-5,
-0.0120047838446837));
#54041=CARTESIAN_POINT('Ctrl Pts',(0.00624999999980556,4.81558075462784E-5,
-0.0120418505678853));
#54042=CARTESIAN_POINT('Ctrl Pts',(0.00625,3.23863339961406E-5,-0.0120652740542929));
#54043=CARTESIAN_POINT('Ctrl Pts',(0.00625,1.42587886819356E-5,-0.01210614745887));
#54044=CARTESIAN_POINT('Ctrl Pts',(0.00624999999996748,9.08500765451901E-6,
-0.0121221892847626));
#54045=CARTESIAN_POINT('Ctrl Pts',(0.00624999999993779,2.01730384467436E-6,
-0.0121551698535138));
#54046=CARTESIAN_POINT('Ctrl Pts',(0.00625000000000007,1.60816358981751E-7,
-0.0121720926860831));
#54047=CARTESIAN_POINT('Ctrl Pts',(0.00624999999999998,3.33362078418518E-9,
-0.0121897894713504));
#54048=CARTESIAN_POINT('Ctrl Pts',(0.00624999999999999,1.25106139975955E-19,
-0.0121905386717337));
#54049=CARTESIAN_POINT('Ctrl Pts',(0.00624999999999999,3.52129387358801E-30,
-0.0121912878729033));
#54050=CARTESIAN_POINT('Ctrl Pts',(0.00625000000000001,0.0002,0.0119660979437743));
#54051=CARTESIAN_POINT('Ctrl Pts',(0.00625000000000001,0.000177324851142135,
0.0119660979437743));
#54052=CARTESIAN_POINT('Ctrl Pts',(0.00624999999999523,0.000154964926961076,
0.0119704464772441));
#54053=CARTESIAN_POINT('Ctrl Pts',(0.0062499999999948,0.000109689157076455,
0.0119883494086744));
#54054=CARTESIAN_POINT('Ctrl Pts',(0.00624999999999042,8.78747849009445E-5,
0.0120028296365125));
#54055=CARTESIAN_POINT('Ctrl Pts',(0.00624999999998795,4.80234630210931E-5,
0.0120416364875857));
#54056=CARTESIAN_POINT('Ctrl Pts',(0.00625,3.13504886185185E-5,0.0120666257463726));
#54057=CARTESIAN_POINT('Ctrl Pts',(0.00625,6.91440040481353E-6,0.0121239135558641));
#54058=CARTESIAN_POINT('Ctrl Pts',(0.00624999999999996,3.00400145182888E-7,
0.0121564072571944));
#54059=CARTESIAN_POINT('Ctrl Pts',(0.00625,3.33362078410748E-9,0.0121897894713504));
#54060=CARTESIAN_POINT('Ctrl Pts',(0.00625000000000001,1.12063813495364E-19,
0.0121905386717337));
#54061=CARTESIAN_POINT('Ctrl Pts',(0.00625000000000001,2.82537309454408E-30,
0.0121912878729033));
#54062=CARTESIAN_POINT('Origin',(0.0125,0.0002,-4.59242549680257E-18));
#54063=CARTESIAN_POINT('Origin',(0.0125,0.0148,-4.59242549680257E-18));
#54064=CARTESIAN_POINT('Origin',(0.0125,0.0148,-0.0092));
#54065=CARTESIAN_POINT('Origin',(-0.00501982557395217,0.0132,-2.16840434497101E-19));
#54066=CARTESIAN_POINT('Origin',(-0.00501982557395217,0.0132,-0.0012));
#54067=CARTESIAN_POINT('Origin',(-0.000359710594690623,0.0128,-0.0122947390492059));
#54068=CARTESIAN_POINT('Origin',(-0.000359710594690624,0.0128,-0.0122947390492059));
#54069=CARTESIAN_POINT('Origin',(0.0125,0.0012,-4.59242549680257E-18));
#54070=CARTESIAN_POINT('Origin',(0.00625,0.0012,-0.0110556546617557));
#54071=CARTESIAN_POINT('Origin',(0.00625,0.0012,0.0110556546617557));
#54072=CARTESIAN_POINT('Origin',(0.00625,0.0012,-0.0110556546617557));
#54073=CARTESIAN_POINT('Origin',(0.00625,0.0012,-0.0110556546617557));
#54074=CARTESIAN_POINT('Origin',(0.00625,0.0012,0.0110556546617557));
#54075=CARTESIAN_POINT('Origin',(0.00625,0.0012,0.0110556546617557));
#54076=CARTESIAN_POINT('Origin',(0.00625,0.013,-0.0110556546617557));
#54077=CARTESIAN_POINT('Origin',(0.00625,0.0128,-0.0110556546617557));
#54078=CARTESIAN_POINT('Origin',(0.,0.0128,0.));
#54079=CARTESIAN_POINT('Ctrl Pts',(0.00585,0.013,-0.0108197735650983));
#54080=CARTESIAN_POINT('Ctrl Pts',(0.00585411539525861,0.013,-0.0108206833115983));
#54081=CARTESIAN_POINT('Ctrl Pts',(0.00585822747590886,0.0129999328797805,
-0.0108215885294959));
#54082=CARTESIAN_POINT('Ctrl Pts',(0.00586233275092189,0.0129998007010341,
-0.0108224887009578));
#54083=CARTESIAN_POINT('Ctrl Pts',(0.00587772753222075,0.012999305030735,
-0.0108258643439401));
#54084=CARTESIAN_POINT('Ctrl Pts',(0.00589302794065804,0.0129978980557532,
-0.0108291492821836));
#54085=CARTESIAN_POINT('Ctrl Pts',(0.00590815479426512,0.0129956754601165,
-0.0108323086673227));
#54086=CARTESIAN_POINT('Ctrl Pts',(0.00595353535508637,0.0129890076732063,
-0.0108417868227401));
#54087=CARTESIAN_POINT('Ctrl Pts',(0.00599741622959946,0.0129757147702998,
-0.0108502251386974));
#54088=CARTESIAN_POINT('Ctrl Pts',(0.00603890034360096,0.0129532705003051,
-0.0108585674477248));
#54089=CARTESIAN_POINT('Ctrl Pts',(0.00604258782040109,0.0129512754540834,
-0.010859308986305));
#54090=CARTESIAN_POINT('Ctrl Pts',(0.0060462546765892,0.012949201590918,
-0.0108600473853386));
#54091=CARTESIAN_POINT('Ctrl Pts',(0.00604988903132446,0.0129470486489094,
-0.0108607801373845));
#54092=CARTESIAN_POINT('Ctrl Pts',(0.00605329623888877,0.0129450302657765,
-0.0108614670924275));
#54093=CARTESIAN_POINT('Ctrl Pts',(0.00605667487947485,0.012942942385175,
-0.0108621490828373));
#54094=CARTESIAN_POINT('Ctrl Pts',(0.00606001515277547,0.0129407851029365,
-0.0108628240276582));
#54095=CARTESIAN_POINT('Ctrl Pts',(0.00608506720253009,0.0129246054861478,
-0.0108678861138156));
#54096=CARTESIAN_POINT('Ctrl Pts',(0.00610795458539415,0.0129044764792163,
-0.0108725465433551));
#54097=CARTESIAN_POINT('Ctrl Pts',(0.00612457636998883,0.0128808171431182,
-0.0108759551040394));
#54098=CARTESIAN_POINT('Ctrl Pts',(0.00613288726228617,0.0128689874750691,
-0.0108776593843815));
#54099=CARTESIAN_POINT('Ctrl Pts',(0.00613963379098558,0.0128562829565036,
-0.0108790527622001));
#54100=CARTESIAN_POINT('Ctrl Pts',(0.00614430549704848,0.0128427837238958,
-0.0108800251995936));
#54101=CARTESIAN_POINT('Ctrl Pts',(0.00614664135007993,0.0128360341075919,
-0.0108805114182903));
#54102=CARTESIAN_POINT('Ctrl Pts',(0.00614845841299802,0.0128290859420224,
-0.0108808921908321));
#54103=CARTESIAN_POINT('Ctrl Pts',(0.00614969177849169,0.0128219510061821,
-0.0108811518076324));
#54104=CARTESIAN_POINT('Ctrl Pts',(0.00615030846123852,0.012818383538262,
-0.0108812816160325));
#54105=CARTESIAN_POINT('Ctrl Pts',(0.0061507792028679,0.0128147694050756,
-0.0108813811091681));
#54106=CARTESIAN_POINT('Ctrl Pts',(0.00615109578867784,0.0128111103044368,
-0.0108814481716018));
#54107=CARTESIAN_POINT('Ctrl Pts',(0.00615141237448779,0.0128074512037979,
-0.0108815152340356));
#54108=CARTESIAN_POINT('Ctrl Pts',(0.00615157480559109,0.0128037471326604,
-0.0108815498625526));
#54109=CARTESIAN_POINT('Ctrl Pts',(0.00615157480314964,0.0128,-0.0108815498639328));
#54110=CARTESIAN_POINT('Origin',(0.00625,0.013,0.0110556546617557));
#54111=CARTESIAN_POINT('Ctrl Pts',(0.00615157480314962,0.013027940984764,
0.0108815498639328));
#54112=CARTESIAN_POINT('Ctrl Pts',(0.00615579813640361,0.0130304241847365,
0.0108791623225664));
#54113=CARTESIAN_POINT('Ctrl Pts',(0.00616006090484548,0.0130330332307525,
0.0108769553183616));
#54114=CARTESIAN_POINT('Ctrl Pts',(0.00618946868719457,0.0130516853607504,
0.0108630181858572));
#54115=CARTESIAN_POINT('Ctrl Pts',(0.00621674266005389,0.0130722240653073,
0.0108564778400306));
#54116=CARTESIAN_POINT('Ctrl Pts',(0.00628029283816163,0.0131269380048229,
0.0108547662808061));
#54117=CARTESIAN_POINT('Ctrl Pts',(0.00631551530880234,0.0131621010483139,
0.010863362352979));
#54118=CARTESIAN_POINT('Ctrl Pts',(0.00634727221305767,0.0131986668442575,
0.010880901825112));
#54119=CARTESIAN_POINT('Ctrl Pts',(0.00634784951391209,0.0131993334243132,
0.0108812244179529));
#54120=CARTESIAN_POINT('Ctrl Pts',(0.00634842519685039,0.0132,0.0108815498639327));
#54121=CARTESIAN_POINT('Ctrl Pts',(0.00585,0.013,-0.0108197735650983));
#54122=CARTESIAN_POINT('Ctrl Pts',(0.00595507260106555,0.013,-0.0106488169107487));
#54123=CARTESIAN_POINT('Ctrl Pts',(0.00595472383252994,0.0132006638620003,
-0.0106493843688813));
#54124=CARTESIAN_POINT('Ctrl Pts',(0.00599769697787199,0.013,-0.0108524233594023));
#54125=CARTESIAN_POINT('Ctrl Pts',(0.00606053271701144,0.0130441963819751,
-0.0107138924935219));
#54126=CARTESIAN_POINT('Ctrl Pts',(0.00614674466944171,0.0132005816098407,
-0.0107674030221155));
#54127=CARTESIAN_POINT('Ctrl Pts',(0.0061515748771313,0.012913544903149,
-0.0108815498221093));
#54128=CARTESIAN_POINT('Ctrl Pts',(0.00625026576929827,0.0129522781147389,
-0.0108257578692845));
#54129=CARTESIAN_POINT('Ctrl Pts',(0.00634882743980344,0.0130273960626492,
-0.0108817778740662));
#54130=CARTESIAN_POINT('Ctrl Pts',(0.0061515748031496,0.0128,-0.0108815498639328));
#54131=CARTESIAN_POINT('Ctrl Pts',(0.00625026565008664,0.0128,-0.0108257577998508));
#54132=CARTESIAN_POINT('Ctrl Pts',(0.00634882729611851,0.0128,-0.0108817777928458));
#54133=CARTESIAN_POINT('Origin',(0.00585,0.0132,-0.0108197735650983));
#54134=CARTESIAN_POINT('Origin',(0.0125,0.0132,-4.59242549680257E-18));
#54135=CARTESIAN_POINT('Ctrl Pts',(-0.127521969753009,0.00292791234232007,
0.0014375007351075));
#54136=CARTESIAN_POINT('Ctrl Pts',(-0.127521790582252,0.0027228384863398,
0.00149851530284674));
#54137=CARTESIAN_POINT('Ctrl Pts',(-0.127524929244986,0.00279751942631414,
0.0016989922391411));
#54138=CARTESIAN_POINT('Ctrl Pts',(-0.127135930686132,0.00292980295225595,
0.00144284563795753));
#54139=CARTESIAN_POINT('Ctrl Pts',(-0.127128303332053,0.00272468023725761,
0.00150425289890664));
#54140=CARTESIAN_POINT('Ctrl Pts',(-0.127086989041986,0.00279975471284059,
0.00170530652254589));
#54141=CARTESIAN_POINT('Ctrl Pts',(-0.126359755598941,0.00281040271795957,
0.00116400921661829));
#54142=CARTESIAN_POINT('Ctrl Pts',(-0.126391171205071,0.00262787967136648,
0.00125349479954768));
#54143=CARTESIAN_POINT('Ctrl Pts',(-0.126205867042022,0.00265838342822912,
0.00137542120560247));
#54144=CARTESIAN_POINT('Ctrl Pts',(-0.125844810804675,0.00261243102946704,
2.73686784602689E-5));
#54145=CARTESIAN_POINT('Ctrl Pts',(-0.125809482099816,0.00243981891809853,
3.02504277461029E-5));
#54146=CARTESIAN_POINT('Ctrl Pts',(-0.125622107008347,0.00242419343546421,
3.23331464449823E-5));
#54147=CARTESIAN_POINT('Ctrl Pts',(-0.126324661426851,0.00279922894991231,
-0.00113315917795553));
#54148=CARTESIAN_POINT('Ctrl Pts',(-0.126353424833284,0.00261785874660316,
-0.00122287857653872));
#54149=CARTESIAN_POINT('Ctrl Pts',(-0.126166065338315,0.00264516117224187,
-0.00133894667362534));
#54150=CARTESIAN_POINT('Ctrl Pts',(-0.127475667560966,0.00298937709191257,
-0.00158152248003426));
#54151=CARTESIAN_POINT('Ctrl Pts',(-0.127477698215336,0.00277625525457815,
-0.00163733766341933));
#54152=CARTESIAN_POINT('Ctrl Pts',(-0.127472373507598,0.00287024649410682,
-0.00186926883315216));
#54153=CARTESIAN_POINT('Ctrl Pts',(-0.128639088312426,0.00281072577948569,
-0.0011657258572821));
#54154=CARTESIAN_POINT('Ctrl Pts',(-0.128607647449207,0.00262816948297644,
-0.00125530022942571));
#54155=CARTESIAN_POINT('Ctrl Pts',(-0.12879282120482,0.00265876571215961,
-0.00137744992107518));
#54156=CARTESIAN_POINT('Ctrl Pts',(-0.129155327766085,0.00261238743571346,
-2.56552014421315E-5));
#54157=CARTESIAN_POINT('Ctrl Pts',(-0.129190650203713,0.00243978444592542,
-2.85609443698061E-5));
#54158=CARTESIAN_POINT('Ctrl Pts',(-0.129378050332955,0.00242414178609797,
-3.03066921534991E-5));
#54159=CARTESIAN_POINT('Ctrl Pts',(-0.128676003572727,0.00279905892909026,
0.00113193946402897));
#54160=CARTESIAN_POINT('Ctrl Pts',(-0.128647225777398,0.00261770650436977,
0.00122160652879797));
#54161=CARTESIAN_POINT('Ctrl Pts',(-0.12883468948467,0.00264495997721762,
0.00133750508047789));
#54162=CARTESIAN_POINT('Ctrl Pts',(-0.127908008885461,0.00292602173206305,
0.00143215583134956));
#54163=CARTESIAN_POINT('Ctrl Pts',(-0.127914748354504,0.00272099921368907,
0.00149278542731802));
#54164=CARTESIAN_POINT('Ctrl Pts',(-0.127962875152517,0.00279528411067127,
0.00169267787348758));
#54165=CARTESIAN_POINT('Ctrl Pts',(-0.127521969753009,0.00292791234232007,
0.0014375007351075));
#54166=CARTESIAN_POINT('Ctrl Pts',(-0.127521790582252,0.0027228384863398,
0.00149851530284674));
#54167=CARTESIAN_POINT('Ctrl Pts',(-0.127524929244986,0.00279751942631414,
0.0016989922391411));
#54168=CARTESIAN_POINT('Ctrl Pts',(-0.107521969753009,0.00292791234232008,
0.0014375007351075));
#54169=CARTESIAN_POINT('Ctrl Pts',(-0.107521790582252,0.00272283848633961,
0.00149851530284679));
#54170=CARTESIAN_POINT('Ctrl Pts',(-0.107524929244986,0.00279751942631421,
0.00169899223914127));
#54171=CARTESIAN_POINT('Ctrl Pts',(-0.107135930686132,0.00292980295225595,
0.00144284563795752));
#54172=CARTESIAN_POINT('Ctrl Pts',(-0.107128303332053,0.00272468023725742,
0.00150425289890669));
#54173=CARTESIAN_POINT('Ctrl Pts',(-0.107086989041985,0.00279975471284066,
0.00170530652254606));
#54174=CARTESIAN_POINT('Ctrl Pts',(-0.106359755598941,0.00281040271795956,
0.00116400921661828));
#54175=CARTESIAN_POINT('Ctrl Pts',(-0.106391171205071,0.00262787967136631,
0.00125349479954775));
#54176=CARTESIAN_POINT('Ctrl Pts',(-0.106205867042022,0.00265838342822915,
0.00137542120560257));
#54177=CARTESIAN_POINT('Ctrl Pts',(-0.105844810804675,0.00261243102946704,
2.73686784602542E-5));
#54178=CARTESIAN_POINT('Ctrl Pts',(-0.105809482099816,0.00243981891809839,
3.02504277460862E-5));
#54179=CARTESIAN_POINT('Ctrl Pts',(-0.105622107008346,0.00242419343546419,
3.23331464449678E-5));
#54180=CARTESIAN_POINT('Ctrl Pts',(-0.106324661426851,0.00279922894991231,
-0.00113315917795554));
#54181=CARTESIAN_POINT('Ctrl Pts',(-0.106353424833284,0.002617858746603,
-0.00122287857653881));
#54182=CARTESIAN_POINT('Ctrl Pts',(-0.106166065338315,0.0026451611722419,
-0.00133894667362546));
#54183=CARTESIAN_POINT('Ctrl Pts',(-0.107475667560966,0.00298937709191257,
-0.00158152248003427));
#54184=CARTESIAN_POINT('Ctrl Pts',(-0.107477698215336,0.00277625525457795,
-0.00163733766341938));
#54185=CARTESIAN_POINT('Ctrl Pts',(-0.107472373507598,0.0028702464941069,
-0.00186926883315237));
#54186=CARTESIAN_POINT('Ctrl Pts',(-0.108639088312426,0.00281072577948568,
-0.00116572585728207));
#54187=CARTESIAN_POINT('Ctrl Pts',(-0.108607647449207,0.00262816948297624,
-0.00125530022942576));
#54188=CARTESIAN_POINT('Ctrl Pts',(-0.10879282120482,0.00265876571215962,
-0.00137744992107526));
#54189=CARTESIAN_POINT('Ctrl Pts',(-0.109155327766085,0.00261238743571347,
-2.5655201442127E-5));
#54190=CARTESIAN_POINT('Ctrl Pts',(-0.109190650203713,0.00243978444592529,
-2.85609443698138E-5));
#54191=CARTESIAN_POINT('Ctrl Pts',(-0.109378050332955,0.00242414178609796,
-3.0306692153495E-5));
#54192=CARTESIAN_POINT('Ctrl Pts',(-0.108676003572727,0.00279905892909026,
0.00113193946402899));
#54193=CARTESIAN_POINT('Ctrl Pts',(-0.108647225777398,0.0026177065043696,
0.00122160652879808));
#54194=CARTESIAN_POINT('Ctrl Pts',(-0.108834689484669,0.00264495997721766,
0.00133750508047803));
#54195=CARTESIAN_POINT('Ctrl Pts',(-0.107908008885461,0.00292602173206305,
0.00143215583134956));
#54196=CARTESIAN_POINT('Ctrl Pts',(-0.107914748354504,0.00272099921368888,
0.00149278542731809));
#54197=CARTESIAN_POINT('Ctrl Pts',(-0.107962875152517,0.00279528411067133,
0.00169267787348776));
#54198=CARTESIAN_POINT('Ctrl Pts',(-0.107521969753009,0.00292791234232008,
0.0014375007351075));
#54199=CARTESIAN_POINT('Ctrl Pts',(-0.107521790582252,0.00272283848633961,
0.00149851530284679));
#54200=CARTESIAN_POINT('Ctrl Pts',(-0.107524929244986,0.00279751942631421,
0.00169899223914127));
#54201=CARTESIAN_POINT('Ctrl Pts',(-0.087521969753009,0.00292791234232007,
0.0014375007351075));
#54202=CARTESIAN_POINT('Ctrl Pts',(-0.0875217905822522,0.00272283848633951,
0.00149851530284683));
#54203=CARTESIAN_POINT('Ctrl Pts',(-0.0875249292449862,0.00279751942631424,
0.00169899223914137));
#54204=CARTESIAN_POINT('Ctrl Pts',(-0.0871359306861318,0.00292980295225596,
0.00144284563795755));
#54205=CARTESIAN_POINT('Ctrl Pts',(-0.087128303332053,0.00272468023725732,
0.00150425289890676));
#54206=CARTESIAN_POINT('Ctrl Pts',(-0.0870869890419856,0.0027997547128407,
0.00170530652254619));
#54207=CARTESIAN_POINT('Ctrl Pts',(-0.0863597555989418,0.00281040271795959,
0.00116400921661838));
#54208=CARTESIAN_POINT('Ctrl Pts',(-0.0863911712050714,0.00262787967136625,
0.00125349479954789));
#54209=CARTESIAN_POINT('Ctrl Pts',(-0.0862058670420218,0.0026583834282292,
0.00137542120560275));
#54210=CARTESIAN_POINT('Ctrl Pts',(-0.0858448108046749,0.00261243102946704,
2.73686784603756E-5));
#54211=CARTESIAN_POINT('Ctrl Pts',(-0.0858094820998151,0.00243981891809831,
3.02504277462256E-5));
#54212=CARTESIAN_POINT('Ctrl Pts',(-0.0856221070083461,0.00242419343546418,
3.23331464451119E-5));
#54213=CARTESIAN_POINT('Ctrl Pts',(-0.0863246614268507,0.00279922894991229,
-0.00113315917795547));
#54214=CARTESIAN_POINT('Ctrl Pts',(-0.0863534248332843,0.00261785874660288,
-0.00122287857653878));
#54215=CARTESIAN_POINT('Ctrl Pts',(-0.0861660653383145,0.00264516117224188,
-0.00133894667362542));
#54216=CARTESIAN_POINT('Ctrl Pts',(-0.0874756675609659,0.00298937709191257,
-0.00158152248003427));
#54217=CARTESIAN_POINT('Ctrl Pts',(-0.0874776982153359,0.00277625525457783,
-0.00163733766341943));
#54218=CARTESIAN_POINT('Ctrl Pts',(-0.0874723735075982,0.00287024649410694,
-0.00186926883315248));
#54219=CARTESIAN_POINT('Ctrl Pts',(-0.0886390883124264,0.00281072577948571,
-0.00116572585728214));
#54220=CARTESIAN_POINT('Ctrl Pts',(-0.088607647449207,0.00262816948297619,
-0.00125530022942588));
#54221=CARTESIAN_POINT('Ctrl Pts',(-0.0887928212048197,0.00265876571215967,
-0.00137744992107541));
#54222=CARTESIAN_POINT('Ctrl Pts',(-0.0891553277660854,0.00261238743571347,
-2.56552014422575E-5));
#54223=CARTESIAN_POINT('Ctrl Pts',(-0.0891906502037131,0.00243978444592521,
-2.85609443699477E-5));
#54224=CARTESIAN_POINT('Ctrl Pts',(-0.0893780503329556,0.00242414178609795,
-3.030669215365E-5));
#54225=CARTESIAN_POINT('Ctrl Pts',(-0.0886760035727276,0.00279905892909023,
0.0011319394640289));
#54226=CARTESIAN_POINT('Ctrl Pts',(-0.0886472257773982,0.0026177065043695,
0.00122160652879803));
#54227=CARTESIAN_POINT('Ctrl Pts',(-0.0888346894846697,0.00264495997721763,
0.00133750508047797));
#54228=CARTESIAN_POINT('Ctrl Pts',(-0.0879080088854605,0.00292602173206304,
0.00143215583134954));
#54229=CARTESIAN_POINT('Ctrl Pts',(-0.0879147483545036,0.00272099921368876,
0.00149278542731808));
#54230=CARTESIAN_POINT('Ctrl Pts',(-0.0879628751525175,0.00279528411067136,
0.00169267787348782));
#54231=CARTESIAN_POINT('Ctrl Pts',(-0.087521969753009,0.00292791234232007,
0.0014375007351075));
#54232=CARTESIAN_POINT('Ctrl Pts',(-0.0875217905822522,0.00272283848633951,
0.00149851530284683));
#54233=CARTESIAN_POINT('Ctrl Pts',(-0.0875249292449862,0.00279751942631424,
0.00169899223914137));
#54234=CARTESIAN_POINT('Ctrl Pts',(-0.0675219697530089,0.00292791234232007,
0.0014375007351075));
#54235=CARTESIAN_POINT('Ctrl Pts',(-0.0675217905822521,0.00272283848633946,
0.00149851530284684));
#54236=CARTESIAN_POINT('Ctrl Pts',(-0.0675249292449862,0.00279751942631426,
0.00169899223914141));
#54237=CARTESIAN_POINT('Ctrl Pts',(-0.0671359306861318,0.00292980295225596,
0.00144284563795754));
#54238=CARTESIAN_POINT('Ctrl Pts',(-0.0671283033320531,0.00272468023725727,
0.00150425289890677));
#54239=CARTESIAN_POINT('Ctrl Pts',(-0.0670869890419856,0.00279975471284072,
0.00170530652254623));
#54240=CARTESIAN_POINT('Ctrl Pts',(-0.0663597555989418,0.00281040271795959,
0.00116400921661836));
#54241=CARTESIAN_POINT('Ctrl Pts',(-0.0663911712050714,0.00262787967136621,
0.00125349479954789));
#54242=CARTESIAN_POINT('Ctrl Pts',(-0.0662058670420217,0.0026583834282292,
0.00137542120560276));
#54243=CARTESIAN_POINT('Ctrl Pts',(-0.065844810804675,0.00261243102946704,
2.73686784603625E-5));
#54244=CARTESIAN_POINT('Ctrl Pts',(-0.0658094820998151,0.00243981891809827,
3.02504277462119E-5));
#54245=CARTESIAN_POINT('Ctrl Pts',(-0.0656221070083461,0.00242419343546418,
3.23331464450973E-5));
#54246=CARTESIAN_POINT('Ctrl Pts',(-0.0663246614268507,0.00279922894991229,
-0.00113315917795546));
#54247=CARTESIAN_POINT('Ctrl Pts',(-0.0663534248332843,0.00261785874660285,
-0.00122287857653879));
#54248=CARTESIAN_POINT('Ctrl Pts',(-0.0661660653383145,0.00264516117224189,
-0.00133894667362545));
#54249=CARTESIAN_POINT('Ctrl Pts',(-0.067475667560966,0.00298937709191257,
-0.00158152248003427));
#54250=CARTESIAN_POINT('Ctrl Pts',(-0.0674776982153359,0.00277625525457778,
-0.00163733766341944));
#54251=CARTESIAN_POINT('Ctrl Pts',(-0.0674723735075983,0.00287024649410697,
-0.00186926883315253));
#54252=CARTESIAN_POINT('Ctrl Pts',(-0.0686390883124264,0.00281072577948571,
-0.00116572585728214));
#54253=CARTESIAN_POINT('Ctrl Pts',(-0.068607647449207,0.00262816948297615,
-0.0012553002294259));
#54254=CARTESIAN_POINT('Ctrl Pts',(-0.0687928212048197,0.00265876571215968,
-0.00137744992107544));
#54255=CARTESIAN_POINT('Ctrl Pts',(-0.0691553277660854,0.00261238743571347,
-2.56552014422452E-5));
#54256=CARTESIAN_POINT('Ctrl Pts',(-0.0691906502037132,0.00243978444592516,
-2.85609443699341E-5));
#54257=CARTESIAN_POINT('Ctrl Pts',(-0.0693780503329557,0.00242414178609795,
-3.03066921536361E-5));
#54258=CARTESIAN_POINT('Ctrl Pts',(-0.0686760035727276,0.00279905892909023,
0.00113193946402892));
#54259=CARTESIAN_POINT('Ctrl Pts',(-0.0686472257773982,0.00261770650436945,
0.00122160652879807));
#54260=CARTESIAN_POINT('Ctrl Pts',(-0.0688346894846698,0.00264495997721765,
0.00133750508047802));
#54261=CARTESIAN_POINT('Ctrl Pts',(-0.0679080088854605,0.00292602173206304,
0.00143215583134953));
#54262=CARTESIAN_POINT('Ctrl Pts',(-0.0679147483545036,0.00272099921368871,
0.0014927854273181));
#54263=CARTESIAN_POINT('Ctrl Pts',(-0.0679628751525174,0.00279528411067137,
0.00169267787348788));
#54264=CARTESIAN_POINT('Ctrl Pts',(-0.0675219697530089,0.00292791234232007,
0.0014375007351075));
#54265=CARTESIAN_POINT('Ctrl Pts',(-0.0675217905822521,0.00272283848633946,
0.00149851530284684));
#54266=CARTESIAN_POINT('Ctrl Pts',(-0.0675249292449862,0.00279751942631426,
0.00169899223914141));
#54267=CARTESIAN_POINT('Ctrl Pts',(-0.047521969753009,0.00292791234232007,
0.0014375007351075));
#54268=CARTESIAN_POINT('Ctrl Pts',(-0.0475217905822521,0.00272283848633948,
0.00149851530284684));
#54269=CARTESIAN_POINT('Ctrl Pts',(-0.0475249292449862,0.00279751942631425,
0.00169899223914139));
#54270=CARTESIAN_POINT('Ctrl Pts',(-0.0471359306861318,0.00292980295225596,
0.00144284563795755));
#54271=CARTESIAN_POINT('Ctrl Pts',(-0.0471283033320531,0.0027246802372573,
0.00150425289890676));
#54272=CARTESIAN_POINT('Ctrl Pts',(-0.0470869890419856,0.00279975471284071,
0.00170530652254621));
#54273=CARTESIAN_POINT('Ctrl Pts',(-0.0463597555989418,0.00281040271795959,
0.00116400921661837));
#54274=CARTESIAN_POINT('Ctrl Pts',(-0.0463911712050714,0.00262787967136623,
0.00125349479954789));
#54275=CARTESIAN_POINT('Ctrl Pts',(-0.0462058670420217,0.0026583834282292,
0.00137542120560276));
#54276=CARTESIAN_POINT('Ctrl Pts',(-0.0458448108046749,0.00261243102946703,
2.73686784603569E-5));
#54277=CARTESIAN_POINT('Ctrl Pts',(-0.0458094820998151,0.00243981891809829,
3.02504277461982E-5));
#54278=CARTESIAN_POINT('Ctrl Pts',(-0.0456221070083461,0.00242419343546418,
3.23331464450899E-5));
#54279=CARTESIAN_POINT('Ctrl Pts',(-0.0463246614268507,0.00279922894991229,
-0.00113315917795547));
#54280=CARTESIAN_POINT('Ctrl Pts',(-0.0463534248332843,0.00261785874660286,
-0.00122287857653879));
#54281=CARTESIAN_POINT('Ctrl Pts',(-0.0461660653383145,0.00264516117224189,
-0.00133894667362545));
#54282=CARTESIAN_POINT('Ctrl Pts',(-0.047475667560966,0.00298937709191257,
-0.00158152248003427));
#54283=CARTESIAN_POINT('Ctrl Pts',(-0.0474776982153359,0.0027762552545778,
-0.00163733766341943));
#54284=CARTESIAN_POINT('Ctrl Pts',(-0.0474723735075983,0.00287024649410696,
-0.00186926883315251));
#54285=CARTESIAN_POINT('Ctrl Pts',(-0.0486390883124264,0.00281072577948571,
-0.00116572585728214));
#54286=CARTESIAN_POINT('Ctrl Pts',(-0.048607647449207,0.00262816948297617,
-0.00125530022942588));
#54287=CARTESIAN_POINT('Ctrl Pts',(-0.0487928212048197,0.00265876571215968,
-0.00137744992107542));
#54288=CARTESIAN_POINT('Ctrl Pts',(-0.0491553277660853,0.00261238743571346,
-2.56552014422379E-5));
#54289=CARTESIAN_POINT('Ctrl Pts',(-0.0491906502037132,0.00243978444592517,
-2.85609443699274E-5));
#54290=CARTESIAN_POINT('Ctrl Pts',(-0.0493780503329557,0.00242414178609795,
-3.03066921536269E-5));
#54291=CARTESIAN_POINT('Ctrl Pts',(-0.0486760035727277,0.00279905892909024,
0.00113193946402892));
#54292=CARTESIAN_POINT('Ctrl Pts',(-0.0486472257773982,0.00261770650436948,
0.00122160652879805));
#54293=CARTESIAN_POINT('Ctrl Pts',(-0.0488346894846697,0.00264495997721764,
0.00133750508047801));
#54294=CARTESIAN_POINT('Ctrl Pts',(-0.0479080088854605,0.00292602173206304,
0.00143215583134954));
#54295=CARTESIAN_POINT('Ctrl Pts',(-0.0479147483545036,0.00272099921368874,
0.00149278542731809));
#54296=CARTESIAN_POINT('Ctrl Pts',(-0.0479628751525174,0.00279528411067136,
0.00169267787348785));
#54297=CARTESIAN_POINT('Ctrl Pts',(-0.047521969753009,0.00292791234232007,
0.0014375007351075));
#54298=CARTESIAN_POINT('Ctrl Pts',(-0.0475217905822521,0.00272283848633948,
0.00149851530284684));
#54299=CARTESIAN_POINT('Ctrl Pts',(-0.0475249292449862,0.00279751942631425,
0.00169899223914139));
#54300=CARTESIAN_POINT('Origin',(-0.0183187040774608,0.000201195130235789,
0.0081064157789351));
#54301=CARTESIAN_POINT('Origin',(-0.0192596558562786,-0.000820619857582921,
0.00981391272232187));
#54302=CARTESIAN_POINT('Ctrl Pts',(-0.0167335787825944,0.000199999999999998,
0.0092755050776766));
#54303=CARTESIAN_POINT('Ctrl Pts',(-0.0167989534819831,0.000445675548177814,
0.00923685991535881));
#54304=CARTESIAN_POINT('Ctrl Pts',(-0.0168953032845749,0.000683360688027424,
0.00925546810437307));
#54305=CARTESIAN_POINT('Ctrl Pts',(-0.0168884171052221,0.000194945401620732,
0.00918397498779601));
#54306=CARTESIAN_POINT('Ctrl Pts',(-0.0169566045154461,0.000427726110919411,
0.00915087413831594));
#54307=CARTESIAN_POINT('Ctrl Pts',(-0.0170529779122477,0.000652022804612772,
0.00916927738948391));
#54308=CARTESIAN_POINT('Ctrl Pts',(-0.0171958663208298,0.000184166395058654,
0.00900179253952732));
#54309=CARTESIAN_POINT('Ctrl Pts',(-0.0172687191497198,0.000389409848041071,
0.00897906560874024));
#54310=CARTESIAN_POINT('Ctrl Pts',(-0.0173642546158974,0.000585686088741027,
0.00899657312123159));
#54311=CARTESIAN_POINT('Ctrl Pts',(-0.0176463723131326,0.000165442575407028,
0.00873284458653405));
#54312=CARTESIAN_POINT('Ctrl Pts',(-0.0177222065528446,0.000322469294492184,
0.00872197465762366));
#54313=CARTESIAN_POINT('Ctrl Pts',(-0.0178122797421618,0.000471566164156617,
0.00873578171227763));
#54314=CARTESIAN_POINT('Ctrl Pts',(-0.0180089482080531,0.00014654221914008,
0.00851355328316542));
#54315=CARTESIAN_POINT('Ctrl Pts',(-0.0180815789893364,0.00025422082507978,
0.00850731258360253));
#54316=CARTESIAN_POINT('Ctrl Pts',(-0.0181617121620799,0.000356444186374595,
0.00851412153872697));
#54317=CARTESIAN_POINT('Ctrl Pts',(-0.0182653366435107,0.000127597262669883,
0.00835462058997495));
#54318=CARTESIAN_POINT('Ctrl Pts',(-0.0183286217321492,0.000184709407290683,
0.00834469986689284));
#54319=CARTESIAN_POINT('Ctrl Pts',(-0.0183949042260683,0.000239045421227612,
0.00834000019373098));
#54320=CARTESIAN_POINT('Ctrl Pts',(-0.0183638281572847,0.000113747397695859,
0.00828933270869108));
#54321=CARTESIAN_POINT('Ctrl Pts',(-0.018416358529888,0.000132790739820186,
0.00827019203209158));
#54322=CARTESIAN_POINT('Ctrl Pts',(-0.0184701394209955,0.000150558685463742,
0.00825332284927026));
#54323=CARTESIAN_POINT('Ctrl Pts',(-0.0183575213134859,0.000106149127372226,
0.00828837051540356));
#54324=CARTESIAN_POINT('Ctrl Pts',(-0.0184024414311689,0.000103709091286823,
0.00826031051413278));
#54325=CARTESIAN_POINT('Ctrl Pts',(-0.0184485607971002,9.99542717525335E-5,
0.00823442538642541));
#54326=CARTESIAN_POINT('Origin',(-0.0177513235169945,0.000199999999999973,
0.0109971890369446));
#54327=CARTESIAN_POINT('Ctrl Pts',(-0.0151447495921968,0.00165220181413017,
0.0102147149330532));
#54328=CARTESIAN_POINT('Ctrl Pts',(-0.0152060889391142,0.00159854195139627,
0.0101784552021597));
#54329=CARTESIAN_POINT('Ctrl Pts',(-0.0152709311364255,0.00154471125155936,
0.0101488045799563));
#54330=CARTESIAN_POINT('Ctrl Pts',(-0.0149661476183632,0.00131323993358782,
0.0103202925086844));
#54331=CARTESIAN_POINT('Ctrl Pts',(-0.015026744798365,0.00132849279769074,
0.0102844714970778));
#54332=CARTESIAN_POINT('Ctrl Pts',(-0.0150879954762257,0.00134387673222698,
0.0102498911921733));
#54333=CARTESIAN_POINT('Ctrl Pts',(-0.0152846624930786,0.000915866669368474,
0.0101320077571046));
#54334=CARTESIAN_POINT('Ctrl Pts',(-0.0153480148170758,0.00101115245864742,
0.0100945580882847));
#54335=CARTESIAN_POINT('Ctrl Pts',(-0.0154164122352271,0.00110671945758542,
0.010068445155131));
#54336=CARTESIAN_POINT('Ctrl Pts',(-0.0157806659000851,0.00060625922996491,
0.00983880362227603));
#54337=CARTESIAN_POINT('Ctrl Pts',(-0.0158458549228214,0.000765968566367971,
0.00980026821960143));
#54338=CARTESIAN_POINT('Ctrl Pts',(-0.0159248091463299,0.000923634413820413,
0.00978867700564263));
#54339=CARTESIAN_POINT('Ctrl Pts',(-0.0163137554251612,0.000352348673268969,
0.00952367664778722));
#54340=CARTESIAN_POINT('Ctrl Pts',(-0.0163805746329843,0.000566476009334006,
0.00948417758842814));
#54341=CARTESIAN_POINT('Ctrl Pts',(-0.0164702186466373,0.000775802287379282,
0.00948955553669219));
#54342=CARTESIAN_POINT('Ctrl Pts',(-0.0167006112850335,0.000209372126995855,
0.00929499326357058));
#54343=CARTESIAN_POINT('Ctrl Pts',(-0.0167673355456445,0.000456254808588579,
0.00925555033064982));
#54344=CARTESIAN_POINT('Ctrl Pts',(-0.0168647148508793,0.000695249121534255,
0.00927416129940651));
#54345=CARTESIAN_POINT('Ctrl Pts',(-0.0169280464492866,0.00013215739489152,
0.0091605487625401));
#54346=CARTESIAN_POINT('Ctrl Pts',(-0.0169943093597287,0.000397467558198914,
0.00912137854910013));
#54347=CARTESIAN_POINT('Ctrl Pts',(-0.0170961872877718,0.000652854831667682,
0.00914812433229151));
#54348=CARTESIAN_POINT('Origin',(-0.0160885892837263,0.00138685515994303,
0.0119750415244209));
#54349=CARTESIAN_POINT('Origin',(-0.0160872238541987,0.00194341959324476,
0.0119756128465044));
#54350=CARTESIAN_POINT('Origin',(-0.0160859565839347,0.00250003209534414,
0.0119763645202741));
#54351=CARTESIAN_POINT('Origin',(-0.0159726371414409,0.00698837807496495,
0.0117686012574936));
#54352=CARTESIAN_POINT('Origin',(-0.0159723098794419,0.0114765413480154,
0.0117691396498924));
#54353=CARTESIAN_POINT('Ctrl Pts',(-0.0177441069319941,0.0132668179233314,
0.00867814822976128));
#54354=CARTESIAN_POINT('Ctrl Pts',(-0.0178357661804268,0.0129212136767161,
0.00862396539501086));
#54355=CARTESIAN_POINT('Ctrl Pts',(-0.0179860636964262,0.0125974920464792,
0.0086822238418441));
#54356=CARTESIAN_POINT('Ctrl Pts',(-0.0174438743220729,0.013159204780945,
0.00885562572567315));
#54357=CARTESIAN_POINT('Ctrl Pts',(-0.0175359527092885,0.012837517340567,
0.00880119512403525));
#54358=CARTESIAN_POINT('Ctrl Pts',(-0.0176783448733239,0.0125332124555831,
0.0088462220838624));
#54359=CARTESIAN_POINT('Ctrl Pts',(-0.0169089556228614,0.012949243145523,
0.0091718339859198));
#54360=CARTESIAN_POINT('Ctrl Pts',(-0.0169998667382091,0.0126714308781741,
0.00911809339755667));
#54361=CARTESIAN_POINT('Ctrl Pts',(-0.0171277195811297,0.012404131932755,
0.00914119593583115));
#54362=CARTESIAN_POINT('Ctrl Pts',(-0.0161568173119193,0.012587525687478,
0.00961644799383991));
#54363=CARTESIAN_POINT('Ctrl Pts',(-0.0162421507775504,0.0123793205558015,
0.00956600454000768));
#54364=CARTESIAN_POINT('Ctrl Pts',(-0.0163495719378372,0.0121753390197973,
0.0095617513260173));
#54365=CARTESIAN_POINT('Ctrl Pts',(-0.0156006461865971,0.0122442363754161,
0.00994521927103916));
#54366=CARTESIAN_POINT('Ctrl Pts',(-0.015679742844943,0.0120991303276778,
0.00989846260172805));
#54367=CARTESIAN_POINT('Ctrl Pts',(-0.0157711425114264,0.0119553567280747,
0.00987670168726923));
#54368=CARTESIAN_POINT('Ctrl Pts',(-0.0151605030169284,0.0118388471177341,
0.0102054025589772));
#54369=CARTESIAN_POINT('Ctrl Pts',(-0.0152322413348173,0.0117684582609837,
0.0101629956498054));
#54370=CARTESIAN_POINT('Ctrl Pts',(-0.0153083644911994,0.0116978452664201,
0.0101297128986875));
#54371=CARTESIAN_POINT('Ctrl Pts',(-0.0149980581487341,0.0114857175403946,
0.0103014291313018));
#54372=CARTESIAN_POINT('Ctrl Pts',(-0.015063582233244,0.011482507293876,
0.0102626956624571));
#54373=CARTESIAN_POINT('Ctrl Pts',(-0.0151307389308278,0.0114792190702809,
0.0102268871915435));
#54374=CARTESIAN_POINT('Ctrl Pts',(-0.0151300208199999,0.0112383215488602,
0.0102234216008868));
#54375=CARTESIAN_POINT('Ctrl Pts',(-0.0151931734358564,0.011286730281564,
0.0101860899861687));
#54376=CARTESIAN_POINT('Ctrl Pts',(-0.0152598713370855,0.0113352008367595,
0.0101554707885479));
#54377=CARTESIAN_POINT('Origin',(-0.0185790388714426,0.0132,0.010507898921278));
#54378=CARTESIAN_POINT('Ctrl Pts',(-0.0194832368868348,0.0133370288977843,
0.0075874409832765));
#54379=CARTESIAN_POINT('Ctrl Pts',(-0.0195033028657649,0.0134070877928086,
0.00749672395384876));
#54380=CARTESIAN_POINT('Ctrl Pts',(-0.0195278886848258,0.013483568243638,
0.00741351892276558));
#54381=CARTESIAN_POINT('Ctrl Pts',(-0.0197507818214645,0.0133230133512749,
0.00744372563506592));
#54382=CARTESIAN_POINT('Ctrl Pts',(-0.0198087010863357,0.0133342024701371,
0.00741111088576182));
#54383=CARTESIAN_POINT('Ctrl Pts',(-0.0198664298167596,0.0133454743880182,
0.00737820542396837));
#54384=CARTESIAN_POINT('Ctrl Pts',(-0.0195727782976753,0.013304973067155,
0.00756333620365235));
#54385=CARTESIAN_POINT('Ctrl Pts',(-0.0196609338252826,0.0132429781941271,
0.00755714489238573));
#54386=CARTESIAN_POINT('Ctrl Pts',(-0.0197531840062628,0.0131867131153442,
0.00755729857743586));
#54387=CARTESIAN_POINT('Ctrl Pts',(-0.0191783091553242,0.0132841167698863,
0.00780994181632697));
#54388=CARTESIAN_POINT('Ctrl Pts',(-0.019287093290927,0.0131399142662646,
0.00781104542072873));
#54389=CARTESIAN_POINT('Ctrl Pts',(-0.0194095336013034,0.0130093728973814,
0.00783616050338385));
#54390=CARTESIAN_POINT('Ctrl Pts',(-0.018716108312103,0.0132659245783802,
0.00809240117807621));
#54391=CARTESIAN_POINT('Ctrl Pts',(-0.0188305568961298,0.0130510820638524,
0.00808446146002699));
#54392=CARTESIAN_POINT('Ctrl Pts',(-0.0189716132786577,0.0128562445176172,
0.00812308749445927));
#54393=CARTESIAN_POINT('Ctrl Pts',(-0.0180691343143712,0.0132449233701698,
0.00848290936225995));
#54394=CARTESIAN_POINT('Ctrl Pts',(-0.018175922042617,0.0129492634754963,
0.0084494961400988));
#54395=CARTESIAN_POINT('Ctrl Pts',(-0.0183289512107979,0.0126768011770632,
0.00849786999827214));
#54396=CARTESIAN_POINT('Ctrl Pts',(-0.0175928450092797,0.0132323460363387,
0.00876779160005616));
#54397=CARTESIAN_POINT('Ctrl Pts',(-0.0176865783709503,0.012888524988684,
0.00870884960536136));
#54398=CARTESIAN_POINT('Ctrl Pts',(-0.0178402497241257,0.0125657338012786,
0.00876073459359184));
#54399=CARTESIAN_POINT('Ctrl Pts',(-0.0173143432412806,0.0132257325396149,
0.00893390798783256));
#54400=CARTESIAN_POINT('Ctrl Pts',(-0.0173993515205757,0.0128564725832721,
0.00885895734423144));
#54401=CARTESIAN_POINT('Ctrl Pts',(-0.0175519300652605,0.0125057034540625,
0.00891265565385289));
#54402=CARTESIAN_POINT('Origin',(-0.0204666233347745,0.0145154811894642,
0.00888488367021892));
#54403=CARTESIAN_POINT('Origin',(-0.0197053153855647,0.013197642208147,
0.00729146575043895));
#54404=CARTESIAN_POINT('Origin',(-0.0197429273583666,0.0131963056902179,
-0.00726122969914678));
#54405=CARTESIAN_POINT('Origin',(-0.0206317819659218,0.0145314876015483,
-0.00877324474953166));
#54406=CARTESIAN_POINT('Ctrl Pts',(-0.0174781162006161,0.013194947177096,
-0.0088353455161641));
#54407=CARTESIAN_POINT('Ctrl Pts',(-0.0175651094419168,0.0128357627682235,
-0.00876647747827708));
#54408=CARTESIAN_POINT('Ctrl Pts',(-0.0177156087422018,0.0124953957683154,
-0.00881967683902286));
#54409=CARTESIAN_POINT('Ctrl Pts',(-0.0177606237719999,0.0132038679035857,
-0.00866858423663555));
#54410=CARTESIAN_POINT('Ctrl Pts',(-0.0178559242864338,0.0128699235417939,
-0.00861502263776792));
#54411=CARTESIAN_POINT('Ctrl Pts',(-0.0180074828014301,0.0125570715094477,
-0.00866647111554646));
#54412=CARTESIAN_POINT('Ctrl Pts',(-0.0182385379182696,0.0132206414165277,
-0.00838543393250545));
#54413=CARTESIAN_POINT('Ctrl Pts',(-0.0183460042794801,0.0129337933037081,
-0.00835600790222576));
#54414=CARTESIAN_POINT('Ctrl Pts',(-0.0184968930862299,0.0126698469468547,
-0.00840408638510566));
#54415=CARTESIAN_POINT('Ctrl Pts',(-0.0188888690299216,0.0132487916607732,
-0.00799516388057441));
#54416=CARTESIAN_POINT('Ctrl Pts',(-0.0190027510573474,0.013040834514991,
-0.00798953516750174));
#54417=CARTESIAN_POINT('Ctrl Pts',(-0.0191416149041577,0.0128523958496762,
-0.00802801969736298));
#54418=CARTESIAN_POINT('Ctrl Pts',(-0.0193515121113206,0.0132730699882502,
-0.00771267516059409));
#54419=CARTESIAN_POINT('Ctrl Pts',(-0.0194591200995059,0.0131333169586524,
-0.00771518874178041));
#54420=CARTESIAN_POINT('Ctrl Pts',(-0.0195796088335704,0.0130068717409757,
-0.00774050347429506));
#54421=CARTESIAN_POINT('Ctrl Pts',(-0.0197520638492665,0.0133014617255382,
-0.00746014347801861));
#54422=CARTESIAN_POINT('Ctrl Pts',(-0.0198383763909096,0.0132421977052975,
-0.00745470174054145));
#54423=CARTESIAN_POINT('Ctrl Pts',(-0.0199284951832807,0.0131884258500566,
-0.00745514727070188));
#54424=CARTESIAN_POINT('Ctrl Pts',(-0.0199259467555682,0.013325645265776,
-0.00733877763912789));
#54425=CARTESIAN_POINT('Ctrl Pts',(-0.0199821693467795,0.0133364139738675,
-0.0073070177250494));
#54426=CARTESIAN_POINT('Ctrl Pts',(-0.0200382272496652,0.0133472837983618,
-0.00727504149123732));
#54427=CARTESIAN_POINT('Ctrl Pts',(-0.0196560990591099,0.0133445491409245,
-0.00747672950133648));
#54428=CARTESIAN_POINT('Ctrl Pts',(-0.0196754866009051,0.0134118597671077,
-0.00738859481309351));
#54429=CARTESIAN_POINT('Ctrl Pts',(-0.0196990588301704,0.0134852524349443,
-0.00730742671988614));
#54430=CARTESIAN_POINT('Origin',(-0.018737818639568,0.0132,-0.0104140389116816));
#54431=CARTESIAN_POINT('Ctrl Pts',(-0.0154071766236069,0.0110829233457151,
-0.0100595855738323));
#54432=CARTESIAN_POINT('Ctrl Pts',(-0.0154721194094679,0.0111605951364923,
-0.0100211957298243));
#54433=CARTESIAN_POINT('Ctrl Pts',(-0.0155420327037426,0.0112386794535643,
-0.00999279989496569));
#54434=CARTESIAN_POINT('Ctrl Pts',(-0.0151569212422682,0.0113984171585124,
-0.0102075198652812));
#54435=CARTESIAN_POINT('Ctrl Pts',(-0.0152241770747978,0.0114088953369853,
-0.0101677627025652));
#54436=CARTESIAN_POINT('Ctrl Pts',(-0.0152926460101778,0.0114192048693264,
-0.0101300478717502));
#54437=CARTESIAN_POINT('Ctrl Pts',(-0.0153264432539109,0.0118064921096535,
-0.0101073097577375));
#54438=CARTESIAN_POINT('Ctrl Pts',(-0.0154009334344641,0.0117391296807366,
-0.0100632761308695));
#54439=CARTESIAN_POINT('Ctrl Pts',(-0.0154795359860423,0.0116713561529081,
-0.0100281788720059));
#54440=CARTESIAN_POINT('Ctrl Pts',(-0.0157884970821157,0.0122415169423427,
-0.00983417434973566));
#54441=CARTESIAN_POINT('Ctrl Pts',(-0.0158707293602409,0.0120936580781721,
-0.00978556411113859));
#54442=CARTESIAN_POINT('Ctrl Pts',(-0.0159658709218911,0.0119472439393342,
-0.00976324159438402));
#54443=CARTESIAN_POINT('Ctrl Pts',(-0.0163381224989415,0.0125871909279286,
-0.00950927245885394));
#54444=CARTESIAN_POINT('Ctrl Pts',(-0.0164265291225076,0.0123754678951022,
-0.00945701235900225));
#54445=CARTESIAN_POINT('Ctrl Pts',(-0.0165379212236351,0.0121682558124033,
-0.00945287823563186));
#54446=CARTESIAN_POINT('Ctrl Pts',(-0.0171083583317725,0.0129643053446502,
-0.00905396040295069));
#54447=CARTESIAN_POINT('Ctrl Pts',(-0.0172023924942094,0.0126795827432054,
-0.00899837367743349));
#54448=CARTESIAN_POINT('Ctrl Pts',(-0.0173348713317463,0.0124060676027306,
-0.00902366736927392));
#54449=CARTESIAN_POINT('Ctrl Pts',(-0.0176718370399433,0.0131859419718071,
-0.00872086937012763));
#54450=CARTESIAN_POINT('Ctrl Pts',(-0.0177670254041465,0.0128543108135448,
-0.00866460035749818));
#54451=CARTESIAN_POINT('Ctrl Pts',(-0.0179151371065852,0.0125415931621198,
-0.00871408984852256));
#54452=CARTESIAN_POINT('Ctrl Pts',(-0.0180036152858858,0.0133040947810426,
-0.00852474419803732));
#54453=CARTESIAN_POINT('Ctrl Pts',(-0.0180979273332784,0.0129456079522531,
-0.00846899320546831));
#54454=CARTESIAN_POINT('Ctrl Pts',(-0.0182549193196156,0.0126114534322405,
-0.00853386516266261));
#54455=CARTESIAN_POINT('Origin',(-0.0162718437026251,0.0114710202288522,
-0.0118595262637278));
#54456=CARTESIAN_POINT('Origin',(-0.0162272231559581,0.00948761256098469,
-0.0118855941465154));
#54457=CARTESIAN_POINT('Origin',(-0.0161828706141249,0.00750421019125213,
-0.0119121602717604));
#54458=CARTESIAN_POINT('Origin',(-0.0161265096054001,0.00500296106758063,
-0.0119313862398486));
#54459=CARTESIAN_POINT('Origin',(-0.0160755784276552,0.00250198330561054,
-0.0119617588041365));
#54460=CARTESIAN_POINT('Origin',(-0.0160741128491222,0.00194984566933334,
-0.0119837251183046));
#54461=CARTESIAN_POINT('Origin',(-0.0160636006313385,0.00139786661560786,
-0.0119901847128056));
#54462=CARTESIAN_POINT('Ctrl Pts',(-0.0168869404495504,0.000131743490843849,
-0.00918484788814817));
#54463=CARTESIAN_POINT('Ctrl Pts',(-0.0169535428340631,0.000396774408641604,
-0.00914547700026949));
#54464=CARTESIAN_POINT('Ctrl Pts',(-0.0170557052878066,0.000651905064219303,
-0.00917195430490026));
#54465=CARTESIAN_POINT('Ctrl Pts',(-0.0166593636290833,0.00020954577683886,
-0.00931937612688517));
#54466=CARTESIAN_POINT('Ctrl Pts',(-0.016726481573608,0.000456067210326956,
-0.0092797004742975));
#54467=CARTESIAN_POINT('Ctrl Pts',(-0.0168241943715066,0.000694725277275201,
-0.00929799565007616));
#54468=CARTESIAN_POINT('Ctrl Pts',(-0.0162745718659412,0.00035276616733443,
-0.0095468393547733));
#54469=CARTESIAN_POINT('Ctrl Pts',(-0.0163418806587457,0.000566569318729898,
-0.00950705088541729));
#54470=CARTESIAN_POINT('Ctrl Pts',(-0.0164319860313115,0.000775586085644678,
-0.00951209192699112));
#54471=CARTESIAN_POINT('Ctrl Pts',(-0.0157435500891547,0.000608559233710922,
-0.0098607440143753));
#54472=CARTESIAN_POINT('Ctrl Pts',(-0.0158093864852093,0.000767682664406866,
-0.00982182592778197));
#54473=CARTESIAN_POINT('Ctrl Pts',(-0.015888931254929,0.000924786987284052,
-0.00980979525072753));
#54474=CARTESIAN_POINT('Ctrl Pts',(-0.0152455191726649,0.000923698582799106,
-0.010155146677592));
#54475=CARTESIAN_POINT('Ctrl Pts',(-0.0153096498691124,0.00101745849940029,
-0.010117236886838));
#54476=CARTESIAN_POINT('Ctrl Pts',(-0.0153787082737323,0.00111153674305079,
-0.0100904302645169));
#54477=CARTESIAN_POINT('Ctrl Pts',(-0.0149409532646179,0.00132777528918322,
-0.01033518573036));
#54478=CARTESIAN_POINT('Ctrl Pts',(-0.0150024908282406,0.00134044710896269,
-0.0102988088268328));
#54479=CARTESIAN_POINT('Ctrl Pts',(-0.0150647545613132,0.00135322574523389,
-0.0102637678926917));
#54480=CARTESIAN_POINT('Ctrl Pts',(-0.0151243477084147,0.00165934770139,
-0.0102267751661056));
#54481=CARTESIAN_POINT('Ctrl Pts',(-0.0151867329811164,0.00160490768149151,
-0.0101898971534335));
#54482=CARTESIAN_POINT('Ctrl Pts',(-0.0152527703332342,0.00155031493930287,
-0.0101599578778916));
#54483=CARTESIAN_POINT('Origin',(-0.0177103885174519,0.000199999999999706,
-0.0110213870786426));
#54484=CARTESIAN_POINT('Ctrl Pts',(-0.018188824141858,8.75761564631602E-5,
-0.00837526872861006));
#54485=CARTESIAN_POINT('Ctrl Pts',(-0.0182113137141289,2.81913691597068E-5,
-0.00831630569299398));
#54486=CARTESIAN_POINT('Ctrl Pts',(-0.018236699754074,-3.41387128105288E-5,
-0.00826219897804721));
#54487=CARTESIAN_POINT('Ctrl Pts',(-0.0183955259428276,0.000103496198700443,
-0.00826521856849081));
#54488=CARTESIAN_POINT('Ctrl Pts',(-0.0184407613226512,9.46547266629223E-5,
-0.00823908285623541));
#54489=CARTESIAN_POINT('Ctrl Pts',(-0.0184860062356923,8.56578675476874E-5,
-0.00821299960804708));
#54490=CARTESIAN_POINT('Ctrl Pts',(-0.0182637622124833,0.000123294745978778,
-0.00835373521604812));
#54491=CARTESIAN_POINT('Ctrl Pts',(-0.0183265003447473,0.000173132371671092,
-0.0083432161596789));
#54492=CARTESIAN_POINT('Ctrl Pts',(-0.0183917093640185,0.000220491112436847,
-0.00833666232475801));
#54493=CARTESIAN_POINT('Ctrl Pts',(-0.0179561164070983,0.000144582042478119,
-0.0085441203472953));
#54494=CARTESIAN_POINT('Ctrl Pts',(-0.0180300450051964,0.000255262336695479,
-0.00853765036489813));
#54495=CARTESIAN_POINT('Ctrl Pts',(-0.0181118555578645,0.000360244421417436,
-0.0085449097825926));
#54496=CARTESIAN_POINT('Ctrl Pts',(-0.0175954738379551,0.000162245221859694,
-0.00876223422164232));
#54497=CARTESIAN_POINT('Ctrl Pts',(-0.0176724428971705,0.000322226944647927,
-0.00875072027092373));
#54498=CARTESIAN_POINT('Ctrl Pts',(-0.0177641850167143,0.000474023149858585,
-0.0087648460645389));
#54499=CARTESIAN_POINT('Ctrl Pts',(-0.0170914446330123,0.000182147225220522,
-0.00906348091051716));
#54500=CARTESIAN_POINT('Ctrl Pts',(-0.0171648487823219,0.000396867148245165,
-0.00903827421404887));
#54501=CARTESIAN_POINT('Ctrl Pts',(-0.0172630627038743,0.000602206025906414,
-0.00905647265972752));
#54502=CARTESIAN_POINT('Ctrl Pts',(-0.0167222986437901,0.000194047757030763,
-0.00928226818221012));
#54503=CARTESIAN_POINT('Ctrl Pts',(-0.0167893016430662,0.000441086163684428,
-0.00924365209871741));
#54504=CARTESIAN_POINT('Ctrl Pts',(-0.0168880399669533,0.000679646241829306,
-0.00926246702800065));
#54505=CARTESIAN_POINT('Ctrl Pts',(-0.0165064972234746,0.000200406501257873,
-0.00940983971047381));
#54506=CARTESIAN_POINT('Ctrl Pts',(-0.0165691023857454,0.000464672578914787,
-0.00936285258941367));
#54507=CARTESIAN_POINT('Ctrl Pts',(-0.01666733255564,0.000721498782670844,
-0.0093817265379391));
#54508=CARTESIAN_POINT('Origin',(-0.0192180740146401,-0.000823943018947793,
-0.00983819116336607));
#54509=CARTESIAN_POINT('Origin',(-0.0183316304034729,0.000200986509768273,
-0.00810139479829735));
#54510=CARTESIAN_POINT('Origin',(-0.00926982557395217,0.0172006855706717,
0.003));
#54511=CARTESIAN_POINT('',(-0.00926982557395217,0.0172006855706717,0.0035));
#54512=CARTESIAN_POINT('Origin',(-0.00926982557395217,0.0172006855706717,
-0.003));
#54513=CARTESIAN_POINT('',(-0.00926982557395217,0.0172006855706717,-0.0025));
#54514=CARTESIAN_POINT('Origin',(0.,0.0254,-0.011));
#54515=CARTESIAN_POINT('',(-6.12323399573677E-20,0.0254,-0.0105));
#54516=CARTESIAN_POINT('Origin',(0.,0.0254,0.011));
#54517=CARTESIAN_POINT('',(-6.12323399573677E-20,0.0254,0.0115));
#54518=CARTESIAN_POINT('Origin',(-0.139,0.0075,0.));
#54519=CARTESIAN_POINT('Origin',(-0.139,0.0075,-0.004));
#54562=UNCERTAINTY_MEASURE_WITH_UNIT(LENGTH_MEASURE(1.E-5),#54581,
'DISTANCE_ACCURACY_VALUE',
'Maximum model space distance between geometric entities at asserted c
onnectivities');
#54564=UNCERTAINTY_MEASURE_WITH_UNIT(LENGTH_MEASURE(1.E-5),#54581,
'DISTANCE_ACCURACY_VALUE',
'Maximum model space distance between geometric entities at asserted c
onnectivities');
#54578=(
GEOMETRIC_REPRESENTATION_CONTEXT(3)
GLOBAL_UNCERTAINTY_ASSIGNED_CONTEXT((#54562))
GLOBAL_UNIT_ASSIGNED_CONTEXT((#54581,#54582,#54583))
REPRESENTATION_CONTEXT('','3D')
);
#54580=(
GEOMETRIC_REPRESENTATION_CONTEXT(3)
GLOBAL_UNCERTAINTY_ASSIGNED_CONTEXT((#54564))
GLOBAL_UNIT_ASSIGNED_CONTEXT((#54581,#54582,#54583))
REPRESENTATION_CONTEXT('','3D')
);
#54581=(
LENGTH_UNIT()
NAMED_UNIT(*)
SI_UNIT($,.METRE.)
);
#54582=(
NAMED_UNIT(*)
PLANE_ANGLE_UNIT()
SI_UNIT($,.RADIAN.)
);
#54583=(
NAMED_UNIT(*)
SI_UNIT($,.STERADIAN.)
SOLID_ANGLE_UNIT()
);
#54597=SHAPE_DEFINITION_REPRESENTATION(#54612,#54642);
#54612=PRODUCT_DEFINITION_SHAPE('',$,#54658);
#54642=SHAPE_REPRESENTATION('',(#19293),#54578);
#54644=PRODUCT_DEFINITION_CONTEXT('part definition',#54691,'design');
#54658=PRODUCT_DEFINITION('Part_9','Part_9',#54673,#54644);
#54673=PRODUCT_DEFINITION_FORMATION('',$,#54706);
#54691=APPLICATION_CONTEXT(
'Core Data for Automotive Mechanical Design Process');
#54692=PRODUCT_CONTEXT('part definition',#54691,'mechanical');
#54706=PRODUCT('Part_9','Part_9','Part 1',(#54692));
#54710=PRESENTATION_STYLE_ASSIGNMENT((#54720));
#54720=SURFACE_STYLE_USAGE(.BOTH.,#54730);
#54730=SURFACE_SIDE_STYLE('',(#54740));
#54740=SURFACE_STYLE_FILL_AREA(#54750);
#54750=FILL_AREA_STYLE('Opaque(170,178,196)',(#54760));
#54760=FILL_AREA_STYLE_COLOUR('Opaque(170,178,196)',#54770);
#54770=COLOUR_RGB('Opaque(170,178,196)', 0.66274510, 0.83137255, 0.94901961);
ENDSEC;
END-ISO-10303-21;
